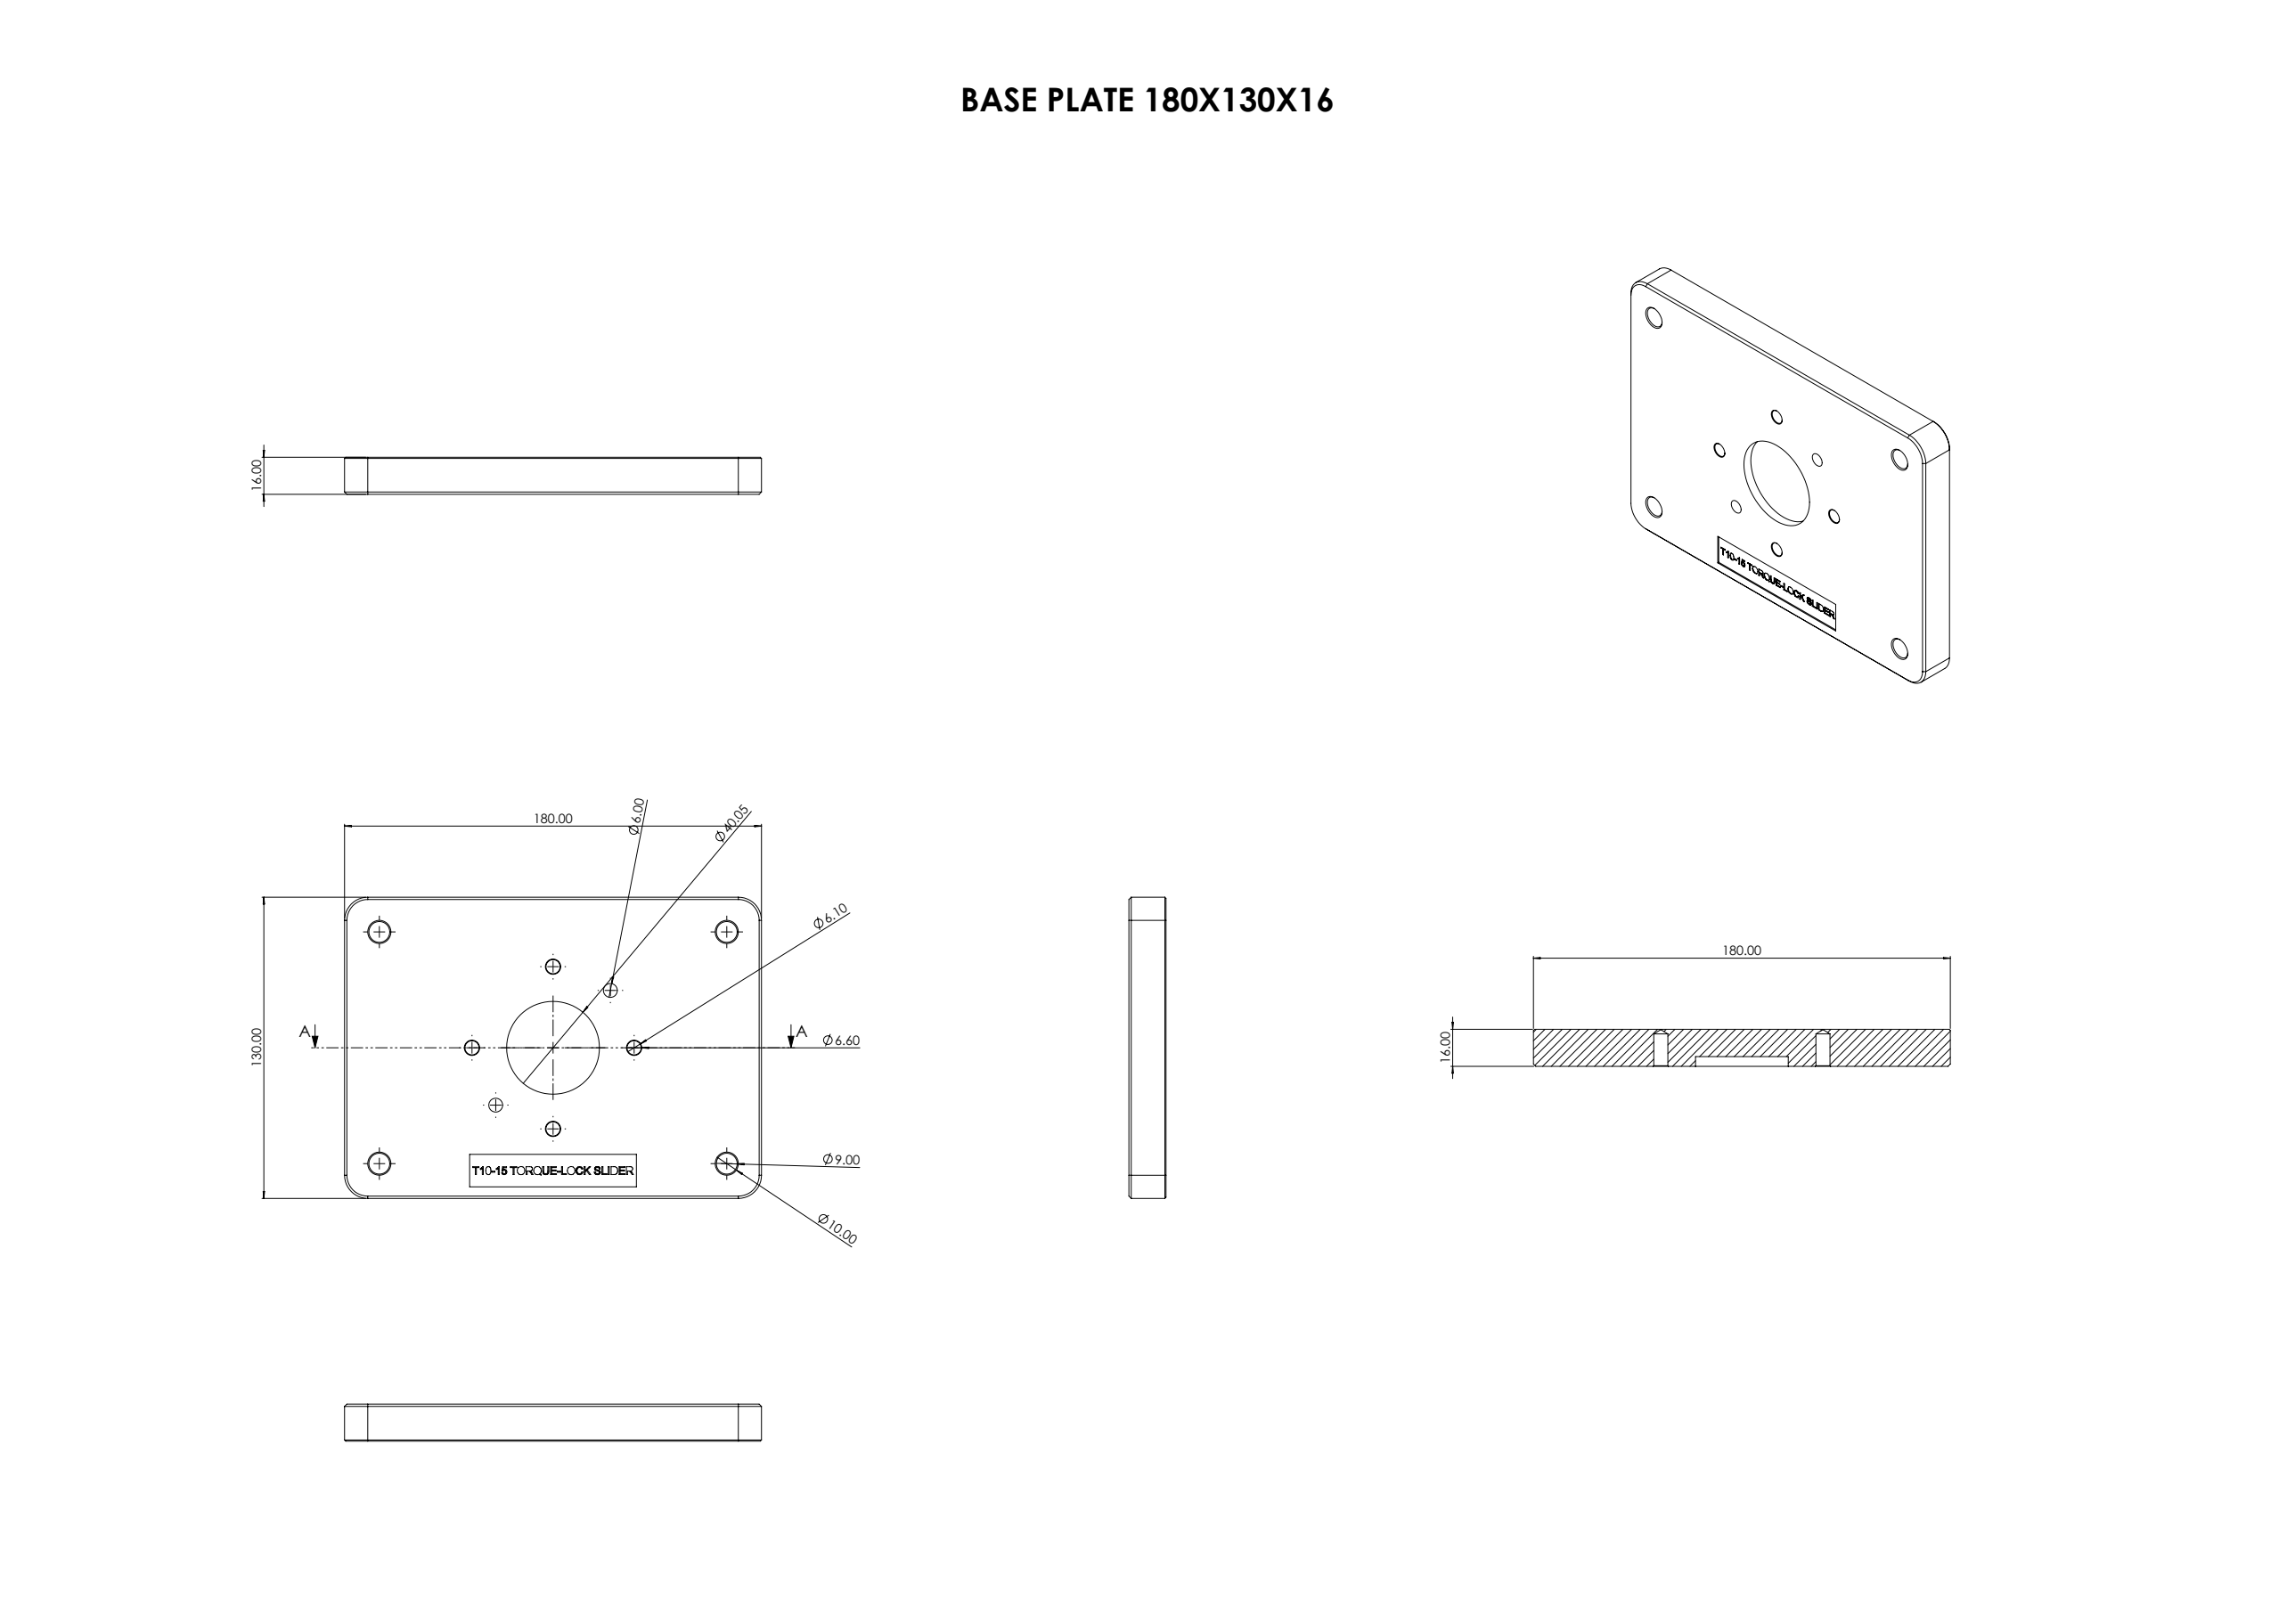
ISO-10303-21;
HEADER;
/* Generated by software containing ST-Developer
 * from STEP Tools, Inc. (www.steptools.com) 
 */

FILE_DESCRIPTION(
/* description */ (''),
/* implementation_level */ '2;1');

FILE_NAME(
/* name */ '04_Base_Plate_180x130x16.step',
/* time_stamp */ '2026-10-11T08:27:52-07:00',
/* author */ (''),
/* organization */ (''),
/* preprocessor_version */ 'ST-DEVELOPER v20.2',
/* originating_system */ 'Autodesk Translation Framework v15.15.0.0',
/* authorisation */ '');

FILE_SCHEMA (('AUTOMOTIVE_DESIGN { 1 0 10303 214 3 1 1 }'));
ENDSEC;

DATA;
#10=MECHANICAL_DESIGN_GEOMETRIC_PRESENTATION_REPRESENTATION('',(#922),#94301);
#147=B_SPLINE_CURVE_WITH_KNOTS('',2,(#80633,#80634,#80635),
 .UNSPECIFIED.,.F.,.F.,(3,3),(0.,1.),.UNSPECIFIED.);
#148=B_SPLINE_CURVE_WITH_KNOTS('',2,(#80639,#80640,#80641),
 .UNSPECIFIED.,.F.,.F.,(3,3),(0.,1.),.UNSPECIFIED.);
#149=B_SPLINE_CURVE_WITH_KNOTS('',2,(#80650,#80651,#80652),
 .UNSPECIFIED.,.F.,.F.,(3,3),(0.,1.),.UNSPECIFIED.);
#150=B_SPLINE_CURVE_WITH_KNOTS('',2,(#80655,#80656,#80657),
 .UNSPECIFIED.,.F.,.F.,(3,3),(0.,1.),.UNSPECIFIED.);
#151=B_SPLINE_CURVE_WITH_KNOTS('',2,(#80665,#80666,#80667),
 .UNSPECIFIED.,.F.,.F.,(3,3),(0.,1.),.UNSPECIFIED.);
#152=B_SPLINE_CURVE_WITH_KNOTS('',2,(#80670,#80671,#80672),
 .UNSPECIFIED.,.F.,.F.,(3,3),(0.,1.),.UNSPECIFIED.);
#153=B_SPLINE_CURVE_WITH_KNOTS('',2,(#80680,#80681,#80682),
 .UNSPECIFIED.,.F.,.F.,(3,3),(0.,1.),.UNSPECIFIED.);
#154=B_SPLINE_CURVE_WITH_KNOTS('',2,(#80685,#80686,#80687),
 .UNSPECIFIED.,.F.,.F.,(3,3),(0.,1.),.UNSPECIFIED.);
#155=B_SPLINE_CURVE_WITH_KNOTS('',2,(#80695,#80696,#80697),
 .UNSPECIFIED.,.F.,.F.,(3,3),(0.,1.),.UNSPECIFIED.);
#156=B_SPLINE_CURVE_WITH_KNOTS('',2,(#80700,#80701,#80702),
 .UNSPECIFIED.,.F.,.F.,(3,3),(0.,1.),.UNSPECIFIED.);
#157=B_SPLINE_CURVE_WITH_KNOTS('',2,(#80710,#80711,#80712),
 .UNSPECIFIED.,.F.,.F.,(3,3),(0.,1.),.UNSPECIFIED.);
#158=B_SPLINE_CURVE_WITH_KNOTS('',2,(#80715,#80716,#80717),
 .UNSPECIFIED.,.F.,.F.,(3,3),(0.,1.),.UNSPECIFIED.);
#159=B_SPLINE_CURVE_WITH_KNOTS('',2,(#80725,#80726,#80727),
 .UNSPECIFIED.,.F.,.F.,(3,3),(0.,1.),.UNSPECIFIED.);
#160=B_SPLINE_CURVE_WITH_KNOTS('',2,(#80730,#80731,#80732),
 .UNSPECIFIED.,.F.,.F.,(3,3),(0.,1.),.UNSPECIFIED.);
#161=B_SPLINE_CURVE_WITH_KNOTS('',2,(#80740,#80741,#80742),
 .UNSPECIFIED.,.F.,.F.,(3,3),(0.,1.),.UNSPECIFIED.);
#162=B_SPLINE_CURVE_WITH_KNOTS('',2,(#80745,#80746,#80747),
 .UNSPECIFIED.,.F.,.F.,(3,3),(0.,1.),.UNSPECIFIED.);
#163=B_SPLINE_CURVE_WITH_KNOTS('',2,(#80755,#80756,#80757),
 .UNSPECIFIED.,.F.,.F.,(3,3),(0.,1.),.UNSPECIFIED.);
#164=B_SPLINE_CURVE_WITH_KNOTS('',2,(#80760,#80761,#80762),
 .UNSPECIFIED.,.F.,.F.,(3,3),(0.,1.),.UNSPECIFIED.);
#165=B_SPLINE_CURVE_WITH_KNOTS('',2,(#80770,#80771,#80772),
 .UNSPECIFIED.,.F.,.F.,(3,3),(0.,1.),.UNSPECIFIED.);
#166=B_SPLINE_CURVE_WITH_KNOTS('',2,(#80775,#80776,#80777),
 .UNSPECIFIED.,.F.,.F.,(3,3),(0.,1.),.UNSPECIFIED.);
#167=B_SPLINE_CURVE_WITH_KNOTS('',2,(#80785,#80786,#80787),
 .UNSPECIFIED.,.F.,.F.,(3,3),(0.,1.),.UNSPECIFIED.);
#168=B_SPLINE_CURVE_WITH_KNOTS('',2,(#80790,#80791,#80792),
 .UNSPECIFIED.,.F.,.F.,(3,3),(0.,1.),.UNSPECIFIED.);
#169=B_SPLINE_CURVE_WITH_KNOTS('',2,(#80800,#80801,#80802),
 .UNSPECIFIED.,.F.,.F.,(3,3),(0.,1.),.UNSPECIFIED.);
#170=B_SPLINE_CURVE_WITH_KNOTS('',2,(#80805,#80806,#80807),
 .UNSPECIFIED.,.F.,.F.,(3,3),(0.,1.),.UNSPECIFIED.);
#171=B_SPLINE_CURVE_WITH_KNOTS('',2,(#80815,#80816,#80817),
 .UNSPECIFIED.,.F.,.F.,(3,3),(0.,1.),.UNSPECIFIED.);
#172=B_SPLINE_CURVE_WITH_KNOTS('',2,(#80820,#80821,#80822),
 .UNSPECIFIED.,.F.,.F.,(3,3),(0.,1.),.UNSPECIFIED.);
#173=B_SPLINE_CURVE_WITH_KNOTS('',2,(#80836,#80837,#80838),
 .UNSPECIFIED.,.F.,.F.,(3,3),(0.,1.),.UNSPECIFIED.);
#174=B_SPLINE_CURVE_WITH_KNOTS('',2,(#80841,#80842,#80843),
 .UNSPECIFIED.,.F.,.F.,(3,3),(0.,1.),.UNSPECIFIED.);
#175=B_SPLINE_CURVE_WITH_KNOTS('',2,(#80851,#80852,#80853),
 .UNSPECIFIED.,.F.,.F.,(3,3),(0.,1.),.UNSPECIFIED.);
#176=B_SPLINE_CURVE_WITH_KNOTS('',2,(#80856,#80857,#80858),
 .UNSPECIFIED.,.F.,.F.,(3,3),(0.,1.),.UNSPECIFIED.);
#177=B_SPLINE_CURVE_WITH_KNOTS('',2,(#80866,#80867,#80868),
 .UNSPECIFIED.,.F.,.F.,(3,3),(0.,1.),.UNSPECIFIED.);
#178=B_SPLINE_CURVE_WITH_KNOTS('',2,(#80871,#80872,#80873),
 .UNSPECIFIED.,.F.,.F.,(3,3),(0.,1.),.UNSPECIFIED.);
#179=B_SPLINE_CURVE_WITH_KNOTS('',2,(#80881,#80882,#80883),
 .UNSPECIFIED.,.F.,.F.,(3,3),(0.,1.),.UNSPECIFIED.);
#180=B_SPLINE_CURVE_WITH_KNOTS('',2,(#80886,#80887,#80888),
 .UNSPECIFIED.,.F.,.F.,(3,3),(0.,1.),.UNSPECIFIED.);
#181=B_SPLINE_CURVE_WITH_KNOTS('',2,(#80896,#80897,#80898),
 .UNSPECIFIED.,.F.,.F.,(3,3),(0.,1.),.UNSPECIFIED.);
#182=B_SPLINE_CURVE_WITH_KNOTS('',2,(#80901,#80902,#80903),
 .UNSPECIFIED.,.F.,.F.,(3,3),(0.,1.),.UNSPECIFIED.);
#183=B_SPLINE_CURVE_WITH_KNOTS('',2,(#80911,#80912,#80913),
 .UNSPECIFIED.,.F.,.F.,(3,3),(0.,1.),.UNSPECIFIED.);
#184=B_SPLINE_CURVE_WITH_KNOTS('',2,(#80916,#80917,#80918),
 .UNSPECIFIED.,.F.,.F.,(3,3),(0.,1.),.UNSPECIFIED.);
#185=B_SPLINE_CURVE_WITH_KNOTS('',2,(#80926,#80927,#80928),
 .UNSPECIFIED.,.F.,.F.,(3,3),(0.,1.),.UNSPECIFIED.);
#186=B_SPLINE_CURVE_WITH_KNOTS('',2,(#80931,#80932,#80933),
 .UNSPECIFIED.,.F.,.F.,(3,3),(0.,1.),.UNSPECIFIED.);
#187=B_SPLINE_CURVE_WITH_KNOTS('',2,(#80941,#80942,#80943),
 .UNSPECIFIED.,.F.,.F.,(3,3),(0.,1.),.UNSPECIFIED.);
#188=B_SPLINE_CURVE_WITH_KNOTS('',2,(#80946,#80947,#80948),
 .UNSPECIFIED.,.F.,.F.,(3,3),(0.,1.),.UNSPECIFIED.);
#189=B_SPLINE_CURVE_WITH_KNOTS('',2,(#80956,#80957,#80958),
 .UNSPECIFIED.,.F.,.F.,(3,3),(0.,1.),.UNSPECIFIED.);
#190=B_SPLINE_CURVE_WITH_KNOTS('',2,(#80961,#80962,#80963),
 .UNSPECIFIED.,.F.,.F.,(3,3),(0.,1.),.UNSPECIFIED.);
#191=B_SPLINE_CURVE_WITH_KNOTS('',2,(#80971,#80972,#80973),
 .UNSPECIFIED.,.F.,.F.,(3,3),(0.,1.),.UNSPECIFIED.);
#192=B_SPLINE_CURVE_WITH_KNOTS('',2,(#80976,#80977,#80978),
 .UNSPECIFIED.,.F.,.F.,(3,3),(0.,1.),.UNSPECIFIED.);
#193=B_SPLINE_CURVE_WITH_KNOTS('',2,(#80986,#80987,#80988),
 .UNSPECIFIED.,.F.,.F.,(3,3),(0.,1.),.UNSPECIFIED.);
#194=B_SPLINE_CURVE_WITH_KNOTS('',2,(#80991,#80992,#80993),
 .UNSPECIFIED.,.F.,.F.,(3,3),(0.,1.),.UNSPECIFIED.);
#195=B_SPLINE_CURVE_WITH_KNOTS('',2,(#81001,#81002,#81003),
 .UNSPECIFIED.,.F.,.F.,(3,3),(0.,1.),.UNSPECIFIED.);
#196=B_SPLINE_CURVE_WITH_KNOTS('',2,(#81006,#81007,#81008),
 .UNSPECIFIED.,.F.,.F.,(3,3),(0.,1.),.UNSPECIFIED.);
#197=B_SPLINE_CURVE_WITH_KNOTS('',2,(#81016,#81017,#81018),
 .UNSPECIFIED.,.F.,.F.,(3,3),(0.,1.),.UNSPECIFIED.);
#198=B_SPLINE_CURVE_WITH_KNOTS('',2,(#81021,#81022,#81023),
 .UNSPECIFIED.,.F.,.F.,(3,3),(0.,1.),.UNSPECIFIED.);
#199=B_SPLINE_CURVE_WITH_KNOTS('',2,(#81031,#81032,#81033),
 .UNSPECIFIED.,.F.,.F.,(3,3),(0.,1.),.UNSPECIFIED.);
#200=B_SPLINE_CURVE_WITH_KNOTS('',2,(#81036,#81037,#81038),
 .UNSPECIFIED.,.F.,.F.,(3,3),(0.,1.),.UNSPECIFIED.);
#201=B_SPLINE_CURVE_WITH_KNOTS('',2,(#81046,#81047,#81048),
 .UNSPECIFIED.,.F.,.F.,(3,3),(0.,1.),.UNSPECIFIED.);
#202=B_SPLINE_CURVE_WITH_KNOTS('',2,(#81051,#81052,#81053),
 .UNSPECIFIED.,.F.,.F.,(3,3),(0.,1.),.UNSPECIFIED.);
#203=B_SPLINE_CURVE_WITH_KNOTS('',2,(#81061,#81062,#81063),
 .UNSPECIFIED.,.F.,.F.,(3,3),(0.,1.),.UNSPECIFIED.);
#204=B_SPLINE_CURVE_WITH_KNOTS('',2,(#81066,#81067,#81068),
 .UNSPECIFIED.,.F.,.F.,(3,3),(0.,1.),.UNSPECIFIED.);
#205=B_SPLINE_CURVE_WITH_KNOTS('',2,(#81076,#81077,#81078),
 .UNSPECIFIED.,.F.,.F.,(3,3),(0.,1.),.UNSPECIFIED.);
#206=B_SPLINE_CURVE_WITH_KNOTS('',2,(#81081,#81082,#81083),
 .UNSPECIFIED.,.F.,.F.,(3,3),(0.,1.),.UNSPECIFIED.);
#207=B_SPLINE_CURVE_WITH_KNOTS('',2,(#81091,#81092,#81093),
 .UNSPECIFIED.,.F.,.F.,(3,3),(0.,1.),.UNSPECIFIED.);
#208=B_SPLINE_CURVE_WITH_KNOTS('',2,(#81096,#81097,#81098),
 .UNSPECIFIED.,.F.,.F.,(3,3),(0.,1.),.UNSPECIFIED.);
#209=B_SPLINE_CURVE_WITH_KNOTS('',2,(#81112,#81113,#81114),
 .UNSPECIFIED.,.F.,.F.,(3,3),(0.,1.),.UNSPECIFIED.);
#210=B_SPLINE_CURVE_WITH_KNOTS('',2,(#81117,#81118,#81119),
 .UNSPECIFIED.,.F.,.F.,(3,3),(0.,1.),.UNSPECIFIED.);
#211=B_SPLINE_CURVE_WITH_KNOTS('',2,(#81126,#81127,#81128),
 .UNSPECIFIED.,.F.,.F.,(3,3),(0.,1.),.UNSPECIFIED.);
#212=B_SPLINE_CURVE_WITH_KNOTS('',2,(#81129,#81130,#81131),
 .UNSPECIFIED.,.F.,.F.,(3,3),(0.,1.),.UNSPECIFIED.);
#213=B_SPLINE_CURVE_WITH_KNOTS('',2,(#81141,#81142,#81143),
 .UNSPECIFIED.,.F.,.F.,(3,3),(0.,1.),.UNSPECIFIED.);
#214=B_SPLINE_CURVE_WITH_KNOTS('',2,(#81147,#81148,#81149),
 .UNSPECIFIED.,.F.,.F.,(3,3),(0.,1.),.UNSPECIFIED.);
#215=B_SPLINE_CURVE_WITH_KNOTS('',2,(#81158,#81159,#81160),
 .UNSPECIFIED.,.F.,.F.,(3,3),(0.,1.),.UNSPECIFIED.);
#216=B_SPLINE_CURVE_WITH_KNOTS('',2,(#81163,#81164,#81165),
 .UNSPECIFIED.,.F.,.F.,(3,3),(0.,1.),.UNSPECIFIED.);
#217=B_SPLINE_CURVE_WITH_KNOTS('',2,(#81173,#81174,#81175),
 .UNSPECIFIED.,.F.,.F.,(3,3),(0.,1.),.UNSPECIFIED.);
#218=B_SPLINE_CURVE_WITH_KNOTS('',2,(#81178,#81179,#81180),
 .UNSPECIFIED.,.F.,.F.,(3,3),(0.,1.),.UNSPECIFIED.);
#219=B_SPLINE_CURVE_WITH_KNOTS('',2,(#81188,#81189,#81190),
 .UNSPECIFIED.,.F.,.F.,(3,3),(0.,1.),.UNSPECIFIED.);
#220=B_SPLINE_CURVE_WITH_KNOTS('',2,(#81193,#81194,#81195),
 .UNSPECIFIED.,.F.,.F.,(3,3),(0.,1.),.UNSPECIFIED.);
#221=B_SPLINE_CURVE_WITH_KNOTS('',2,(#81203,#81204,#81205),
 .UNSPECIFIED.,.F.,.F.,(3,3),(0.,1.),.UNSPECIFIED.);
#222=B_SPLINE_CURVE_WITH_KNOTS('',2,(#81208,#81209,#81210),
 .UNSPECIFIED.,.F.,.F.,(3,3),(0.,1.),.UNSPECIFIED.);
#223=B_SPLINE_CURVE_WITH_KNOTS('',2,(#81218,#81219,#81220),
 .UNSPECIFIED.,.F.,.F.,(3,3),(0.,1.),.UNSPECIFIED.);
#224=B_SPLINE_CURVE_WITH_KNOTS('',2,(#81223,#81224,#81225),
 .UNSPECIFIED.,.F.,.F.,(3,3),(0.,1.),.UNSPECIFIED.);
#225=B_SPLINE_CURVE_WITH_KNOTS('',2,(#81233,#81234,#81235),
 .UNSPECIFIED.,.F.,.F.,(3,3),(0.,1.),.UNSPECIFIED.);
#226=B_SPLINE_CURVE_WITH_KNOTS('',2,(#81238,#81239,#81240),
 .UNSPECIFIED.,.F.,.F.,(3,3),(0.,1.),.UNSPECIFIED.);
#227=B_SPLINE_CURVE_WITH_KNOTS('',2,(#81248,#81249,#81250),
 .UNSPECIFIED.,.F.,.F.,(3,3),(0.,1.),.UNSPECIFIED.);
#228=B_SPLINE_CURVE_WITH_KNOTS('',2,(#81253,#81254,#81255),
 .UNSPECIFIED.,.F.,.F.,(3,3),(0.,1.),.UNSPECIFIED.);
#229=B_SPLINE_CURVE_WITH_KNOTS('',2,(#81269,#81270,#81271),
 .UNSPECIFIED.,.F.,.F.,(3,3),(0.,1.),.UNSPECIFIED.);
#230=B_SPLINE_CURVE_WITH_KNOTS('',2,(#81274,#81275,#81276),
 .UNSPECIFIED.,.F.,.F.,(3,3),(0.,1.),.UNSPECIFIED.);
#231=B_SPLINE_CURVE_WITH_KNOTS('',2,(#81284,#81285,#81286),
 .UNSPECIFIED.,.F.,.F.,(3,3),(0.,1.),.UNSPECIFIED.);
#232=B_SPLINE_CURVE_WITH_KNOTS('',2,(#81289,#81290,#81291),
 .UNSPECIFIED.,.F.,.F.,(3,3),(0.,1.),.UNSPECIFIED.);
#233=B_SPLINE_CURVE_WITH_KNOTS('',2,(#81299,#81300,#81301),
 .UNSPECIFIED.,.F.,.F.,(3,3),(0.,1.),.UNSPECIFIED.);
#234=B_SPLINE_CURVE_WITH_KNOTS('',2,(#81304,#81305,#81306),
 .UNSPECIFIED.,.F.,.F.,(3,3),(0.,1.),.UNSPECIFIED.);
#235=B_SPLINE_CURVE_WITH_KNOTS('',2,(#81314,#81315,#81316),
 .UNSPECIFIED.,.F.,.F.,(3,3),(0.,1.),.UNSPECIFIED.);
#236=B_SPLINE_CURVE_WITH_KNOTS('',2,(#81319,#81320,#81321),
 .UNSPECIFIED.,.F.,.F.,(3,3),(0.,1.),.UNSPECIFIED.);
#237=B_SPLINE_CURVE_WITH_KNOTS('',2,(#81329,#81330,#81331),
 .UNSPECIFIED.,.F.,.F.,(3,3),(0.,1.),.UNSPECIFIED.);
#238=B_SPLINE_CURVE_WITH_KNOTS('',2,(#81334,#81335,#81336),
 .UNSPECIFIED.,.F.,.F.,(3,3),(0.,1.),.UNSPECIFIED.);
#239=B_SPLINE_CURVE_WITH_KNOTS('',2,(#81344,#81345,#81346),
 .UNSPECIFIED.,.F.,.F.,(3,3),(0.,1.),.UNSPECIFIED.);
#240=B_SPLINE_CURVE_WITH_KNOTS('',2,(#81349,#81350,#81351),
 .UNSPECIFIED.,.F.,.F.,(3,3),(0.,1.),.UNSPECIFIED.);
#241=B_SPLINE_CURVE_WITH_KNOTS('',2,(#81359,#81360,#81361),
 .UNSPECIFIED.,.F.,.F.,(3,3),(0.,1.),.UNSPECIFIED.);
#242=B_SPLINE_CURVE_WITH_KNOTS('',2,(#81364,#81365,#81366),
 .UNSPECIFIED.,.F.,.F.,(3,3),(0.,1.),.UNSPECIFIED.);
#243=B_SPLINE_CURVE_WITH_KNOTS('',2,(#81374,#81375,#81376),
 .UNSPECIFIED.,.F.,.F.,(3,3),(0.,1.),.UNSPECIFIED.);
#244=B_SPLINE_CURVE_WITH_KNOTS('',2,(#81379,#81380,#81381),
 .UNSPECIFIED.,.F.,.F.,(3,3),(0.,1.),.UNSPECIFIED.);
#245=B_SPLINE_CURVE_WITH_KNOTS('',2,(#81389,#81390,#81391),
 .UNSPECIFIED.,.F.,.F.,(3,3),(0.,1.),.UNSPECIFIED.);
#246=B_SPLINE_CURVE_WITH_KNOTS('',2,(#81394,#81395,#81396),
 .UNSPECIFIED.,.F.,.F.,(3,3),(0.,1.),.UNSPECIFIED.);
#247=B_SPLINE_CURVE_WITH_KNOTS('',2,(#81404,#81405,#81406),
 .UNSPECIFIED.,.F.,.F.,(3,3),(0.,1.),.UNSPECIFIED.);
#248=B_SPLINE_CURVE_WITH_KNOTS('',2,(#81409,#81410,#81411),
 .UNSPECIFIED.,.F.,.F.,(3,3),(0.,1.),.UNSPECIFIED.);
#249=B_SPLINE_CURVE_WITH_KNOTS('',2,(#81425,#81426,#81427),
 .UNSPECIFIED.,.F.,.F.,(3,3),(0.,1.),.UNSPECIFIED.);
#250=B_SPLINE_CURVE_WITH_KNOTS('',2,(#81430,#81431,#81432),
 .UNSPECIFIED.,.F.,.F.,(3,3),(0.,1.),.UNSPECIFIED.);
#251=B_SPLINE_CURVE_WITH_KNOTS('',2,(#81439,#81440,#81441),
 .UNSPECIFIED.,.F.,.F.,(3,3),(0.,1.),.UNSPECIFIED.);
#252=B_SPLINE_CURVE_WITH_KNOTS('',2,(#81442,#81443,#81444),
 .UNSPECIFIED.,.F.,.F.,(3,3),(0.,1.),.UNSPECIFIED.);
#253=B_SPLINE_CURVE_WITH_KNOTS('',2,(#81540,#81541,#81542),
 .UNSPECIFIED.,.F.,.F.,(3,3),(0.,1.),.UNSPECIFIED.);
#254=B_SPLINE_CURVE_WITH_KNOTS('',2,(#81546,#81547,#81548),
 .UNSPECIFIED.,.F.,.F.,(3,3),(0.,1.),.UNSPECIFIED.);
#255=B_SPLINE_CURVE_WITH_KNOTS('',2,(#81557,#81558,#81559),
 .UNSPECIFIED.,.F.,.F.,(3,3),(0.,1.),.UNSPECIFIED.);
#256=B_SPLINE_CURVE_WITH_KNOTS('',2,(#81562,#81563,#81564),
 .UNSPECIFIED.,.F.,.F.,(3,3),(0.,1.),.UNSPECIFIED.);
#257=B_SPLINE_CURVE_WITH_KNOTS('',2,(#81572,#81573,#81574),
 .UNSPECIFIED.,.F.,.F.,(3,3),(0.,1.),.UNSPECIFIED.);
#258=B_SPLINE_CURVE_WITH_KNOTS('',2,(#81577,#81578,#81579),
 .UNSPECIFIED.,.F.,.F.,(3,3),(0.,1.),.UNSPECIFIED.);
#259=B_SPLINE_CURVE_WITH_KNOTS('',2,(#81587,#81588,#81589),
 .UNSPECIFIED.,.F.,.F.,(3,3),(0.,1.),.UNSPECIFIED.);
#260=B_SPLINE_CURVE_WITH_KNOTS('',2,(#81592,#81593,#81594),
 .UNSPECIFIED.,.F.,.F.,(3,3),(0.,1.),.UNSPECIFIED.);
#261=B_SPLINE_CURVE_WITH_KNOTS('',2,(#81620,#81621,#81622),
 .UNSPECIFIED.,.F.,.F.,(3,3),(0.,1.),.UNSPECIFIED.);
#262=B_SPLINE_CURVE_WITH_KNOTS('',2,(#81625,#81626,#81627),
 .UNSPECIFIED.,.F.,.F.,(3,3),(0.,1.),.UNSPECIFIED.);
#263=B_SPLINE_CURVE_WITH_KNOTS('',2,(#81635,#81636,#81637),
 .UNSPECIFIED.,.F.,.F.,(3,3),(0.,1.),.UNSPECIFIED.);
#264=B_SPLINE_CURVE_WITH_KNOTS('',2,(#81640,#81641,#81642),
 .UNSPECIFIED.,.F.,.F.,(3,3),(0.,1.),.UNSPECIFIED.);
#265=B_SPLINE_CURVE_WITH_KNOTS('',2,(#81650,#81651,#81652),
 .UNSPECIFIED.,.F.,.F.,(3,3),(0.,1.),.UNSPECIFIED.);
#266=B_SPLINE_CURVE_WITH_KNOTS('',2,(#81655,#81656,#81657),
 .UNSPECIFIED.,.F.,.F.,(3,3),(0.,1.),.UNSPECIFIED.);
#267=B_SPLINE_CURVE_WITH_KNOTS('',2,(#81665,#81666,#81667),
 .UNSPECIFIED.,.F.,.F.,(3,3),(0.,1.),.UNSPECIFIED.);
#268=B_SPLINE_CURVE_WITH_KNOTS('',2,(#81670,#81671,#81672),
 .UNSPECIFIED.,.F.,.F.,(3,3),(0.,1.),.UNSPECIFIED.);
#269=B_SPLINE_CURVE_WITH_KNOTS('',2,(#81680,#81681,#81682),
 .UNSPECIFIED.,.F.,.F.,(3,3),(0.,1.),.UNSPECIFIED.);
#270=B_SPLINE_CURVE_WITH_KNOTS('',2,(#81685,#81686,#81687),
 .UNSPECIFIED.,.F.,.F.,(3,3),(0.,1.),.UNSPECIFIED.);
#271=B_SPLINE_CURVE_WITH_KNOTS('',2,(#81695,#81696,#81697),
 .UNSPECIFIED.,.F.,.F.,(3,3),(0.,1.),.UNSPECIFIED.);
#272=B_SPLINE_CURVE_WITH_KNOTS('',2,(#81700,#81701,#81702),
 .UNSPECIFIED.,.F.,.F.,(3,3),(0.,1.),.UNSPECIFIED.);
#273=B_SPLINE_CURVE_WITH_KNOTS('',2,(#81727,#81728,#81729),
 .UNSPECIFIED.,.F.,.F.,(3,3),(0.,1.),.UNSPECIFIED.);
#274=B_SPLINE_CURVE_WITH_KNOTS('',2,(#81730,#81731,#81732),
 .UNSPECIFIED.,.F.,.F.,(3,3),(0.,1.),.UNSPECIFIED.);
#275=B_SPLINE_CURVE_WITH_KNOTS('',2,(#81750,#81751,#81752),
 .UNSPECIFIED.,.F.,.F.,(3,3),(0.,1.),.UNSPECIFIED.);
#276=B_SPLINE_CURVE_WITH_KNOTS('',2,(#81755,#81756,#81757),
 .UNSPECIFIED.,.F.,.F.,(3,3),(0.,1.),.UNSPECIFIED.);
#277=B_SPLINE_CURVE_WITH_KNOTS('',2,(#81765,#81766,#81767),
 .UNSPECIFIED.,.F.,.F.,(3,3),(0.,1.),.UNSPECIFIED.);
#278=B_SPLINE_CURVE_WITH_KNOTS('',2,(#81770,#81771,#81772),
 .UNSPECIFIED.,.F.,.F.,(3,3),(0.,1.),.UNSPECIFIED.);
#279=B_SPLINE_CURVE_WITH_KNOTS('',2,(#81780,#81781,#81782),
 .UNSPECIFIED.,.F.,.F.,(3,3),(0.,1.),.UNSPECIFIED.);
#280=B_SPLINE_CURVE_WITH_KNOTS('',2,(#81785,#81786,#81787),
 .UNSPECIFIED.,.F.,.F.,(3,3),(0.,1.),.UNSPECIFIED.);
#281=B_SPLINE_CURVE_WITH_KNOTS('',2,(#81795,#81796,#81797),
 .UNSPECIFIED.,.F.,.F.,(3,3),(0.,1.),.UNSPECIFIED.);
#282=B_SPLINE_CURVE_WITH_KNOTS('',2,(#81800,#81801,#81802),
 .UNSPECIFIED.,.F.,.F.,(3,3),(0.,1.),.UNSPECIFIED.);
#283=B_SPLINE_CURVE_WITH_KNOTS('',2,(#81828,#81829,#81830),
 .UNSPECIFIED.,.F.,.F.,(3,3),(0.,1.),.UNSPECIFIED.);
#284=B_SPLINE_CURVE_WITH_KNOTS('',2,(#81833,#81834,#81835),
 .UNSPECIFIED.,.F.,.F.,(3,3),(0.,1.),.UNSPECIFIED.);
#285=B_SPLINE_CURVE_WITH_KNOTS('',2,(#81843,#81844,#81845),
 .UNSPECIFIED.,.F.,.F.,(3,3),(0.,1.),.UNSPECIFIED.);
#286=B_SPLINE_CURVE_WITH_KNOTS('',2,(#81848,#81849,#81850),
 .UNSPECIFIED.,.F.,.F.,(3,3),(0.,1.),.UNSPECIFIED.);
#287=B_SPLINE_CURVE_WITH_KNOTS('',2,(#81858,#81859,#81860),
 .UNSPECIFIED.,.F.,.F.,(3,3),(0.,1.),.UNSPECIFIED.);
#288=B_SPLINE_CURVE_WITH_KNOTS('',2,(#81863,#81864,#81865),
 .UNSPECIFIED.,.F.,.F.,(3,3),(0.,1.),.UNSPECIFIED.);
#289=B_SPLINE_CURVE_WITH_KNOTS('',2,(#81873,#81874,#81875),
 .UNSPECIFIED.,.F.,.F.,(3,3),(0.,1.),.UNSPECIFIED.);
#290=B_SPLINE_CURVE_WITH_KNOTS('',2,(#81878,#81879,#81880),
 .UNSPECIFIED.,.F.,.F.,(3,3),(0.,1.),.UNSPECIFIED.);
#291=B_SPLINE_CURVE_WITH_KNOTS('',2,(#81888,#81889,#81890),
 .UNSPECIFIED.,.F.,.F.,(3,3),(0.,1.),.UNSPECIFIED.);
#292=B_SPLINE_CURVE_WITH_KNOTS('',2,(#81893,#81894,#81895),
 .UNSPECIFIED.,.F.,.F.,(3,3),(0.,1.),.UNSPECIFIED.);
#293=B_SPLINE_CURVE_WITH_KNOTS('',2,(#81903,#81904,#81905),
 .UNSPECIFIED.,.F.,.F.,(3,3),(0.,1.),.UNSPECIFIED.);
#294=B_SPLINE_CURVE_WITH_KNOTS('',2,(#81908,#81909,#81910),
 .UNSPECIFIED.,.F.,.F.,(3,3),(0.,1.),.UNSPECIFIED.);
#295=B_SPLINE_CURVE_WITH_KNOTS('',2,(#81918,#81919,#81920),
 .UNSPECIFIED.,.F.,.F.,(3,3),(0.,1.),.UNSPECIFIED.);
#296=B_SPLINE_CURVE_WITH_KNOTS('',2,(#81923,#81924,#81925),
 .UNSPECIFIED.,.F.,.F.,(3,3),(0.,1.),.UNSPECIFIED.);
#297=B_SPLINE_CURVE_WITH_KNOTS('',2,(#82005,#82006,#82007),
 .UNSPECIFIED.,.F.,.F.,(3,3),(0.,1.),.UNSPECIFIED.);
#298=B_SPLINE_CURVE_WITH_KNOTS('',2,(#82011,#82012,#82013),
 .UNSPECIFIED.,.F.,.F.,(3,3),(0.,1.),.UNSPECIFIED.);
#299=B_SPLINE_CURVE_WITH_KNOTS('',2,(#82022,#82023,#82024),
 .UNSPECIFIED.,.F.,.F.,(3,3),(0.,1.),.UNSPECIFIED.);
#300=B_SPLINE_CURVE_WITH_KNOTS('',2,(#82027,#82028,#82029),
 .UNSPECIFIED.,.F.,.F.,(3,3),(0.,1.),.UNSPECIFIED.);
#301=B_SPLINE_CURVE_WITH_KNOTS('',2,(#82043,#82044,#82045),
 .UNSPECIFIED.,.F.,.F.,(3,3),(0.,1.),.UNSPECIFIED.);
#302=B_SPLINE_CURVE_WITH_KNOTS('',2,(#82048,#82049,#82050),
 .UNSPECIFIED.,.F.,.F.,(3,3),(0.,1.),.UNSPECIFIED.);
#303=B_SPLINE_CURVE_WITH_KNOTS('',2,(#82058,#82059,#82060),
 .UNSPECIFIED.,.F.,.F.,(3,3),(0.,1.),.UNSPECIFIED.);
#304=B_SPLINE_CURVE_WITH_KNOTS('',2,(#82063,#82064,#82065),
 .UNSPECIFIED.,.F.,.F.,(3,3),(0.,1.),.UNSPECIFIED.);
#305=B_SPLINE_CURVE_WITH_KNOTS('',2,(#82096,#82097,#82098),
 .UNSPECIFIED.,.F.,.F.,(3,3),(0.,1.),.UNSPECIFIED.);
#306=B_SPLINE_CURVE_WITH_KNOTS('',2,(#82102,#82103,#82104),
 .UNSPECIFIED.,.F.,.F.,(3,3),(0.,1.),.UNSPECIFIED.);
#307=B_SPLINE_CURVE_WITH_KNOTS('',2,(#82113,#82114,#82115),
 .UNSPECIFIED.,.F.,.F.,(3,3),(0.,1.),.UNSPECIFIED.);
#308=B_SPLINE_CURVE_WITH_KNOTS('',2,(#82118,#82119,#82120),
 .UNSPECIFIED.,.F.,.F.,(3,3),(0.,1.),.UNSPECIFIED.);
#309=B_SPLINE_CURVE_WITH_KNOTS('',2,(#82128,#82129,#82130),
 .UNSPECIFIED.,.F.,.F.,(3,3),(0.,1.),.UNSPECIFIED.);
#310=B_SPLINE_CURVE_WITH_KNOTS('',2,(#82133,#82134,#82135),
 .UNSPECIFIED.,.F.,.F.,(3,3),(0.,1.),.UNSPECIFIED.);
#311=B_SPLINE_CURVE_WITH_KNOTS('',2,(#82143,#82144,#82145),
 .UNSPECIFIED.,.F.,.F.,(3,3),(0.,1.),.UNSPECIFIED.);
#312=B_SPLINE_CURVE_WITH_KNOTS('',2,(#82148,#82149,#82150),
 .UNSPECIFIED.,.F.,.F.,(3,3),(0.,1.),.UNSPECIFIED.);
#313=B_SPLINE_CURVE_WITH_KNOTS('',2,(#82158,#82159,#82160),
 .UNSPECIFIED.,.F.,.F.,(3,3),(0.,1.),.UNSPECIFIED.);
#314=B_SPLINE_CURVE_WITH_KNOTS('',2,(#82163,#82164,#82165),
 .UNSPECIFIED.,.F.,.F.,(3,3),(0.,1.),.UNSPECIFIED.);
#315=B_SPLINE_CURVE_WITH_KNOTS('',2,(#82173,#82174,#82175),
 .UNSPECIFIED.,.F.,.F.,(3,3),(0.,1.),.UNSPECIFIED.);
#316=B_SPLINE_CURVE_WITH_KNOTS('',2,(#82178,#82179,#82180),
 .UNSPECIFIED.,.F.,.F.,(3,3),(0.,1.),.UNSPECIFIED.);
#317=B_SPLINE_CURVE_WITH_KNOTS('',2,(#82188,#82189,#82190),
 .UNSPECIFIED.,.F.,.F.,(3,3),(0.,1.),.UNSPECIFIED.);
#318=B_SPLINE_CURVE_WITH_KNOTS('',2,(#82193,#82194,#82195),
 .UNSPECIFIED.,.F.,.F.,(3,3),(0.,1.),.UNSPECIFIED.);
#319=B_SPLINE_CURVE_WITH_KNOTS('',2,(#82203,#82204,#82205),
 .UNSPECIFIED.,.F.,.F.,(3,3),(0.,1.),.UNSPECIFIED.);
#320=B_SPLINE_CURVE_WITH_KNOTS('',2,(#82208,#82209,#82210),
 .UNSPECIFIED.,.F.,.F.,(3,3),(0.,1.),.UNSPECIFIED.);
#321=B_SPLINE_CURVE_WITH_KNOTS('',2,(#82218,#82219,#82220),
 .UNSPECIFIED.,.F.,.F.,(3,3),(0.,1.),.UNSPECIFIED.);
#322=B_SPLINE_CURVE_WITH_KNOTS('',2,(#82223,#82224,#82225),
 .UNSPECIFIED.,.F.,.F.,(3,3),(0.,1.),.UNSPECIFIED.);
#323=B_SPLINE_CURVE_WITH_KNOTS('',2,(#82233,#82234,#82235),
 .UNSPECIFIED.,.F.,.F.,(3,3),(0.,1.),.UNSPECIFIED.);
#324=B_SPLINE_CURVE_WITH_KNOTS('',2,(#82238,#82239,#82240),
 .UNSPECIFIED.,.F.,.F.,(3,3),(0.,1.),.UNSPECIFIED.);
#325=B_SPLINE_CURVE_WITH_KNOTS('',2,(#82248,#82249,#82250),
 .UNSPECIFIED.,.F.,.F.,(3,3),(0.,1.),.UNSPECIFIED.);
#326=B_SPLINE_CURVE_WITH_KNOTS('',2,(#82253,#82254,#82255),
 .UNSPECIFIED.,.F.,.F.,(3,3),(0.,1.),.UNSPECIFIED.);
#327=B_SPLINE_CURVE_WITH_KNOTS('',2,(#82262,#82263,#82264),
 .UNSPECIFIED.,.F.,.F.,(3,3),(0.,1.),.UNSPECIFIED.);
#328=B_SPLINE_CURVE_WITH_KNOTS('',2,(#82265,#82266,#82267),
 .UNSPECIFIED.,.F.,.F.,(3,3),(0.,1.),.UNSPECIFIED.);
#329=B_SPLINE_CURVE_WITH_KNOTS('',2,(#82277,#82278,#82279),
 .UNSPECIFIED.,.F.,.F.,(3,3),(0.,1.),.UNSPECIFIED.);
#330=B_SPLINE_CURVE_WITH_KNOTS('',2,(#82283,#82284,#82285),
 .UNSPECIFIED.,.F.,.F.,(3,3),(0.,1.),.UNSPECIFIED.);
#331=B_SPLINE_CURVE_WITH_KNOTS('',2,(#82294,#82295,#82296),
 .UNSPECIFIED.,.F.,.F.,(3,3),(0.,1.),.UNSPECIFIED.);
#332=B_SPLINE_CURVE_WITH_KNOTS('',2,(#82299,#82300,#82301),
 .UNSPECIFIED.,.F.,.F.,(3,3),(0.,1.),.UNSPECIFIED.);
#333=B_SPLINE_CURVE_WITH_KNOTS('',2,(#82315,#82316,#82317),
 .UNSPECIFIED.,.F.,.F.,(3,3),(0.,1.),.UNSPECIFIED.);
#334=B_SPLINE_CURVE_WITH_KNOTS('',2,(#82320,#82321,#82322),
 .UNSPECIFIED.,.F.,.F.,(3,3),(0.,1.),.UNSPECIFIED.);
#335=B_SPLINE_CURVE_WITH_KNOTS('',2,(#82330,#82331,#82332),
 .UNSPECIFIED.,.F.,.F.,(3,3),(0.,1.),.UNSPECIFIED.);
#336=B_SPLINE_CURVE_WITH_KNOTS('',2,(#82335,#82336,#82337),
 .UNSPECIFIED.,.F.,.F.,(3,3),(0.,1.),.UNSPECIFIED.);
#337=B_SPLINE_CURVE_WITH_KNOTS('',2,(#82393,#82394,#82395),
 .UNSPECIFIED.,.F.,.F.,(3,3),(0.,1.),.UNSPECIFIED.);
#338=B_SPLINE_CURVE_WITH_KNOTS('',2,(#82399,#82400,#82401),
 .UNSPECIFIED.,.F.,.F.,(3,3),(0.,1.),.UNSPECIFIED.);
#339=B_SPLINE_CURVE_WITH_KNOTS('',2,(#82410,#82411,#82412),
 .UNSPECIFIED.,.F.,.F.,(3,3),(0.,1.),.UNSPECIFIED.);
#340=B_SPLINE_CURVE_WITH_KNOTS('',2,(#82415,#82416,#82417),
 .UNSPECIFIED.,.F.,.F.,(3,3),(0.,1.),.UNSPECIFIED.);
#341=B_SPLINE_CURVE_WITH_KNOTS('',2,(#82425,#82426,#82427),
 .UNSPECIFIED.,.F.,.F.,(3,3),(0.,1.),.UNSPECIFIED.);
#342=B_SPLINE_CURVE_WITH_KNOTS('',2,(#82430,#82431,#82432),
 .UNSPECIFIED.,.F.,.F.,(3,3),(0.,1.),.UNSPECIFIED.);
#343=B_SPLINE_CURVE_WITH_KNOTS('',2,(#82440,#82441,#82442),
 .UNSPECIFIED.,.F.,.F.,(3,3),(0.,1.),.UNSPECIFIED.);
#344=B_SPLINE_CURVE_WITH_KNOTS('',2,(#82445,#82446,#82447),
 .UNSPECIFIED.,.F.,.F.,(3,3),(0.,1.),.UNSPECIFIED.);
#345=B_SPLINE_CURVE_WITH_KNOTS('',2,(#82455,#82456,#82457),
 .UNSPECIFIED.,.F.,.F.,(3,3),(0.,1.),.UNSPECIFIED.);
#346=B_SPLINE_CURVE_WITH_KNOTS('',2,(#82460,#82461,#82462),
 .UNSPECIFIED.,.F.,.F.,(3,3),(0.,1.),.UNSPECIFIED.);
#347=B_SPLINE_CURVE_WITH_KNOTS('',2,(#82506,#82507,#82508),
 .UNSPECIFIED.,.F.,.F.,(3,3),(0.,1.),.UNSPECIFIED.);
#348=B_SPLINE_CURVE_WITH_KNOTS('',2,(#82511,#82512,#82513),
 .UNSPECIFIED.,.F.,.F.,(3,3),(0.,1.),.UNSPECIFIED.);
#349=B_SPLINE_CURVE_WITH_KNOTS('',2,(#82521,#82522,#82523),
 .UNSPECIFIED.,.F.,.F.,(3,3),(0.,1.),.UNSPECIFIED.);
#350=B_SPLINE_CURVE_WITH_KNOTS('',2,(#82526,#82527,#82528),
 .UNSPECIFIED.,.F.,.F.,(3,3),(0.,1.),.UNSPECIFIED.);
#351=B_SPLINE_CURVE_WITH_KNOTS('',2,(#82536,#82537,#82538),
 .UNSPECIFIED.,.F.,.F.,(3,3),(0.,1.),.UNSPECIFIED.);
#352=B_SPLINE_CURVE_WITH_KNOTS('',2,(#82541,#82542,#82543),
 .UNSPECIFIED.,.F.,.F.,(3,3),(0.,1.),.UNSPECIFIED.);
#353=B_SPLINE_CURVE_WITH_KNOTS('',2,(#82551,#82552,#82553),
 .UNSPECIFIED.,.F.,.F.,(3,3),(0.,1.),.UNSPECIFIED.);
#354=B_SPLINE_CURVE_WITH_KNOTS('',2,(#82556,#82557,#82558),
 .UNSPECIFIED.,.F.,.F.,(3,3),(0.,1.),.UNSPECIFIED.);
#355=B_SPLINE_CURVE_WITH_KNOTS('',2,(#82566,#82567,#82568),
 .UNSPECIFIED.,.F.,.F.,(3,3),(0.,1.),.UNSPECIFIED.);
#356=B_SPLINE_CURVE_WITH_KNOTS('',2,(#82571,#82572,#82573),
 .UNSPECIFIED.,.F.,.F.,(3,3),(0.,1.),.UNSPECIFIED.);
#357=B_SPLINE_CURVE_WITH_KNOTS('',2,(#82581,#82582,#82583),
 .UNSPECIFIED.,.F.,.F.,(3,3),(0.,1.),.UNSPECIFIED.);
#358=B_SPLINE_CURVE_WITH_KNOTS('',2,(#82586,#82587,#82588),
 .UNSPECIFIED.,.F.,.F.,(3,3),(0.,1.),.UNSPECIFIED.);
#359=B_SPLINE_CURVE_WITH_KNOTS('',2,(#82596,#82597,#82598),
 .UNSPECIFIED.,.F.,.F.,(3,3),(0.,1.),.UNSPECIFIED.);
#360=B_SPLINE_CURVE_WITH_KNOTS('',2,(#82601,#82602,#82603),
 .UNSPECIFIED.,.F.,.F.,(3,3),(0.,1.),.UNSPECIFIED.);
#361=B_SPLINE_CURVE_WITH_KNOTS('',2,(#82611,#82612,#82613),
 .UNSPECIFIED.,.F.,.F.,(3,3),(0.,1.),.UNSPECIFIED.);
#362=B_SPLINE_CURVE_WITH_KNOTS('',2,(#82616,#82617,#82618),
 .UNSPECIFIED.,.F.,.F.,(3,3),(0.,1.),.UNSPECIFIED.);
#363=B_SPLINE_CURVE_WITH_KNOTS('',2,(#82632,#82633,#82634),
 .UNSPECIFIED.,.F.,.F.,(3,3),(0.,1.),.UNSPECIFIED.);
#364=B_SPLINE_CURVE_WITH_KNOTS('',2,(#82637,#82638,#82639),
 .UNSPECIFIED.,.F.,.F.,(3,3),(0.,1.),.UNSPECIFIED.);
#365=B_SPLINE_CURVE_WITH_KNOTS('',2,(#82646,#82647,#82648),
 .UNSPECIFIED.,.F.,.F.,(3,3),(0.,1.),.UNSPECIFIED.);
#366=B_SPLINE_CURVE_WITH_KNOTS('',2,(#82649,#82650,#82651),
 .UNSPECIFIED.,.F.,.F.,(3,3),(0.,1.),.UNSPECIFIED.);
#367=B_SPLINE_CURVE_WITH_KNOTS('',2,(#82661,#82662,#82663),
 .UNSPECIFIED.,.F.,.F.,(3,3),(0.,1.),.UNSPECIFIED.);
#368=B_SPLINE_CURVE_WITH_KNOTS('',2,(#82667,#82668,#82669),
 .UNSPECIFIED.,.F.,.F.,(3,3),(0.,1.),.UNSPECIFIED.);
#369=B_SPLINE_CURVE_WITH_KNOTS('',2,(#82678,#82679,#82680),
 .UNSPECIFIED.,.F.,.F.,(3,3),(0.,1.),.UNSPECIFIED.);
#370=B_SPLINE_CURVE_WITH_KNOTS('',2,(#82683,#82684,#82685),
 .UNSPECIFIED.,.F.,.F.,(3,3),(0.,1.),.UNSPECIFIED.);
#371=B_SPLINE_CURVE_WITH_KNOTS('',2,(#82693,#82694,#82695),
 .UNSPECIFIED.,.F.,.F.,(3,3),(0.,1.),.UNSPECIFIED.);
#372=B_SPLINE_CURVE_WITH_KNOTS('',2,(#82698,#82699,#82700),
 .UNSPECIFIED.,.F.,.F.,(3,3),(0.,1.),.UNSPECIFIED.);
#373=B_SPLINE_CURVE_WITH_KNOTS('',2,(#82708,#82709,#82710),
 .UNSPECIFIED.,.F.,.F.,(3,3),(0.,1.),.UNSPECIFIED.);
#374=B_SPLINE_CURVE_WITH_KNOTS('',2,(#82713,#82714,#82715),
 .UNSPECIFIED.,.F.,.F.,(3,3),(0.,1.),.UNSPECIFIED.);
#375=B_SPLINE_CURVE_WITH_KNOTS('',2,(#82723,#82724,#82725),
 .UNSPECIFIED.,.F.,.F.,(3,3),(0.,1.),.UNSPECIFIED.);
#376=B_SPLINE_CURVE_WITH_KNOTS('',2,(#82728,#82729,#82730),
 .UNSPECIFIED.,.F.,.F.,(3,3),(0.,1.),.UNSPECIFIED.);
#377=B_SPLINE_CURVE_WITH_KNOTS('',2,(#82738,#82739,#82740),
 .UNSPECIFIED.,.F.,.F.,(3,3),(0.,1.),.UNSPECIFIED.);
#378=B_SPLINE_CURVE_WITH_KNOTS('',2,(#82743,#82744,#82745),
 .UNSPECIFIED.,.F.,.F.,(3,3),(0.,1.),.UNSPECIFIED.);
#379=B_SPLINE_CURVE_WITH_KNOTS('',2,(#82753,#82754,#82755),
 .UNSPECIFIED.,.F.,.F.,(3,3),(0.,1.),.UNSPECIFIED.);
#380=B_SPLINE_CURVE_WITH_KNOTS('',2,(#82758,#82759,#82760),
 .UNSPECIFIED.,.F.,.F.,(3,3),(0.,1.),.UNSPECIFIED.);
#381=B_SPLINE_CURVE_WITH_KNOTS('',2,(#82768,#82769,#82770),
 .UNSPECIFIED.,.F.,.F.,(3,3),(0.,1.),.UNSPECIFIED.);
#382=B_SPLINE_CURVE_WITH_KNOTS('',2,(#82773,#82774,#82775),
 .UNSPECIFIED.,.F.,.F.,(3,3),(0.,1.),.UNSPECIFIED.);
#383=B_SPLINE_CURVE_WITH_KNOTS('',2,(#82783,#82784,#82785),
 .UNSPECIFIED.,.F.,.F.,(3,3),(0.,1.),.UNSPECIFIED.);
#384=B_SPLINE_CURVE_WITH_KNOTS('',2,(#82788,#82789,#82790),
 .UNSPECIFIED.,.F.,.F.,(3,3),(0.,1.),.UNSPECIFIED.);
#385=B_SPLINE_CURVE_WITH_KNOTS('',2,(#82798,#82799,#82800),
 .UNSPECIFIED.,.F.,.F.,(3,3),(0.,1.),.UNSPECIFIED.);
#386=B_SPLINE_CURVE_WITH_KNOTS('',2,(#82803,#82804,#82805),
 .UNSPECIFIED.,.F.,.F.,(3,3),(0.,1.),.UNSPECIFIED.);
#387=B_SPLINE_CURVE_WITH_KNOTS('',2,(#82812,#82813,#82814),
 .UNSPECIFIED.,.F.,.F.,(3,3),(0.,1.),.UNSPECIFIED.);
#388=B_SPLINE_CURVE_WITH_KNOTS('',2,(#82815,#82816,#82817),
 .UNSPECIFIED.,.F.,.F.,(3,3),(0.,1.),.UNSPECIFIED.);
#389=B_SPLINE_CURVE_WITH_KNOTS('',2,(#82827,#82828,#82829),
 .UNSPECIFIED.,.F.,.F.,(3,3),(0.,1.),.UNSPECIFIED.);
#390=B_SPLINE_CURVE_WITH_KNOTS('',2,(#82833,#82834,#82835),
 .UNSPECIFIED.,.F.,.F.,(3,3),(0.,1.),.UNSPECIFIED.);
#391=B_SPLINE_CURVE_WITH_KNOTS('',2,(#82844,#82845,#82846),
 .UNSPECIFIED.,.F.,.F.,(3,3),(0.,1.),.UNSPECIFIED.);
#392=B_SPLINE_CURVE_WITH_KNOTS('',2,(#82849,#82850,#82851),
 .UNSPECIFIED.,.F.,.F.,(3,3),(0.,1.),.UNSPECIFIED.);
#393=B_SPLINE_CURVE_WITH_KNOTS('',2,(#82859,#82860,#82861),
 .UNSPECIFIED.,.F.,.F.,(3,3),(0.,1.),.UNSPECIFIED.);
#394=B_SPLINE_CURVE_WITH_KNOTS('',2,(#82864,#82865,#82866),
 .UNSPECIFIED.,.F.,.F.,(3,3),(0.,1.),.UNSPECIFIED.);
#395=B_SPLINE_CURVE_WITH_KNOTS('',2,(#82874,#82875,#82876),
 .UNSPECIFIED.,.F.,.F.,(3,3),(0.,1.),.UNSPECIFIED.);
#396=B_SPLINE_CURVE_WITH_KNOTS('',2,(#82879,#82880,#82881),
 .UNSPECIFIED.,.F.,.F.,(3,3),(0.,1.),.UNSPECIFIED.);
#397=B_SPLINE_CURVE_WITH_KNOTS('',2,(#82889,#82890,#82891),
 .UNSPECIFIED.,.F.,.F.,(3,3),(0.,1.),.UNSPECIFIED.);
#398=B_SPLINE_CURVE_WITH_KNOTS('',2,(#82894,#82895,#82896),
 .UNSPECIFIED.,.F.,.F.,(3,3),(0.,1.),.UNSPECIFIED.);
#399=B_SPLINE_CURVE_WITH_KNOTS('',2,(#82904,#82905,#82906),
 .UNSPECIFIED.,.F.,.F.,(3,3),(0.,1.),.UNSPECIFIED.);
#400=B_SPLINE_CURVE_WITH_KNOTS('',2,(#82909,#82910,#82911),
 .UNSPECIFIED.,.F.,.F.,(3,3),(0.,1.),.UNSPECIFIED.);
#401=B_SPLINE_CURVE_WITH_KNOTS('',2,(#82919,#82920,#82921),
 .UNSPECIFIED.,.F.,.F.,(3,3),(0.,1.),.UNSPECIFIED.);
#402=B_SPLINE_CURVE_WITH_KNOTS('',2,(#82924,#82925,#82926),
 .UNSPECIFIED.,.F.,.F.,(3,3),(0.,1.),.UNSPECIFIED.);
#403=B_SPLINE_CURVE_WITH_KNOTS('',2,(#82934,#82935,#82936),
 .UNSPECIFIED.,.F.,.F.,(3,3),(0.,1.),.UNSPECIFIED.);
#404=B_SPLINE_CURVE_WITH_KNOTS('',2,(#82939,#82940,#82941),
 .UNSPECIFIED.,.F.,.F.,(3,3),(0.,1.),.UNSPECIFIED.);
#405=B_SPLINE_CURVE_WITH_KNOTS('',2,(#82949,#82950,#82951),
 .UNSPECIFIED.,.F.,.F.,(3,3),(0.,1.),.UNSPECIFIED.);
#406=B_SPLINE_CURVE_WITH_KNOTS('',2,(#82954,#82955,#82956),
 .UNSPECIFIED.,.F.,.F.,(3,3),(0.,1.),.UNSPECIFIED.);
#407=B_SPLINE_CURVE_WITH_KNOTS('',2,(#82964,#82965,#82966),
 .UNSPECIFIED.,.F.,.F.,(3,3),(0.,1.),.UNSPECIFIED.);
#408=B_SPLINE_CURVE_WITH_KNOTS('',2,(#82969,#82970,#82971),
 .UNSPECIFIED.,.F.,.F.,(3,3),(0.,1.),.UNSPECIFIED.);
#409=B_SPLINE_CURVE_WITH_KNOTS('',2,(#82979,#82980,#82981),
 .UNSPECIFIED.,.F.,.F.,(3,3),(0.,1.),.UNSPECIFIED.);
#410=B_SPLINE_CURVE_WITH_KNOTS('',2,(#82984,#82985,#82986),
 .UNSPECIFIED.,.F.,.F.,(3,3),(0.,1.),.UNSPECIFIED.);
#411=B_SPLINE_CURVE_WITH_KNOTS('',2,(#83000,#83001,#83002),
 .UNSPECIFIED.,.F.,.F.,(3,3),(0.,1.),.UNSPECIFIED.);
#412=B_SPLINE_CURVE_WITH_KNOTS('',2,(#83005,#83006,#83007),
 .UNSPECIFIED.,.F.,.F.,(3,3),(0.,1.),.UNSPECIFIED.);
#413=B_SPLINE_CURVE_WITH_KNOTS('',2,(#83015,#83016,#83017),
 .UNSPECIFIED.,.F.,.F.,(3,3),(0.,1.),.UNSPECIFIED.);
#414=B_SPLINE_CURVE_WITH_KNOTS('',2,(#83020,#83021,#83022),
 .UNSPECIFIED.,.F.,.F.,(3,3),(0.,1.),.UNSPECIFIED.);
#415=B_SPLINE_CURVE_WITH_KNOTS('',2,(#83029,#83030,#83031),
 .UNSPECIFIED.,.F.,.F.,(3,3),(0.,1.),.UNSPECIFIED.);
#416=B_SPLINE_CURVE_WITH_KNOTS('',2,(#83032,#83033,#83034),
 .UNSPECIFIED.,.F.,.F.,(3,3),(0.,1.),.UNSPECIFIED.);
#417=B_SPLINE_CURVE_WITH_KNOTS('',2,(#83142,#83143,#83144),
 .UNSPECIFIED.,.F.,.F.,(3,3),(0.,1.),.UNSPECIFIED.);
#418=B_SPLINE_CURVE_WITH_KNOTS('',2,(#83148,#83149,#83150),
 .UNSPECIFIED.,.F.,.F.,(3,3),(0.,1.),.UNSPECIFIED.);
#419=B_SPLINE_CURVE_WITH_KNOTS('',2,(#83159,#83160,#83161),
 .UNSPECIFIED.,.F.,.F.,(3,3),(0.,1.),.UNSPECIFIED.);
#420=B_SPLINE_CURVE_WITH_KNOTS('',2,(#83164,#83165,#83166),
 .UNSPECIFIED.,.F.,.F.,(3,3),(0.,1.),.UNSPECIFIED.);
#421=B_SPLINE_CURVE_WITH_KNOTS('',2,(#83174,#83175,#83176),
 .UNSPECIFIED.,.F.,.F.,(3,3),(0.,1.),.UNSPECIFIED.);
#422=B_SPLINE_CURVE_WITH_KNOTS('',2,(#83179,#83180,#83181),
 .UNSPECIFIED.,.F.,.F.,(3,3),(0.,1.),.UNSPECIFIED.);
#423=B_SPLINE_CURVE_WITH_KNOTS('',2,(#83189,#83190,#83191),
 .UNSPECIFIED.,.F.,.F.,(3,3),(0.,1.),.UNSPECIFIED.);
#424=B_SPLINE_CURVE_WITH_KNOTS('',2,(#83194,#83195,#83196),
 .UNSPECIFIED.,.F.,.F.,(3,3),(0.,1.),.UNSPECIFIED.);
#425=B_SPLINE_CURVE_WITH_KNOTS('',2,(#83204,#83205,#83206),
 .UNSPECIFIED.,.F.,.F.,(3,3),(0.,1.),.UNSPECIFIED.);
#426=B_SPLINE_CURVE_WITH_KNOTS('',2,(#83209,#83210,#83211),
 .UNSPECIFIED.,.F.,.F.,(3,3),(0.,1.),.UNSPECIFIED.);
#427=B_SPLINE_CURVE_WITH_KNOTS('',2,(#83219,#83220,#83221),
 .UNSPECIFIED.,.F.,.F.,(3,3),(0.,1.),.UNSPECIFIED.);
#428=B_SPLINE_CURVE_WITH_KNOTS('',2,(#83224,#83225,#83226),
 .UNSPECIFIED.,.F.,.F.,(3,3),(0.,1.),.UNSPECIFIED.);
#429=B_SPLINE_CURVE_WITH_KNOTS('',2,(#83234,#83235,#83236),
 .UNSPECIFIED.,.F.,.F.,(3,3),(0.,1.),.UNSPECIFIED.);
#430=B_SPLINE_CURVE_WITH_KNOTS('',2,(#83239,#83240,#83241),
 .UNSPECIFIED.,.F.,.F.,(3,3),(0.,1.),.UNSPECIFIED.);
#431=B_SPLINE_CURVE_WITH_KNOTS('',2,(#83249,#83250,#83251),
 .UNSPECIFIED.,.F.,.F.,(3,3),(0.,1.),.UNSPECIFIED.);
#432=B_SPLINE_CURVE_WITH_KNOTS('',2,(#83254,#83255,#83256),
 .UNSPECIFIED.,.F.,.F.,(3,3),(0.,1.),.UNSPECIFIED.);
#433=B_SPLINE_CURVE_WITH_KNOTS('',2,(#83264,#83265,#83266),
 .UNSPECIFIED.,.F.,.F.,(3,3),(0.,1.),.UNSPECIFIED.);
#434=B_SPLINE_CURVE_WITH_KNOTS('',2,(#83269,#83270,#83271),
 .UNSPECIFIED.,.F.,.F.,(3,3),(0.,1.),.UNSPECIFIED.);
#435=B_SPLINE_CURVE_WITH_KNOTS('',2,(#83279,#83280,#83281),
 .UNSPECIFIED.,.F.,.F.,(3,3),(0.,1.),.UNSPECIFIED.);
#436=B_SPLINE_CURVE_WITH_KNOTS('',2,(#83284,#83285,#83286),
 .UNSPECIFIED.,.F.,.F.,(3,3),(0.,1.),.UNSPECIFIED.);
#437=B_SPLINE_CURVE_WITH_KNOTS('',2,(#83293,#83294,#83295),
 .UNSPECIFIED.,.F.,.F.,(3,3),(0.,1.),.UNSPECIFIED.);
#438=B_SPLINE_CURVE_WITH_KNOTS('',2,(#83296,#83297,#83298),
 .UNSPECIFIED.,.F.,.F.,(3,3),(0.,1.),.UNSPECIFIED.);
#439=B_SPLINE_CURVE_WITH_KNOTS('',2,(#83418,#83419,#83420),
 .UNSPECIFIED.,.F.,.F.,(3,3),(0.,1.),.UNSPECIFIED.);
#440=B_SPLINE_CURVE_WITH_KNOTS('',2,(#83424,#83425,#83426),
 .UNSPECIFIED.,.F.,.F.,(3,3),(0.,1.),.UNSPECIFIED.);
#441=B_SPLINE_CURVE_WITH_KNOTS('',2,(#83435,#83436,#83437),
 .UNSPECIFIED.,.F.,.F.,(3,3),(0.,1.),.UNSPECIFIED.);
#442=B_SPLINE_CURVE_WITH_KNOTS('',2,(#83440,#83441,#83442),
 .UNSPECIFIED.,.F.,.F.,(3,3),(0.,1.),.UNSPECIFIED.);
#443=B_SPLINE_CURVE_WITH_KNOTS('',2,(#83450,#83451,#83452),
 .UNSPECIFIED.,.F.,.F.,(3,3),(0.,1.),.UNSPECIFIED.);
#444=B_SPLINE_CURVE_WITH_KNOTS('',2,(#83455,#83456,#83457),
 .UNSPECIFIED.,.F.,.F.,(3,3),(0.,1.),.UNSPECIFIED.);
#445=B_SPLINE_CURVE_WITH_KNOTS('',2,(#83465,#83466,#83467),
 .UNSPECIFIED.,.F.,.F.,(3,3),(0.,1.),.UNSPECIFIED.);
#446=B_SPLINE_CURVE_WITH_KNOTS('',2,(#83470,#83471,#83472),
 .UNSPECIFIED.,.F.,.F.,(3,3),(0.,1.),.UNSPECIFIED.);
#447=B_SPLINE_CURVE_WITH_KNOTS('',2,(#83480,#83481,#83482),
 .UNSPECIFIED.,.F.,.F.,(3,3),(0.,1.),.UNSPECIFIED.);
#448=B_SPLINE_CURVE_WITH_KNOTS('',2,(#83485,#83486,#83487),
 .UNSPECIFIED.,.F.,.F.,(3,3),(0.,1.),.UNSPECIFIED.);
#449=B_SPLINE_CURVE_WITH_KNOTS('',2,(#83495,#83496,#83497),
 .UNSPECIFIED.,.F.,.F.,(3,3),(0.,1.),.UNSPECIFIED.);
#450=B_SPLINE_CURVE_WITH_KNOTS('',2,(#83500,#83501,#83502),
 .UNSPECIFIED.,.F.,.F.,(3,3),(0.,1.),.UNSPECIFIED.);
#451=B_SPLINE_CURVE_WITH_KNOTS('',2,(#83510,#83511,#83512),
 .UNSPECIFIED.,.F.,.F.,(3,3),(0.,1.),.UNSPECIFIED.);
#452=B_SPLINE_CURVE_WITH_KNOTS('',2,(#83515,#83516,#83517),
 .UNSPECIFIED.,.F.,.F.,(3,3),(0.,1.),.UNSPECIFIED.);
#453=B_SPLINE_CURVE_WITH_KNOTS('',2,(#83525,#83526,#83527),
 .UNSPECIFIED.,.F.,.F.,(3,3),(0.,1.),.UNSPECIFIED.);
#454=B_SPLINE_CURVE_WITH_KNOTS('',2,(#83530,#83531,#83532),
 .UNSPECIFIED.,.F.,.F.,(3,3),(0.,1.),.UNSPECIFIED.);
#455=B_SPLINE_CURVE_WITH_KNOTS('',2,(#83557,#83558,#83559),
 .UNSPECIFIED.,.F.,.F.,(3,3),(0.,1.),.UNSPECIFIED.);
#456=B_SPLINE_CURVE_WITH_KNOTS('',2,(#83560,#83561,#83562),
 .UNSPECIFIED.,.F.,.F.,(3,3),(0.,1.),.UNSPECIFIED.);
#457=B_SPLINE_CURVE_WITH_KNOTS('',2,(#83580,#83581,#83582),
 .UNSPECIFIED.,.F.,.F.,(3,3),(0.,1.),.UNSPECIFIED.);
#458=B_SPLINE_CURVE_WITH_KNOTS('',2,(#83585,#83586,#83587),
 .UNSPECIFIED.,.F.,.F.,(3,3),(0.,1.),.UNSPECIFIED.);
#459=B_SPLINE_CURVE_WITH_KNOTS('',2,(#83595,#83596,#83597),
 .UNSPECIFIED.,.F.,.F.,(3,3),(0.,1.),.UNSPECIFIED.);
#460=B_SPLINE_CURVE_WITH_KNOTS('',2,(#83600,#83601,#83602),
 .UNSPECIFIED.,.F.,.F.,(3,3),(0.,1.),.UNSPECIFIED.);
#461=B_SPLINE_CURVE_WITH_KNOTS('',2,(#83610,#83611,#83612),
 .UNSPECIFIED.,.F.,.F.,(3,3),(0.,1.),.UNSPECIFIED.);
#462=B_SPLINE_CURVE_WITH_KNOTS('',2,(#83615,#83616,#83617),
 .UNSPECIFIED.,.F.,.F.,(3,3),(0.,1.),.UNSPECIFIED.);
#463=B_SPLINE_CURVE_WITH_KNOTS('',2,(#83625,#83626,#83627),
 .UNSPECIFIED.,.F.,.F.,(3,3),(0.,1.),.UNSPECIFIED.);
#464=B_SPLINE_CURVE_WITH_KNOTS('',2,(#83630,#83631,#83632),
 .UNSPECIFIED.,.F.,.F.,(3,3),(0.,1.),.UNSPECIFIED.);
#465=B_SPLINE_CURVE_WITH_KNOTS('',2,(#83658,#83659,#83660),
 .UNSPECIFIED.,.F.,.F.,(3,3),(0.,1.),.UNSPECIFIED.);
#466=B_SPLINE_CURVE_WITH_KNOTS('',2,(#83663,#83664,#83665),
 .UNSPECIFIED.,.F.,.F.,(3,3),(0.,1.),.UNSPECIFIED.);
#467=B_SPLINE_CURVE_WITH_KNOTS('',2,(#83673,#83674,#83675),
 .UNSPECIFIED.,.F.,.F.,(3,3),(0.,1.),.UNSPECIFIED.);
#468=B_SPLINE_CURVE_WITH_KNOTS('',2,(#83678,#83679,#83680),
 .UNSPECIFIED.,.F.,.F.,(3,3),(0.,1.),.UNSPECIFIED.);
#469=B_SPLINE_CURVE_WITH_KNOTS('',2,(#83688,#83689,#83690),
 .UNSPECIFIED.,.F.,.F.,(3,3),(0.,1.),.UNSPECIFIED.);
#470=B_SPLINE_CURVE_WITH_KNOTS('',2,(#83693,#83694,#83695),
 .UNSPECIFIED.,.F.,.F.,(3,3),(0.,1.),.UNSPECIFIED.);
#471=B_SPLINE_CURVE_WITH_KNOTS('',2,(#83703,#83704,#83705),
 .UNSPECIFIED.,.F.,.F.,(3,3),(0.,1.),.UNSPECIFIED.);
#472=B_SPLINE_CURVE_WITH_KNOTS('',2,(#83708,#83709,#83710),
 .UNSPECIFIED.,.F.,.F.,(3,3),(0.,1.),.UNSPECIFIED.);
#473=B_SPLINE_CURVE_WITH_KNOTS('',2,(#83718,#83719,#83720),
 .UNSPECIFIED.,.F.,.F.,(3,3),(0.,1.),.UNSPECIFIED.);
#474=B_SPLINE_CURVE_WITH_KNOTS('',2,(#83723,#83724,#83725),
 .UNSPECIFIED.,.F.,.F.,(3,3),(0.,1.),.UNSPECIFIED.);
#475=B_SPLINE_CURVE_WITH_KNOTS('',2,(#83733,#83734,#83735),
 .UNSPECIFIED.,.F.,.F.,(3,3),(0.,1.),.UNSPECIFIED.);
#476=B_SPLINE_CURVE_WITH_KNOTS('',2,(#83738,#83739,#83740),
 .UNSPECIFIED.,.F.,.F.,(3,3),(0.,1.),.UNSPECIFIED.);
#477=B_SPLINE_CURVE_WITH_KNOTS('',2,(#83748,#83749,#83750),
 .UNSPECIFIED.,.F.,.F.,(3,3),(0.,1.),.UNSPECIFIED.);
#478=B_SPLINE_CURVE_WITH_KNOTS('',2,(#83753,#83754,#83755),
 .UNSPECIFIED.,.F.,.F.,(3,3),(0.,1.),.UNSPECIFIED.);
#719=B_SPLINE_SURFACE_WITH_KNOTS('',2,1,((#80625,#80626),(#80627,#80628),
(#80629,#80630)),.UNSPECIFIED.,.F.,.F.,.F.,(3,3),(2,2),(0.,1.),(0.,0.03),
 .UNSPECIFIED.);
#720=B_SPLINE_SURFACE_WITH_KNOTS('',2,1,((#80643,#80644),(#80645,#80646),
(#80647,#80648)),.UNSPECIFIED.,.F.,.F.,.F.,(3,3),(2,2),(0.,1.),(0.,0.03),
 .UNSPECIFIED.);
#721=B_SPLINE_SURFACE_WITH_KNOTS('',2,1,((#80658,#80659),(#80660,#80661),
(#80662,#80663)),.UNSPECIFIED.,.F.,.F.,.F.,(3,3),(2,2),(0.,1.),(0.,0.03),
 .UNSPECIFIED.);
#722=B_SPLINE_SURFACE_WITH_KNOTS('',2,1,((#80673,#80674),(#80675,#80676),
(#80677,#80678)),.UNSPECIFIED.,.F.,.F.,.F.,(3,3),(2,2),(0.,1.),(0.,0.03),
 .UNSPECIFIED.);
#723=B_SPLINE_SURFACE_WITH_KNOTS('',2,1,((#80688,#80689),(#80690,#80691),
(#80692,#80693)),.UNSPECIFIED.,.F.,.F.,.F.,(3,3),(2,2),(0.,1.),(0.,0.03),
 .UNSPECIFIED.);
#724=B_SPLINE_SURFACE_WITH_KNOTS('',2,1,((#80703,#80704),(#80705,#80706),
(#80707,#80708)),.UNSPECIFIED.,.F.,.F.,.F.,(3,3),(2,2),(0.,1.),(0.,0.03),
 .UNSPECIFIED.);
#725=B_SPLINE_SURFACE_WITH_KNOTS('',2,1,((#80718,#80719),(#80720,#80721),
(#80722,#80723)),.UNSPECIFIED.,.F.,.F.,.F.,(3,3),(2,2),(0.,1.),(0.,0.03),
 .UNSPECIFIED.);
#726=B_SPLINE_SURFACE_WITH_KNOTS('',2,1,((#80733,#80734),(#80735,#80736),
(#80737,#80738)),.UNSPECIFIED.,.F.,.F.,.F.,(3,3),(2,2),(0.,1.),(0.,0.03),
 .UNSPECIFIED.);
#727=B_SPLINE_SURFACE_WITH_KNOTS('',2,1,((#80748,#80749),(#80750,#80751),
(#80752,#80753)),.UNSPECIFIED.,.F.,.F.,.F.,(3,3),(2,2),(0.,1.),(0.,0.03),
 .UNSPECIFIED.);
#728=B_SPLINE_SURFACE_WITH_KNOTS('',2,1,((#80763,#80764),(#80765,#80766),
(#80767,#80768)),.UNSPECIFIED.,.F.,.F.,.F.,(3,3),(2,2),(0.,1.),(0.,0.03),
 .UNSPECIFIED.);
#729=B_SPLINE_SURFACE_WITH_KNOTS('',2,1,((#80778,#80779),(#80780,#80781),
(#80782,#80783)),.UNSPECIFIED.,.F.,.F.,.F.,(3,3),(2,2),(0.,1.),(0.,0.03),
 .UNSPECIFIED.);
#730=B_SPLINE_SURFACE_WITH_KNOTS('',2,1,((#80793,#80794),(#80795,#80796),
(#80797,#80798)),.UNSPECIFIED.,.F.,.F.,.F.,(3,3),(2,2),(0.,1.),(0.,0.03),
 .UNSPECIFIED.);
#731=B_SPLINE_SURFACE_WITH_KNOTS('',2,1,((#80808,#80809),(#80810,#80811),
(#80812,#80813)),.UNSPECIFIED.,.F.,.F.,.F.,(3,3),(2,2),(0.,1.),(0.,0.03),
 .UNSPECIFIED.);
#732=B_SPLINE_SURFACE_WITH_KNOTS('',2,1,((#80829,#80830),(#80831,#80832),
(#80833,#80834)),.UNSPECIFIED.,.F.,.F.,.F.,(3,3),(2,2),(0.,1.),(0.,0.03),
 .UNSPECIFIED.);
#733=B_SPLINE_SURFACE_WITH_KNOTS('',2,1,((#80844,#80845),(#80846,#80847),
(#80848,#80849)),.UNSPECIFIED.,.F.,.F.,.F.,(3,3),(2,2),(0.,1.),(0.,0.03),
 .UNSPECIFIED.);
#734=B_SPLINE_SURFACE_WITH_KNOTS('',2,1,((#80859,#80860),(#80861,#80862),
(#80863,#80864)),.UNSPECIFIED.,.F.,.F.,.F.,(3,3),(2,2),(0.,1.),(0.,0.03),
 .UNSPECIFIED.);
#735=B_SPLINE_SURFACE_WITH_KNOTS('',2,1,((#80874,#80875),(#80876,#80877),
(#80878,#80879)),.UNSPECIFIED.,.F.,.F.,.F.,(3,3),(2,2),(0.,1.),(0.,0.03),
 .UNSPECIFIED.);
#736=B_SPLINE_SURFACE_WITH_KNOTS('',2,1,((#80889,#80890),(#80891,#80892),
(#80893,#80894)),.UNSPECIFIED.,.F.,.F.,.F.,(3,3),(2,2),(0.,1.),(0.,0.03),
 .UNSPECIFIED.);
#737=B_SPLINE_SURFACE_WITH_KNOTS('',2,1,((#80904,#80905),(#80906,#80907),
(#80908,#80909)),.UNSPECIFIED.,.F.,.F.,.F.,(3,3),(2,2),(0.,1.),(0.,0.03),
 .UNSPECIFIED.);
#738=B_SPLINE_SURFACE_WITH_KNOTS('',2,1,((#80919,#80920),(#80921,#80922),
(#80923,#80924)),.UNSPECIFIED.,.F.,.F.,.F.,(3,3),(2,2),(0.,1.),(0.,0.03),
 .UNSPECIFIED.);
#739=B_SPLINE_SURFACE_WITH_KNOTS('',2,1,((#80934,#80935),(#80936,#80937),
(#80938,#80939)),.UNSPECIFIED.,.F.,.F.,.F.,(3,3),(2,2),(0.,1.),(0.,0.03),
 .UNSPECIFIED.);
#740=B_SPLINE_SURFACE_WITH_KNOTS('',2,1,((#80949,#80950),(#80951,#80952),
(#80953,#80954)),.UNSPECIFIED.,.F.,.F.,.F.,(3,3),(2,2),(0.,1.),(0.,0.03),
 .UNSPECIFIED.);
#741=B_SPLINE_SURFACE_WITH_KNOTS('',2,1,((#80964,#80965),(#80966,#80967),
(#80968,#80969)),.UNSPECIFIED.,.F.,.F.,.F.,(3,3),(2,2),(0.,1.),(0.,0.03),
 .UNSPECIFIED.);
#742=B_SPLINE_SURFACE_WITH_KNOTS('',2,1,((#80979,#80980),(#80981,#80982),
(#80983,#80984)),.UNSPECIFIED.,.F.,.F.,.F.,(3,3),(2,2),(0.,1.),(0.,0.03),
 .UNSPECIFIED.);
#743=B_SPLINE_SURFACE_WITH_KNOTS('',2,1,((#80994,#80995),(#80996,#80997),
(#80998,#80999)),.UNSPECIFIED.,.F.,.F.,.F.,(3,3),(2,2),(0.,1.),(0.,0.03),
 .UNSPECIFIED.);
#744=B_SPLINE_SURFACE_WITH_KNOTS('',2,1,((#81009,#81010),(#81011,#81012),
(#81013,#81014)),.UNSPECIFIED.,.F.,.F.,.F.,(3,3),(2,2),(0.,1.),(0.,0.03),
 .UNSPECIFIED.);
#745=B_SPLINE_SURFACE_WITH_KNOTS('',2,1,((#81024,#81025),(#81026,#81027),
(#81028,#81029)),.UNSPECIFIED.,.F.,.F.,.F.,(3,3),(2,2),(0.,1.),(0.,0.03),
 .UNSPECIFIED.);
#746=B_SPLINE_SURFACE_WITH_KNOTS('',2,1,((#81039,#81040),(#81041,#81042),
(#81043,#81044)),.UNSPECIFIED.,.F.,.F.,.F.,(3,3),(2,2),(0.,1.),(0.,0.03),
 .UNSPECIFIED.);
#747=B_SPLINE_SURFACE_WITH_KNOTS('',2,1,((#81054,#81055),(#81056,#81057),
(#81058,#81059)),.UNSPECIFIED.,.F.,.F.,.F.,(3,3),(2,2),(0.,1.),(0.,0.03),
 .UNSPECIFIED.);
#748=B_SPLINE_SURFACE_WITH_KNOTS('',2,1,((#81069,#81070),(#81071,#81072),
(#81073,#81074)),.UNSPECIFIED.,.F.,.F.,.F.,(3,3),(2,2),(0.,1.),(0.,0.03),
 .UNSPECIFIED.);
#749=B_SPLINE_SURFACE_WITH_KNOTS('',2,1,((#81084,#81085),(#81086,#81087),
(#81088,#81089)),.UNSPECIFIED.,.F.,.F.,.F.,(3,3),(2,2),(0.,1.),(0.,0.03),
 .UNSPECIFIED.);
#750=B_SPLINE_SURFACE_WITH_KNOTS('',2,1,((#81105,#81106),(#81107,#81108),
(#81109,#81110)),.UNSPECIFIED.,.F.,.F.,.F.,(3,3),(2,2),(0.,1.),(0.,0.03),
 .UNSPECIFIED.);
#751=B_SPLINE_SURFACE_WITH_KNOTS('',2,1,((#81120,#81121),(#81122,#81123),
(#81124,#81125)),.UNSPECIFIED.,.F.,.F.,.F.,(3,3),(2,2),(0.,1.),(0.,0.03),
 .UNSPECIFIED.);
#752=B_SPLINE_SURFACE_WITH_KNOTS('',2,1,((#81133,#81134),(#81135,#81136),
(#81137,#81138)),.UNSPECIFIED.,.F.,.F.,.F.,(3,3),(2,2),(0.,1.),(0.,0.03),
 .UNSPECIFIED.);
#753=B_SPLINE_SURFACE_WITH_KNOTS('',2,1,((#81151,#81152),(#81153,#81154),
(#81155,#81156)),.UNSPECIFIED.,.F.,.F.,.F.,(3,3),(2,2),(0.,1.),(0.,0.03),
 .UNSPECIFIED.);
#754=B_SPLINE_SURFACE_WITH_KNOTS('',2,1,((#81166,#81167),(#81168,#81169),
(#81170,#81171)),.UNSPECIFIED.,.F.,.F.,.F.,(3,3),(2,2),(0.,1.),(0.,0.03),
 .UNSPECIFIED.);
#755=B_SPLINE_SURFACE_WITH_KNOTS('',2,1,((#81181,#81182),(#81183,#81184),
(#81185,#81186)),.UNSPECIFIED.,.F.,.F.,.F.,(3,3),(2,2),(0.,1.),(0.,0.03),
 .UNSPECIFIED.);
#756=B_SPLINE_SURFACE_WITH_KNOTS('',2,1,((#81196,#81197),(#81198,#81199),
(#81200,#81201)),.UNSPECIFIED.,.F.,.F.,.F.,(3,3),(2,2),(0.,1.),(0.,0.03),
 .UNSPECIFIED.);
#757=B_SPLINE_SURFACE_WITH_KNOTS('',2,1,((#81211,#81212),(#81213,#81214),
(#81215,#81216)),.UNSPECIFIED.,.F.,.F.,.F.,(3,3),(2,2),(0.,1.),(0.,0.03),
 .UNSPECIFIED.);
#758=B_SPLINE_SURFACE_WITH_KNOTS('',2,1,((#81226,#81227),(#81228,#81229),
(#81230,#81231)),.UNSPECIFIED.,.F.,.F.,.F.,(3,3),(2,2),(0.,1.),(0.,0.03),
 .UNSPECIFIED.);
#759=B_SPLINE_SURFACE_WITH_KNOTS('',2,1,((#81241,#81242),(#81243,#81244),
(#81245,#81246)),.UNSPECIFIED.,.F.,.F.,.F.,(3,3),(2,2),(0.,1.),(0.,0.03),
 .UNSPECIFIED.);
#760=B_SPLINE_SURFACE_WITH_KNOTS('',2,1,((#81262,#81263),(#81264,#81265),
(#81266,#81267)),.UNSPECIFIED.,.F.,.F.,.F.,(3,3),(2,2),(0.,1.),(0.,0.03),
 .UNSPECIFIED.);
#761=B_SPLINE_SURFACE_WITH_KNOTS('',2,1,((#81277,#81278),(#81279,#81280),
(#81281,#81282)),.UNSPECIFIED.,.F.,.F.,.F.,(3,3),(2,2),(0.,1.),(0.,0.03),
 .UNSPECIFIED.);
#762=B_SPLINE_SURFACE_WITH_KNOTS('',2,1,((#81292,#81293),(#81294,#81295),
(#81296,#81297)),.UNSPECIFIED.,.F.,.F.,.F.,(3,3),(2,2),(0.,1.),(0.,0.03),
 .UNSPECIFIED.);
#763=B_SPLINE_SURFACE_WITH_KNOTS('',2,1,((#81307,#81308),(#81309,#81310),
(#81311,#81312)),.UNSPECIFIED.,.F.,.F.,.F.,(3,3),(2,2),(0.,1.),(0.,0.03),
 .UNSPECIFIED.);
#764=B_SPLINE_SURFACE_WITH_KNOTS('',2,1,((#81322,#81323),(#81324,#81325),
(#81326,#81327)),.UNSPECIFIED.,.F.,.F.,.F.,(3,3),(2,2),(0.,1.),(0.,0.03),
 .UNSPECIFIED.);
#765=B_SPLINE_SURFACE_WITH_KNOTS('',2,1,((#81337,#81338),(#81339,#81340),
(#81341,#81342)),.UNSPECIFIED.,.F.,.F.,.F.,(3,3),(2,2),(0.,1.),(0.,0.03),
 .UNSPECIFIED.);
#766=B_SPLINE_SURFACE_WITH_KNOTS('',2,1,((#81352,#81353),(#81354,#81355),
(#81356,#81357)),.UNSPECIFIED.,.F.,.F.,.F.,(3,3),(2,2),(0.,1.),(0.,0.03),
 .UNSPECIFIED.);
#767=B_SPLINE_SURFACE_WITH_KNOTS('',2,1,((#81367,#81368),(#81369,#81370),
(#81371,#81372)),.UNSPECIFIED.,.F.,.F.,.F.,(3,3),(2,2),(0.,1.),(0.,0.03),
 .UNSPECIFIED.);
#768=B_SPLINE_SURFACE_WITH_KNOTS('',2,1,((#81382,#81383),(#81384,#81385),
(#81386,#81387)),.UNSPECIFIED.,.F.,.F.,.F.,(3,3),(2,2),(0.,1.),(0.,0.03),
 .UNSPECIFIED.);
#769=B_SPLINE_SURFACE_WITH_KNOTS('',2,1,((#81397,#81398),(#81399,#81400),
(#81401,#81402)),.UNSPECIFIED.,.F.,.F.,.F.,(3,3),(2,2),(0.,1.),(0.,0.03),
 .UNSPECIFIED.);
#770=B_SPLINE_SURFACE_WITH_KNOTS('',2,1,((#81418,#81419),(#81420,#81421),
(#81422,#81423)),.UNSPECIFIED.,.F.,.F.,.F.,(3,3),(2,2),(0.,1.),(0.,0.03),
 .UNSPECIFIED.);
#771=B_SPLINE_SURFACE_WITH_KNOTS('',2,1,((#81433,#81434),(#81435,#81436),
(#81437,#81438)),.UNSPECIFIED.,.F.,.F.,.F.,(3,3),(2,2),(0.,1.),(0.,0.03),
 .UNSPECIFIED.);
#772=B_SPLINE_SURFACE_WITH_KNOTS('',2,1,((#81532,#81533),(#81534,#81535),
(#81536,#81537)),.UNSPECIFIED.,.F.,.F.,.F.,(3,3),(2,2),(0.,1.),(0.,0.03),
 .UNSPECIFIED.);
#773=B_SPLINE_SURFACE_WITH_KNOTS('',2,1,((#81550,#81551),(#81552,#81553),
(#81554,#81555)),.UNSPECIFIED.,.F.,.F.,.F.,(3,3),(2,2),(0.,1.),(0.,0.03),
 .UNSPECIFIED.);
#774=B_SPLINE_SURFACE_WITH_KNOTS('',2,1,((#81565,#81566),(#81567,#81568),
(#81569,#81570)),.UNSPECIFIED.,.F.,.F.,.F.,(3,3),(2,2),(0.,1.),(0.,0.03),
 .UNSPECIFIED.);
#775=B_SPLINE_SURFACE_WITH_KNOTS('',2,1,((#81580,#81581),(#81582,#81583),
(#81584,#81585)),.UNSPECIFIED.,.F.,.F.,.F.,(3,3),(2,2),(0.,1.),(0.,0.03),
 .UNSPECIFIED.);
#776=B_SPLINE_SURFACE_WITH_KNOTS('',2,1,((#81613,#81614),(#81615,#81616),
(#81617,#81618)),.UNSPECIFIED.,.F.,.F.,.F.,(3,3),(2,2),(0.,1.),(0.,0.03),
 .UNSPECIFIED.);
#777=B_SPLINE_SURFACE_WITH_KNOTS('',2,1,((#81628,#81629),(#81630,#81631),
(#81632,#81633)),.UNSPECIFIED.,.F.,.F.,.F.,(3,3),(2,2),(0.,1.),(0.,0.03),
 .UNSPECIFIED.);
#778=B_SPLINE_SURFACE_WITH_KNOTS('',2,1,((#81643,#81644),(#81645,#81646),
(#81647,#81648)),.UNSPECIFIED.,.F.,.F.,.F.,(3,3),(2,2),(0.,1.),(0.,0.03),
 .UNSPECIFIED.);
#779=B_SPLINE_SURFACE_WITH_KNOTS('',2,1,((#81658,#81659),(#81660,#81661),
(#81662,#81663)),.UNSPECIFIED.,.F.,.F.,.F.,(3,3),(2,2),(0.,1.),(0.,0.03),
 .UNSPECIFIED.);
#780=B_SPLINE_SURFACE_WITH_KNOTS('',2,1,((#81673,#81674),(#81675,#81676),
(#81677,#81678)),.UNSPECIFIED.,.F.,.F.,.F.,(3,3),(2,2),(0.,1.),(0.,0.03),
 .UNSPECIFIED.);
#781=B_SPLINE_SURFACE_WITH_KNOTS('',2,1,((#81688,#81689),(#81690,#81691),
(#81692,#81693)),.UNSPECIFIED.,.F.,.F.,.F.,(3,3),(2,2),(0.,1.),(0.,0.03),
 .UNSPECIFIED.);
#782=B_SPLINE_SURFACE_WITH_KNOTS('',2,1,((#81721,#81722),(#81723,#81724),
(#81725,#81726)),.UNSPECIFIED.,.F.,.F.,.F.,(3,3),(2,2),(0.,1.),(0.,0.03),
 .UNSPECIFIED.);
#783=B_SPLINE_SURFACE_WITH_KNOTS('',2,1,((#81743,#81744),(#81745,#81746),
(#81747,#81748)),.UNSPECIFIED.,.F.,.F.,.F.,(3,3),(2,2),(0.,1.),(0.,0.03),
 .UNSPECIFIED.);
#784=B_SPLINE_SURFACE_WITH_KNOTS('',2,1,((#81758,#81759),(#81760,#81761),
(#81762,#81763)),.UNSPECIFIED.,.F.,.F.,.F.,(3,3),(2,2),(0.,1.),(0.,0.03),
 .UNSPECIFIED.);
#785=B_SPLINE_SURFACE_WITH_KNOTS('',2,1,((#81773,#81774),(#81775,#81776),
(#81777,#81778)),.UNSPECIFIED.,.F.,.F.,.F.,(3,3),(2,2),(0.,1.),(0.,0.03),
 .UNSPECIFIED.);
#786=B_SPLINE_SURFACE_WITH_KNOTS('',2,1,((#81788,#81789),(#81790,#81791),
(#81792,#81793)),.UNSPECIFIED.,.F.,.F.,.F.,(3,3),(2,2),(0.,1.),(0.,0.03),
 .UNSPECIFIED.);
#787=B_SPLINE_SURFACE_WITH_KNOTS('',2,1,((#81821,#81822),(#81823,#81824),
(#81825,#81826)),.UNSPECIFIED.,.F.,.F.,.F.,(3,3),(2,2),(0.,1.),(0.,0.03),
 .UNSPECIFIED.);
#788=B_SPLINE_SURFACE_WITH_KNOTS('',2,1,((#81836,#81837),(#81838,#81839),
(#81840,#81841)),.UNSPECIFIED.,.F.,.F.,.F.,(3,3),(2,2),(0.,1.),(0.,0.03),
 .UNSPECIFIED.);
#789=B_SPLINE_SURFACE_WITH_KNOTS('',2,1,((#81851,#81852),(#81853,#81854),
(#81855,#81856)),.UNSPECIFIED.,.F.,.F.,.F.,(3,3),(2,2),(0.,1.),(0.,0.03),
 .UNSPECIFIED.);
#790=B_SPLINE_SURFACE_WITH_KNOTS('',2,1,((#81866,#81867),(#81868,#81869),
(#81870,#81871)),.UNSPECIFIED.,.F.,.F.,.F.,(3,3),(2,2),(0.,1.),(0.,0.03),
 .UNSPECIFIED.);
#791=B_SPLINE_SURFACE_WITH_KNOTS('',2,1,((#81881,#81882),(#81883,#81884),
(#81885,#81886)),.UNSPECIFIED.,.F.,.F.,.F.,(3,3),(2,2),(0.,1.),(0.,0.03),
 .UNSPECIFIED.);
#792=B_SPLINE_SURFACE_WITH_KNOTS('',2,1,((#81896,#81897),(#81898,#81899),
(#81900,#81901)),.UNSPECIFIED.,.F.,.F.,.F.,(3,3),(2,2),(0.,1.),(0.,0.03),
 .UNSPECIFIED.);
#793=B_SPLINE_SURFACE_WITH_KNOTS('',2,1,((#81911,#81912),(#81913,#81914),
(#81915,#81916)),.UNSPECIFIED.,.F.,.F.,.F.,(3,3),(2,2),(0.,1.),(0.,0.03),
 .UNSPECIFIED.);
#794=B_SPLINE_SURFACE_WITH_KNOTS('',2,1,((#81997,#81998),(#81999,#82000),
(#82001,#82002)),.UNSPECIFIED.,.F.,.F.,.F.,(3,3),(2,2),(0.,1.),(0.,0.03),
 .UNSPECIFIED.);
#795=B_SPLINE_SURFACE_WITH_KNOTS('',2,1,((#82015,#82016),(#82017,#82018),
(#82019,#82020)),.UNSPECIFIED.,.F.,.F.,.F.,(3,3),(2,2),(0.,1.),(0.,0.03),
 .UNSPECIFIED.);
#796=B_SPLINE_SURFACE_WITH_KNOTS('',2,1,((#82036,#82037),(#82038,#82039),
(#82040,#82041)),.UNSPECIFIED.,.F.,.F.,.F.,(3,3),(2,2),(0.,1.),(0.,0.03),
 .UNSPECIFIED.);
#797=B_SPLINE_SURFACE_WITH_KNOTS('',2,1,((#82051,#82052),(#82053,#82054),
(#82055,#82056)),.UNSPECIFIED.,.F.,.F.,.F.,(3,3),(2,2),(0.,1.),(0.,0.03),
 .UNSPECIFIED.);
#798=B_SPLINE_SURFACE_WITH_KNOTS('',2,1,((#82088,#82089),(#82090,#82091),
(#82092,#82093)),.UNSPECIFIED.,.F.,.F.,.F.,(3,3),(2,2),(0.,1.),(0.,0.03),
 .UNSPECIFIED.);
#799=B_SPLINE_SURFACE_WITH_KNOTS('',2,1,((#82106,#82107),(#82108,#82109),
(#82110,#82111)),.UNSPECIFIED.,.F.,.F.,.F.,(3,3),(2,2),(0.,1.),(0.,0.03),
 .UNSPECIFIED.);
#800=B_SPLINE_SURFACE_WITH_KNOTS('',2,1,((#82121,#82122),(#82123,#82124),
(#82125,#82126)),.UNSPECIFIED.,.F.,.F.,.F.,(3,3),(2,2),(0.,1.),(0.,0.03),
 .UNSPECIFIED.);
#801=B_SPLINE_SURFACE_WITH_KNOTS('',2,1,((#82136,#82137),(#82138,#82139),
(#82140,#82141)),.UNSPECIFIED.,.F.,.F.,.F.,(3,3),(2,2),(0.,1.),(0.,0.03),
 .UNSPECIFIED.);
#802=B_SPLINE_SURFACE_WITH_KNOTS('',2,1,((#82151,#82152),(#82153,#82154),
(#82155,#82156)),.UNSPECIFIED.,.F.,.F.,.F.,(3,3),(2,2),(0.,1.),(0.,0.03),
 .UNSPECIFIED.);
#803=B_SPLINE_SURFACE_WITH_KNOTS('',2,1,((#82166,#82167),(#82168,#82169),
(#82170,#82171)),.UNSPECIFIED.,.F.,.F.,.F.,(3,3),(2,2),(0.,1.),(0.,0.03),
 .UNSPECIFIED.);
#804=B_SPLINE_SURFACE_WITH_KNOTS('',2,1,((#82181,#82182),(#82183,#82184),
(#82185,#82186)),.UNSPECIFIED.,.F.,.F.,.F.,(3,3),(2,2),(0.,1.),(0.,0.03),
 .UNSPECIFIED.);
#805=B_SPLINE_SURFACE_WITH_KNOTS('',2,1,((#82196,#82197),(#82198,#82199),
(#82200,#82201)),.UNSPECIFIED.,.F.,.F.,.F.,(3,3),(2,2),(0.,1.),(0.,0.03),
 .UNSPECIFIED.);
#806=B_SPLINE_SURFACE_WITH_KNOTS('',2,1,((#82211,#82212),(#82213,#82214),
(#82215,#82216)),.UNSPECIFIED.,.F.,.F.,.F.,(3,3),(2,2),(0.,1.),(0.,0.03),
 .UNSPECIFIED.);
#807=B_SPLINE_SURFACE_WITH_KNOTS('',2,1,((#82226,#82227),(#82228,#82229),
(#82230,#82231)),.UNSPECIFIED.,.F.,.F.,.F.,(3,3),(2,2),(0.,1.),(0.,0.03),
 .UNSPECIFIED.);
#808=B_SPLINE_SURFACE_WITH_KNOTS('',2,1,((#82241,#82242),(#82243,#82244),
(#82245,#82246)),.UNSPECIFIED.,.F.,.F.,.F.,(3,3),(2,2),(0.,1.),(0.,0.03),
 .UNSPECIFIED.);
#809=B_SPLINE_SURFACE_WITH_KNOTS('',2,1,((#82256,#82257),(#82258,#82259),
(#82260,#82261)),.UNSPECIFIED.,.F.,.F.,.F.,(3,3),(2,2),(0.,1.),(0.,0.03),
 .UNSPECIFIED.);
#810=B_SPLINE_SURFACE_WITH_KNOTS('',2,1,((#82269,#82270),(#82271,#82272),
(#82273,#82274)),.UNSPECIFIED.,.F.,.F.,.F.,(3,3),(2,2),(0.,1.),(0.,0.03),
 .UNSPECIFIED.);
#811=B_SPLINE_SURFACE_WITH_KNOTS('',2,1,((#82287,#82288),(#82289,#82290),
(#82291,#82292)),.UNSPECIFIED.,.F.,.F.,.F.,(3,3),(2,2),(0.,1.),(0.,0.03),
 .UNSPECIFIED.);
#812=B_SPLINE_SURFACE_WITH_KNOTS('',2,1,((#82308,#82309),(#82310,#82311),
(#82312,#82313)),.UNSPECIFIED.,.F.,.F.,.F.,(3,3),(2,2),(0.,1.),(0.,0.03),
 .UNSPECIFIED.);
#813=B_SPLINE_SURFACE_WITH_KNOTS('',2,1,((#82323,#82324),(#82325,#82326),
(#82327,#82328)),.UNSPECIFIED.,.F.,.F.,.F.,(3,3),(2,2),(0.,1.),(0.,0.03),
 .UNSPECIFIED.);
#814=B_SPLINE_SURFACE_WITH_KNOTS('',2,1,((#82385,#82386),(#82387,#82388),
(#82389,#82390)),.UNSPECIFIED.,.F.,.F.,.F.,(3,3),(2,2),(0.,1.),(0.,0.03),
 .UNSPECIFIED.);
#815=B_SPLINE_SURFACE_WITH_KNOTS('',2,1,((#82403,#82404),(#82405,#82406),
(#82407,#82408)),.UNSPECIFIED.,.F.,.F.,.F.,(3,3),(2,2),(0.,1.),(0.,0.03),
 .UNSPECIFIED.);
#816=B_SPLINE_SURFACE_WITH_KNOTS('',2,1,((#82418,#82419),(#82420,#82421),
(#82422,#82423)),.UNSPECIFIED.,.F.,.F.,.F.,(3,3),(2,2),(0.,1.),(0.,0.03),
 .UNSPECIFIED.);
#817=B_SPLINE_SURFACE_WITH_KNOTS('',2,1,((#82433,#82434),(#82435,#82436),
(#82437,#82438)),.UNSPECIFIED.,.F.,.F.,.F.,(3,3),(2,2),(0.,1.),(0.,0.03),
 .UNSPECIFIED.);
#818=B_SPLINE_SURFACE_WITH_KNOTS('',2,1,((#82448,#82449),(#82450,#82451),
(#82452,#82453)),.UNSPECIFIED.,.F.,.F.,.F.,(3,3),(2,2),(0.,1.),(0.,0.03),
 .UNSPECIFIED.);
#819=B_SPLINE_SURFACE_WITH_KNOTS('',2,1,((#82499,#82500),(#82501,#82502),
(#82503,#82504)),.UNSPECIFIED.,.F.,.F.,.F.,(3,3),(2,2),(0.,1.),(0.,0.03),
 .UNSPECIFIED.);
#820=B_SPLINE_SURFACE_WITH_KNOTS('',2,1,((#82514,#82515),(#82516,#82517),
(#82518,#82519)),.UNSPECIFIED.,.F.,.F.,.F.,(3,3),(2,2),(0.,1.),(0.,0.03),
 .UNSPECIFIED.);
#821=B_SPLINE_SURFACE_WITH_KNOTS('',2,1,((#82529,#82530),(#82531,#82532),
(#82533,#82534)),.UNSPECIFIED.,.F.,.F.,.F.,(3,3),(2,2),(0.,1.),(0.,0.03),
 .UNSPECIFIED.);
#822=B_SPLINE_SURFACE_WITH_KNOTS('',2,1,((#82544,#82545),(#82546,#82547),
(#82548,#82549)),.UNSPECIFIED.,.F.,.F.,.F.,(3,3),(2,2),(0.,1.),(0.,0.03),
 .UNSPECIFIED.);
#823=B_SPLINE_SURFACE_WITH_KNOTS('',2,1,((#82559,#82560),(#82561,#82562),
(#82563,#82564)),.UNSPECIFIED.,.F.,.F.,.F.,(3,3),(2,2),(0.,1.),(0.,0.03),
 .UNSPECIFIED.);
#824=B_SPLINE_SURFACE_WITH_KNOTS('',2,1,((#82574,#82575),(#82576,#82577),
(#82578,#82579)),.UNSPECIFIED.,.F.,.F.,.F.,(3,3),(2,2),(0.,1.),(0.,0.03),
 .UNSPECIFIED.);
#825=B_SPLINE_SURFACE_WITH_KNOTS('',2,1,((#82589,#82590),(#82591,#82592),
(#82593,#82594)),.UNSPECIFIED.,.F.,.F.,.F.,(3,3),(2,2),(0.,1.),(0.,0.03),
 .UNSPECIFIED.);
#826=B_SPLINE_SURFACE_WITH_KNOTS('',2,1,((#82604,#82605),(#82606,#82607),
(#82608,#82609)),.UNSPECIFIED.,.F.,.F.,.F.,(3,3),(2,2),(0.,1.),(0.,0.03),
 .UNSPECIFIED.);
#827=B_SPLINE_SURFACE_WITH_KNOTS('',2,1,((#82625,#82626),(#82627,#82628),
(#82629,#82630)),.UNSPECIFIED.,.F.,.F.,.F.,(3,3),(2,2),(0.,1.),(0.,0.03),
 .UNSPECIFIED.);
#828=B_SPLINE_SURFACE_WITH_KNOTS('',2,1,((#82640,#82641),(#82642,#82643),
(#82644,#82645)),.UNSPECIFIED.,.F.,.F.,.F.,(3,3),(2,2),(0.,1.),(0.,0.03),
 .UNSPECIFIED.);
#829=B_SPLINE_SURFACE_WITH_KNOTS('',2,1,((#82653,#82654),(#82655,#82656),
(#82657,#82658)),.UNSPECIFIED.,.F.,.F.,.F.,(3,3),(2,2),(0.,1.),(0.,0.03),
 .UNSPECIFIED.);
#830=B_SPLINE_SURFACE_WITH_KNOTS('',2,1,((#82671,#82672),(#82673,#82674),
(#82675,#82676)),.UNSPECIFIED.,.F.,.F.,.F.,(3,3),(2,2),(0.,1.),(0.,0.03),
 .UNSPECIFIED.);
#831=B_SPLINE_SURFACE_WITH_KNOTS('',2,1,((#82686,#82687),(#82688,#82689),
(#82690,#82691)),.UNSPECIFIED.,.F.,.F.,.F.,(3,3),(2,2),(0.,1.),(0.,0.03),
 .UNSPECIFIED.);
#832=B_SPLINE_SURFACE_WITH_KNOTS('',2,1,((#82701,#82702),(#82703,#82704),
(#82705,#82706)),.UNSPECIFIED.,.F.,.F.,.F.,(3,3),(2,2),(0.,1.),(0.,0.03),
 .UNSPECIFIED.);
#833=B_SPLINE_SURFACE_WITH_KNOTS('',2,1,((#82716,#82717),(#82718,#82719),
(#82720,#82721)),.UNSPECIFIED.,.F.,.F.,.F.,(3,3),(2,2),(0.,1.),(0.,0.03),
 .UNSPECIFIED.);
#834=B_SPLINE_SURFACE_WITH_KNOTS('',2,1,((#82731,#82732),(#82733,#82734),
(#82735,#82736)),.UNSPECIFIED.,.F.,.F.,.F.,(3,3),(2,2),(0.,1.),(0.,0.03),
 .UNSPECIFIED.);
#835=B_SPLINE_SURFACE_WITH_KNOTS('',2,1,((#82746,#82747),(#82748,#82749),
(#82750,#82751)),.UNSPECIFIED.,.F.,.F.,.F.,(3,3),(2,2),(0.,1.),(0.,0.03),
 .UNSPECIFIED.);
#836=B_SPLINE_SURFACE_WITH_KNOTS('',2,1,((#82761,#82762),(#82763,#82764),
(#82765,#82766)),.UNSPECIFIED.,.F.,.F.,.F.,(3,3),(2,2),(0.,1.),(0.,0.03),
 .UNSPECIFIED.);
#837=B_SPLINE_SURFACE_WITH_KNOTS('',2,1,((#82776,#82777),(#82778,#82779),
(#82780,#82781)),.UNSPECIFIED.,.F.,.F.,.F.,(3,3),(2,2),(0.,1.),(0.,0.03),
 .UNSPECIFIED.);
#838=B_SPLINE_SURFACE_WITH_KNOTS('',2,1,((#82791,#82792),(#82793,#82794),
(#82795,#82796)),.UNSPECIFIED.,.F.,.F.,.F.,(3,3),(2,2),(0.,1.),(0.,0.03),
 .UNSPECIFIED.);
#839=B_SPLINE_SURFACE_WITH_KNOTS('',2,1,((#82806,#82807),(#82808,#82809),
(#82810,#82811)),.UNSPECIFIED.,.F.,.F.,.F.,(3,3),(2,2),(0.,1.),(0.,0.03),
 .UNSPECIFIED.);
#840=B_SPLINE_SURFACE_WITH_KNOTS('',2,1,((#82819,#82820),(#82821,#82822),
(#82823,#82824)),.UNSPECIFIED.,.F.,.F.,.F.,(3,3),(2,2),(0.,1.),(0.,0.03),
 .UNSPECIFIED.);
#841=B_SPLINE_SURFACE_WITH_KNOTS('',2,1,((#82837,#82838),(#82839,#82840),
(#82841,#82842)),.UNSPECIFIED.,.F.,.F.,.F.,(3,3),(2,2),(0.,1.),(0.,0.03),
 .UNSPECIFIED.);
#842=B_SPLINE_SURFACE_WITH_KNOTS('',2,1,((#82852,#82853),(#82854,#82855),
(#82856,#82857)),.UNSPECIFIED.,.F.,.F.,.F.,(3,3),(2,2),(0.,1.),(0.,0.03),
 .UNSPECIFIED.);
#843=B_SPLINE_SURFACE_WITH_KNOTS('',2,1,((#82867,#82868),(#82869,#82870),
(#82871,#82872)),.UNSPECIFIED.,.F.,.F.,.F.,(3,3),(2,2),(0.,1.),(0.,0.03),
 .UNSPECIFIED.);
#844=B_SPLINE_SURFACE_WITH_KNOTS('',2,1,((#82882,#82883),(#82884,#82885),
(#82886,#82887)),.UNSPECIFIED.,.F.,.F.,.F.,(3,3),(2,2),(0.,1.),(0.,0.03),
 .UNSPECIFIED.);
#845=B_SPLINE_SURFACE_WITH_KNOTS('',2,1,((#82897,#82898),(#82899,#82900),
(#82901,#82902)),.UNSPECIFIED.,.F.,.F.,.F.,(3,3),(2,2),(0.,1.),(0.,0.03),
 .UNSPECIFIED.);
#846=B_SPLINE_SURFACE_WITH_KNOTS('',2,1,((#82912,#82913),(#82914,#82915),
(#82916,#82917)),.UNSPECIFIED.,.F.,.F.,.F.,(3,3),(2,2),(0.,1.),(0.,0.03),
 .UNSPECIFIED.);
#847=B_SPLINE_SURFACE_WITH_KNOTS('',2,1,((#82927,#82928),(#82929,#82930),
(#82931,#82932)),.UNSPECIFIED.,.F.,.F.,.F.,(3,3),(2,2),(0.,1.),(0.,0.03),
 .UNSPECIFIED.);
#848=B_SPLINE_SURFACE_WITH_KNOTS('',2,1,((#82942,#82943),(#82944,#82945),
(#82946,#82947)),.UNSPECIFIED.,.F.,.F.,.F.,(3,3),(2,2),(0.,1.),(0.,0.03),
 .UNSPECIFIED.);
#849=B_SPLINE_SURFACE_WITH_KNOTS('',2,1,((#82957,#82958),(#82959,#82960),
(#82961,#82962)),.UNSPECIFIED.,.F.,.F.,.F.,(3,3),(2,2),(0.,1.),(0.,0.03),
 .UNSPECIFIED.);
#850=B_SPLINE_SURFACE_WITH_KNOTS('',2,1,((#82972,#82973),(#82974,#82975),
(#82976,#82977)),.UNSPECIFIED.,.F.,.F.,.F.,(3,3),(2,2),(0.,1.),(0.,0.03),
 .UNSPECIFIED.);
#851=B_SPLINE_SURFACE_WITH_KNOTS('',2,1,((#82993,#82994),(#82995,#82996),
(#82997,#82998)),.UNSPECIFIED.,.F.,.F.,.F.,(3,3),(2,2),(0.,1.),(0.,0.03),
 .UNSPECIFIED.);
#852=B_SPLINE_SURFACE_WITH_KNOTS('',2,1,((#83008,#83009),(#83010,#83011),
(#83012,#83013)),.UNSPECIFIED.,.F.,.F.,.F.,(3,3),(2,2),(0.,1.),(0.,0.03),
 .UNSPECIFIED.);
#853=B_SPLINE_SURFACE_WITH_KNOTS('',2,1,((#83023,#83024),(#83025,#83026),
(#83027,#83028)),.UNSPECIFIED.,.F.,.F.,.F.,(3,3),(2,2),(0.,1.),(0.,0.03),
 .UNSPECIFIED.);
#854=B_SPLINE_SURFACE_WITH_KNOTS('',2,1,((#83134,#83135),(#83136,#83137),
(#83138,#83139)),.UNSPECIFIED.,.F.,.F.,.F.,(3,3),(2,2),(0.,1.),(0.,0.03),
 .UNSPECIFIED.);
#855=B_SPLINE_SURFACE_WITH_KNOTS('',2,1,((#83152,#83153),(#83154,#83155),
(#83156,#83157)),.UNSPECIFIED.,.F.,.F.,.F.,(3,3),(2,2),(0.,1.),(0.,0.03),
 .UNSPECIFIED.);
#856=B_SPLINE_SURFACE_WITH_KNOTS('',2,1,((#83167,#83168),(#83169,#83170),
(#83171,#83172)),.UNSPECIFIED.,.F.,.F.,.F.,(3,3),(2,2),(0.,1.),(0.,0.03),
 .UNSPECIFIED.);
#857=B_SPLINE_SURFACE_WITH_KNOTS('',2,1,((#83182,#83183),(#83184,#83185),
(#83186,#83187)),.UNSPECIFIED.,.F.,.F.,.F.,(3,3),(2,2),(0.,1.),(0.,0.03),
 .UNSPECIFIED.);
#858=B_SPLINE_SURFACE_WITH_KNOTS('',2,1,((#83197,#83198),(#83199,#83200),
(#83201,#83202)),.UNSPECIFIED.,.F.,.F.,.F.,(3,3),(2,2),(0.,1.),(0.,0.03),
 .UNSPECIFIED.);
#859=B_SPLINE_SURFACE_WITH_KNOTS('',2,1,((#83212,#83213),(#83214,#83215),
(#83216,#83217)),.UNSPECIFIED.,.F.,.F.,.F.,(3,3),(2,2),(0.,1.),(0.,0.03),
 .UNSPECIFIED.);
#860=B_SPLINE_SURFACE_WITH_KNOTS('',2,1,((#83227,#83228),(#83229,#83230),
(#83231,#83232)),.UNSPECIFIED.,.F.,.F.,.F.,(3,3),(2,2),(0.,1.),(0.,0.03),
 .UNSPECIFIED.);
#861=B_SPLINE_SURFACE_WITH_KNOTS('',2,1,((#83242,#83243),(#83244,#83245),
(#83246,#83247)),.UNSPECIFIED.,.F.,.F.,.F.,(3,3),(2,2),(0.,1.),(0.,0.03),
 .UNSPECIFIED.);
#862=B_SPLINE_SURFACE_WITH_KNOTS('',2,1,((#83257,#83258),(#83259,#83260),
(#83261,#83262)),.UNSPECIFIED.,.F.,.F.,.F.,(3,3),(2,2),(0.,1.),(0.,0.03),
 .UNSPECIFIED.);
#863=B_SPLINE_SURFACE_WITH_KNOTS('',2,1,((#83272,#83273),(#83274,#83275),
(#83276,#83277)),.UNSPECIFIED.,.F.,.F.,.F.,(3,3),(2,2),(0.,1.),(0.,0.03),
 .UNSPECIFIED.);
#864=B_SPLINE_SURFACE_WITH_KNOTS('',2,1,((#83287,#83288),(#83289,#83290),
(#83291,#83292)),.UNSPECIFIED.,.F.,.F.,.F.,(3,3),(2,2),(0.,1.),(0.,0.03),
 .UNSPECIFIED.);
#865=B_SPLINE_SURFACE_WITH_KNOTS('',2,1,((#83410,#83411),(#83412,#83413),
(#83414,#83415)),.UNSPECIFIED.,.F.,.F.,.F.,(3,3),(2,2),(0.,1.),(0.,0.03),
 .UNSPECIFIED.);
#866=B_SPLINE_SURFACE_WITH_KNOTS('',2,1,((#83428,#83429),(#83430,#83431),
(#83432,#83433)),.UNSPECIFIED.,.F.,.F.,.F.,(3,3),(2,2),(0.,1.),(0.,0.03),
 .UNSPECIFIED.);
#867=B_SPLINE_SURFACE_WITH_KNOTS('',2,1,((#83443,#83444),(#83445,#83446),
(#83447,#83448)),.UNSPECIFIED.,.F.,.F.,.F.,(3,3),(2,2),(0.,1.),(0.,0.03),
 .UNSPECIFIED.);
#868=B_SPLINE_SURFACE_WITH_KNOTS('',2,1,((#83458,#83459),(#83460,#83461),
(#83462,#83463)),.UNSPECIFIED.,.F.,.F.,.F.,(3,3),(2,2),(0.,1.),(0.,0.03),
 .UNSPECIFIED.);
#869=B_SPLINE_SURFACE_WITH_KNOTS('',2,1,((#83473,#83474),(#83475,#83476),
(#83477,#83478)),.UNSPECIFIED.,.F.,.F.,.F.,(3,3),(2,2),(0.,1.),(0.,0.03),
 .UNSPECIFIED.);
#870=B_SPLINE_SURFACE_WITH_KNOTS('',2,1,((#83488,#83489),(#83490,#83491),
(#83492,#83493)),.UNSPECIFIED.,.F.,.F.,.F.,(3,3),(2,2),(0.,1.),(0.,0.03),
 .UNSPECIFIED.);
#871=B_SPLINE_SURFACE_WITH_KNOTS('',2,1,((#83503,#83504),(#83505,#83506),
(#83507,#83508)),.UNSPECIFIED.,.F.,.F.,.F.,(3,3),(2,2),(0.,1.),(0.,0.03),
 .UNSPECIFIED.);
#872=B_SPLINE_SURFACE_WITH_KNOTS('',2,1,((#83518,#83519),(#83520,#83521),
(#83522,#83523)),.UNSPECIFIED.,.F.,.F.,.F.,(3,3),(2,2),(0.,1.),(0.,0.03),
 .UNSPECIFIED.);
#873=B_SPLINE_SURFACE_WITH_KNOTS('',2,1,((#83551,#83552),(#83553,#83554),
(#83555,#83556)),.UNSPECIFIED.,.F.,.F.,.F.,(3,3),(2,2),(0.,1.),(0.,0.03),
 .UNSPECIFIED.);
#874=B_SPLINE_SURFACE_WITH_KNOTS('',2,1,((#83573,#83574),(#83575,#83576),
(#83577,#83578)),.UNSPECIFIED.,.F.,.F.,.F.,(3,3),(2,2),(0.,1.),(0.,0.03),
 .UNSPECIFIED.);
#875=B_SPLINE_SURFACE_WITH_KNOTS('',2,1,((#83588,#83589),(#83590,#83591),
(#83592,#83593)),.UNSPECIFIED.,.F.,.F.,.F.,(3,3),(2,2),(0.,1.),(0.,0.03),
 .UNSPECIFIED.);
#876=B_SPLINE_SURFACE_WITH_KNOTS('',2,1,((#83603,#83604),(#83605,#83606),
(#83607,#83608)),.UNSPECIFIED.,.F.,.F.,.F.,(3,3),(2,2),(0.,1.),(0.,0.03),
 .UNSPECIFIED.);
#877=B_SPLINE_SURFACE_WITH_KNOTS('',2,1,((#83618,#83619),(#83620,#83621),
(#83622,#83623)),.UNSPECIFIED.,.F.,.F.,.F.,(3,3),(2,2),(0.,1.),(0.,0.03),
 .UNSPECIFIED.);
#878=B_SPLINE_SURFACE_WITH_KNOTS('',2,1,((#83651,#83652),(#83653,#83654),
(#83655,#83656)),.UNSPECIFIED.,.F.,.F.,.F.,(3,3),(2,2),(0.,1.),(0.,0.03),
 .UNSPECIFIED.);
#879=B_SPLINE_SURFACE_WITH_KNOTS('',2,1,((#83666,#83667),(#83668,#83669),
(#83670,#83671)),.UNSPECIFIED.,.F.,.F.,.F.,(3,3),(2,2),(0.,1.),(0.,0.03),
 .UNSPECIFIED.);
#880=B_SPLINE_SURFACE_WITH_KNOTS('',2,1,((#83681,#83682),(#83683,#83684),
(#83685,#83686)),.UNSPECIFIED.,.F.,.F.,.F.,(3,3),(2,2),(0.,1.),(0.,0.03),
 .UNSPECIFIED.);
#881=B_SPLINE_SURFACE_WITH_KNOTS('',2,1,((#83696,#83697),(#83698,#83699),
(#83700,#83701)),.UNSPECIFIED.,.F.,.F.,.F.,(3,3),(2,2),(0.,1.),(0.,0.03),
 .UNSPECIFIED.);
#882=B_SPLINE_SURFACE_WITH_KNOTS('',2,1,((#83711,#83712),(#83713,#83714),
(#83715,#83716)),.UNSPECIFIED.,.F.,.F.,.F.,(3,3),(2,2),(0.,1.),(0.,0.03),
 .UNSPECIFIED.);
#883=B_SPLINE_SURFACE_WITH_KNOTS('',2,1,((#83726,#83727),(#83728,#83729),
(#83730,#83731)),.UNSPECIFIED.,.F.,.F.,.F.,(3,3),(2,2),(0.,1.),(0.,0.03),
 .UNSPECIFIED.);
#884=B_SPLINE_SURFACE_WITH_KNOTS('',2,1,((#83741,#83742),(#83743,#83744),
(#83745,#83746)),.UNSPECIFIED.,.F.,.F.,.F.,(3,3),(2,2),(0.,1.),(0.,0.03),
 .UNSPECIFIED.);
#894=SHAPE_REPRESENTATION_RELATIONSHIP('SRR','None',#94374,#908);
#908=ADVANCED_BREP_SHAPE_REPRESENTATION('',(#936),#94290);
#922=STYLED_ITEM('',(#94560),#936);
#936=MANIFOLD_SOLID_BREP('Body1',#51021);
#989=FACE_BOUND('',#18062,.T.);
#990=FACE_BOUND('',#18063,.T.);
#991=FACE_BOUND('',#18064,.T.);
#992=FACE_BOUND('',#18065,.T.);
#993=FACE_BOUND('',#18066,.T.);
#994=FACE_BOUND('',#18067,.T.);
#995=FACE_BOUND('',#18068,.T.);
#996=FACE_BOUND('',#18069,.T.);
#997=FACE_BOUND('',#18070,.T.);
#998=FACE_BOUND('',#18071,.T.);
#999=FACE_BOUND('',#18072,.T.);
#1000=FACE_BOUND('',#18073,.T.);
#1001=FACE_BOUND('',#18074,.T.);
#1002=FACE_BOUND('',#18075,.T.);
#1003=FACE_BOUND('',#18076,.T.);
#1004=FACE_BOUND('',#18077,.T.);
#1005=FACE_BOUND('',#18078,.T.);
#1006=FACE_BOUND('',#18079,.T.);
#1007=FACE_BOUND('',#18080,.T.);
#1008=FACE_BOUND('',#18081,.T.);
#1009=FACE_BOUND('',#18082,.T.);
#1010=FACE_BOUND('',#18083,.T.);
#1011=FACE_BOUND('',#18084,.T.);
#1012=FACE_BOUND('',#18088,.T.);
#1013=FACE_BOUND('',#18089,.T.);
#1014=FACE_BOUND('',#18090,.T.);
#1015=FACE_BOUND('',#18091,.T.);
#1016=FACE_BOUND('',#18092,.T.);
#1017=FACE_BOUND('',#18093,.T.);
#1018=FACE_BOUND('',#18094,.T.);
#1019=FACE_BOUND('',#18095,.T.);
#1020=FACE_BOUND('',#18096,.T.);
#1021=FACE_BOUND('',#18097,.T.);
#1022=FACE_BOUND('',#18098,.T.);
#1023=FACE_BOUND('',#18099,.T.);
#1024=FACE_BOUND('',#18102,.T.);
#1025=FACE_BOUND('',#18103,.T.);
#1026=FACE_BOUND('',#18104,.T.);
#1027=FACE_BOUND('',#18105,.T.);
#1140=CYLINDRICAL_SURFACE('',#54371,4.5);
#1141=CYLINDRICAL_SURFACE('',#54400,4.5);
#1142=CYLINDRICAL_SURFACE('',#54405,4.5);
#1143=CYLINDRICAL_SURFACE('',#54410,4.5);
#1144=CYLINDRICAL_SURFACE('',#54415,3.);
#1145=CYLINDRICAL_SURFACE('',#54418,3.);
#1146=CYLINDRICAL_SURFACE('',#54423,3.05);
#1147=CYLINDRICAL_SURFACE('',#54428,3.05);
#1148=CYLINDRICAL_SURFACE('',#54433,3.05);
#1149=CYLINDRICAL_SURFACE('',#54438,3.05);
#1150=CYLINDRICAL_SURFACE('',#54439,20.025);
#1151=CYLINDRICAL_SURFACE('',#54455,10.);
#1152=CYLINDRICAL_SURFACE('',#54458,10.);
#1153=CYLINDRICAL_SURFACE('',#54470,10.);
#1154=CYLINDRICAL_SURFACE('',#54472,10.);
#5357=LINE('',#80530,#9885);
#5358=LINE('',#80532,#9886);
#5359=LINE('',#80534,#9887);
#5360=LINE('',#80535,#9888);
#5361=LINE('',#80538,#9889);
#5362=LINE('',#80540,#9890);
#5363=LINE('',#80541,#9891);
#5364=LINE('',#80544,#9892);
#5365=LINE('',#80546,#9893);
#5366=LINE('',#80547,#9894);
#5367=LINE('',#80550,#9895);
#5368=LINE('',#80552,#9896);
#5369=LINE('',#80553,#9897);
#5370=LINE('',#80556,#9898);
#5371=LINE('',#80558,#9899);
#5372=LINE('',#80559,#9900);
#5373=LINE('',#80562,#9901);
#5374=LINE('',#80564,#9902);
#5375=LINE('',#80565,#9903);
#5376=LINE('',#80568,#9904);
#5377=LINE('',#80570,#9905);
#5378=LINE('',#80571,#9906);
#5379=LINE('',#80574,#9907);
#5380=LINE('',#80576,#9908);
#5381=LINE('',#80577,#9909);
#5382=LINE('',#80580,#9910);
#5383=LINE('',#80582,#9911);
#5384=LINE('',#80583,#9912);
#5385=LINE('',#80586,#9913);
#5386=LINE('',#80588,#9914);
#5387=LINE('',#80589,#9915);
#5388=LINE('',#80592,#9916);
#5389=LINE('',#80594,#9917);
#5390=LINE('',#80595,#9918);
#5391=LINE('',#80597,#9919);
#5392=LINE('',#80598,#9920);
#5393=LINE('',#80603,#9921);
#5394=LINE('',#80605,#9922);
#5395=LINE('',#80607,#9923);
#5396=LINE('',#80608,#9924);
#5397=LINE('',#80611,#9925);
#5398=LINE('',#80613,#9926);
#5399=LINE('',#80614,#9927);
#5400=LINE('',#80617,#9928);
#5401=LINE('',#80619,#9929);
#5402=LINE('',#80620,#9930);
#5403=LINE('',#80622,#9931);
#5404=LINE('',#80623,#9932);
#5405=LINE('',#80637,#9933);
#5406=LINE('',#80642,#9934);
#5407=LINE('',#80654,#9935);
#5408=LINE('',#80669,#9936);
#5409=LINE('',#80684,#9937);
#5410=LINE('',#80699,#9938);
#5411=LINE('',#80714,#9939);
#5412=LINE('',#80729,#9940);
#5413=LINE('',#80744,#9941);
#5414=LINE('',#80759,#9942);
#5415=LINE('',#80774,#9943);
#5416=LINE('',#80789,#9944);
#5417=LINE('',#80804,#9945);
#5418=LINE('',#80819,#9946);
#5419=LINE('',#80825,#9947);
#5420=LINE('',#80827,#9948);
#5421=LINE('',#80828,#9949);
#5422=LINE('',#80840,#9950);
#5423=LINE('',#80855,#9951);
#5424=LINE('',#80870,#9952);
#5425=LINE('',#80885,#9953);
#5426=LINE('',#80900,#9954);
#5427=LINE('',#80915,#9955);
#5428=LINE('',#80930,#9956);
#5429=LINE('',#80945,#9957);
#5430=LINE('',#80960,#9958);
#5431=LINE('',#80975,#9959);
#5432=LINE('',#80990,#9960);
#5433=LINE('',#81005,#9961);
#5434=LINE('',#81020,#9962);
#5435=LINE('',#81035,#9963);
#5436=LINE('',#81050,#9964);
#5437=LINE('',#81065,#9965);
#5438=LINE('',#81080,#9966);
#5439=LINE('',#81095,#9967);
#5440=LINE('',#81101,#9968);
#5441=LINE('',#81103,#9969);
#5442=LINE('',#81104,#9970);
#5443=LINE('',#81116,#9971);
#5444=LINE('',#81145,#9972);
#5445=LINE('',#81150,#9973);
#5446=LINE('',#81162,#9974);
#5447=LINE('',#81177,#9975);
#5448=LINE('',#81192,#9976);
#5449=LINE('',#81207,#9977);
#5450=LINE('',#81222,#9978);
#5451=LINE('',#81237,#9979);
#5452=LINE('',#81252,#9980);
#5453=LINE('',#81258,#9981);
#5454=LINE('',#81260,#9982);
#5455=LINE('',#81261,#9983);
#5456=LINE('',#81273,#9984);
#5457=LINE('',#81288,#9985);
#5458=LINE('',#81303,#9986);
#5459=LINE('',#81318,#9987);
#5460=LINE('',#81333,#9988);
#5461=LINE('',#81348,#9989);
#5462=LINE('',#81363,#9990);
#5463=LINE('',#81378,#9991);
#5464=LINE('',#81393,#9992);
#5465=LINE('',#81408,#9993);
#5466=LINE('',#81414,#9994);
#5467=LINE('',#81416,#9995);
#5468=LINE('',#81417,#9996);
#5469=LINE('',#81429,#9997);
#5470=LINE('',#81449,#9998);
#5471=LINE('',#81451,#9999);
#5472=LINE('',#81453,#10000);
#5473=LINE('',#81454,#10001);
#5474=LINE('',#81457,#10002);
#5475=LINE('',#81459,#10003);
#5476=LINE('',#81460,#10004);
#5477=LINE('',#81463,#10005);
#5478=LINE('',#81465,#10006);
#5479=LINE('',#81466,#10007);
#5480=LINE('',#81469,#10008);
#5481=LINE('',#81471,#10009);
#5482=LINE('',#81472,#10010);
#5483=LINE('',#81475,#10011);
#5484=LINE('',#81477,#10012);
#5485=LINE('',#81478,#10013);
#5486=LINE('',#81480,#10014);
#5487=LINE('',#81481,#10015);
#5488=LINE('',#81486,#10016);
#5489=LINE('',#81488,#10017);
#5490=LINE('',#81490,#10018);
#5491=LINE('',#81491,#10019);
#5492=LINE('',#81494,#10020);
#5493=LINE('',#81496,#10021);
#5494=LINE('',#81497,#10022);
#5495=LINE('',#81500,#10023);
#5496=LINE('',#81502,#10024);
#5497=LINE('',#81503,#10025);
#5498=LINE('',#81506,#10026);
#5499=LINE('',#81508,#10027);
#5500=LINE('',#81509,#10028);
#5501=LINE('',#81512,#10029);
#5502=LINE('',#81514,#10030);
#5503=LINE('',#81515,#10031);
#5504=LINE('',#81518,#10032);
#5505=LINE('',#81520,#10033);
#5506=LINE('',#81521,#10034);
#5507=LINE('',#81524,#10035);
#5508=LINE('',#81526,#10036);
#5509=LINE('',#81527,#10037);
#5510=LINE('',#81529,#10038);
#5511=LINE('',#81530,#10039);
#5512=LINE('',#81544,#10040);
#5513=LINE('',#81549,#10041);
#5514=LINE('',#81561,#10042);
#5515=LINE('',#81576,#10043);
#5516=LINE('',#81591,#10044);
#5517=LINE('',#81597,#10045);
#5518=LINE('',#81599,#10046);
#5519=LINE('',#81600,#10047);
#5520=LINE('',#81603,#10048);
#5521=LINE('',#81605,#10049);
#5522=LINE('',#81606,#10050);
#5523=LINE('',#81609,#10051);
#5524=LINE('',#81611,#10052);
#5525=LINE('',#81612,#10053);
#5526=LINE('',#81624,#10054);
#5527=LINE('',#81639,#10055);
#5528=LINE('',#81654,#10056);
#5529=LINE('',#81669,#10057);
#5530=LINE('',#81684,#10058);
#5531=LINE('',#81699,#10059);
#5532=LINE('',#81705,#10060);
#5533=LINE('',#81707,#10061);
#5534=LINE('',#81708,#10062);
#5535=LINE('',#81711,#10063);
#5536=LINE('',#81713,#10064);
#5537=LINE('',#81714,#10065);
#5538=LINE('',#81717,#10066);
#5539=LINE('',#81719,#10067);
#5540=LINE('',#81720,#10068);
#5541=LINE('',#81737,#10069);
#5542=LINE('',#81739,#10070);
#5543=LINE('',#81741,#10071);
#5544=LINE('',#81742,#10072);
#5545=LINE('',#81754,#10073);
#5546=LINE('',#81769,#10074);
#5547=LINE('',#81784,#10075);
#5548=LINE('',#81799,#10076);
#5549=LINE('',#81805,#10077);
#5550=LINE('',#81807,#10078);
#5551=LINE('',#81808,#10079);
#5552=LINE('',#81811,#10080);
#5553=LINE('',#81813,#10081);
#5554=LINE('',#81814,#10082);
#5555=LINE('',#81817,#10083);
#5556=LINE('',#81819,#10084);
#5557=LINE('',#81820,#10085);
#5558=LINE('',#81832,#10086);
#5559=LINE('',#81847,#10087);
#5560=LINE('',#81862,#10088);
#5561=LINE('',#81877,#10089);
#5562=LINE('',#81892,#10090);
#5563=LINE('',#81907,#10091);
#5564=LINE('',#81922,#10092);
#5565=LINE('',#81928,#10093);
#5566=LINE('',#81930,#10094);
#5567=LINE('',#81931,#10095);
#5568=LINE('',#81934,#10096);
#5569=LINE('',#81936,#10097);
#5570=LINE('',#81937,#10098);
#5571=LINE('',#81940,#10099);
#5572=LINE('',#81942,#10100);
#5573=LINE('',#81943,#10101);
#5574=LINE('',#81945,#10102);
#5575=LINE('',#81946,#10103);
#5576=LINE('',#81951,#10104);
#5577=LINE('',#81953,#10105);
#5578=LINE('',#81955,#10106);
#5579=LINE('',#81956,#10107);
#5580=LINE('',#81959,#10108);
#5581=LINE('',#81961,#10109);
#5582=LINE('',#81962,#10110);
#5583=LINE('',#81965,#10111);
#5584=LINE('',#81967,#10112);
#5585=LINE('',#81968,#10113);
#5586=LINE('',#81971,#10114);
#5587=LINE('',#81973,#10115);
#5588=LINE('',#81974,#10116);
#5589=LINE('',#81977,#10117);
#5590=LINE('',#81979,#10118);
#5591=LINE('',#81980,#10119);
#5592=LINE('',#81983,#10120);
#5593=LINE('',#81985,#10121);
#5594=LINE('',#81986,#10122);
#5595=LINE('',#81989,#10123);
#5596=LINE('',#81991,#10124);
#5597=LINE('',#81992,#10125);
#5598=LINE('',#81994,#10126);
#5599=LINE('',#81995,#10127);
#5600=LINE('',#82009,#10128);
#5601=LINE('',#82014,#10129);
#5602=LINE('',#82026,#10130);
#5603=LINE('',#82032,#10131);
#5604=LINE('',#82034,#10132);
#5605=LINE('',#82035,#10133);
#5606=LINE('',#82047,#10134);
#5607=LINE('',#82062,#10135);
#5608=LINE('',#82068,#10136);
#5609=LINE('',#82070,#10137);
#5610=LINE('',#82071,#10138);
#5611=LINE('',#82074,#10139);
#5612=LINE('',#82076,#10140);
#5613=LINE('',#82077,#10141);
#5614=LINE('',#82080,#10142);
#5615=LINE('',#82082,#10143);
#5616=LINE('',#82083,#10144);
#5617=LINE('',#82085,#10145);
#5618=LINE('',#82086,#10146);
#5619=LINE('',#82100,#10147);
#5620=LINE('',#82105,#10148);
#5621=LINE('',#82117,#10149);
#5622=LINE('',#82132,#10150);
#5623=LINE('',#82147,#10151);
#5624=LINE('',#82162,#10152);
#5625=LINE('',#82177,#10153);
#5626=LINE('',#82192,#10154);
#5627=LINE('',#82207,#10155);
#5628=LINE('',#82222,#10156);
#5629=LINE('',#82237,#10157);
#5630=LINE('',#82252,#10158);
#5631=LINE('',#82281,#10159);
#5632=LINE('',#82286,#10160);
#5633=LINE('',#82298,#10161);
#5634=LINE('',#82304,#10162);
#5635=LINE('',#82306,#10163);
#5636=LINE('',#82307,#10164);
#5637=LINE('',#82319,#10165);
#5638=LINE('',#82334,#10166);
#5639=LINE('',#82340,#10167);
#5640=LINE('',#82342,#10168);
#5641=LINE('',#82343,#10169);
#5642=LINE('',#82346,#10170);
#5643=LINE('',#82348,#10171);
#5644=LINE('',#82349,#10172);
#5645=LINE('',#82352,#10173);
#5646=LINE('',#82354,#10174);
#5647=LINE('',#82355,#10175);
#5648=LINE('',#82357,#10176);
#5649=LINE('',#82358,#10177);
#5650=LINE('',#82363,#10178);
#5651=LINE('',#82365,#10179);
#5652=LINE('',#82367,#10180);
#5653=LINE('',#82368,#10181);
#5654=LINE('',#82371,#10182);
#5655=LINE('',#82373,#10183);
#5656=LINE('',#82374,#10184);
#5657=LINE('',#82377,#10185);
#5658=LINE('',#82379,#10186);
#5659=LINE('',#82380,#10187);
#5660=LINE('',#82382,#10188);
#5661=LINE('',#82383,#10189);
#5662=LINE('',#82397,#10190);
#5663=LINE('',#82402,#10191);
#5664=LINE('',#82414,#10192);
#5665=LINE('',#82429,#10193);
#5666=LINE('',#82444,#10194);
#5667=LINE('',#82459,#10195);
#5668=LINE('',#82465,#10196);
#5669=LINE('',#82467,#10197);
#5670=LINE('',#82468,#10198);
#5671=LINE('',#82471,#10199);
#5672=LINE('',#82473,#10200);
#5673=LINE('',#82474,#10201);
#5674=LINE('',#82477,#10202);
#5675=LINE('',#82479,#10203);
#5676=LINE('',#82480,#10204);
#5677=LINE('',#82483,#10205);
#5678=LINE('',#82485,#10206);
#5679=LINE('',#82486,#10207);
#5680=LINE('',#82489,#10208);
#5681=LINE('',#82491,#10209);
#5682=LINE('',#82492,#10210);
#5683=LINE('',#82495,#10211);
#5684=LINE('',#82497,#10212);
#5685=LINE('',#82498,#10213);
#5686=LINE('',#82510,#10214);
#5687=LINE('',#82525,#10215);
#5688=LINE('',#82540,#10216);
#5689=LINE('',#82555,#10217);
#5690=LINE('',#82570,#10218);
#5691=LINE('',#82585,#10219);
#5692=LINE('',#82600,#10220);
#5693=LINE('',#82615,#10221);
#5694=LINE('',#82621,#10222);
#5695=LINE('',#82623,#10223);
#5696=LINE('',#82624,#10224);
#5697=LINE('',#82636,#10225);
#5698=LINE('',#82665,#10226);
#5699=LINE('',#82670,#10227);
#5700=LINE('',#82682,#10228);
#5701=LINE('',#82697,#10229);
#5702=LINE('',#82712,#10230);
#5703=LINE('',#82727,#10231);
#5704=LINE('',#82742,#10232);
#5705=LINE('',#82757,#10233);
#5706=LINE('',#82772,#10234);
#5707=LINE('',#82787,#10235);
#5708=LINE('',#82802,#10236);
#5709=LINE('',#82831,#10237);
#5710=LINE('',#82836,#10238);
#5711=LINE('',#82848,#10239);
#5712=LINE('',#82863,#10240);
#5713=LINE('',#82878,#10241);
#5714=LINE('',#82893,#10242);
#5715=LINE('',#82908,#10243);
#5716=LINE('',#82923,#10244);
#5717=LINE('',#82938,#10245);
#5718=LINE('',#82953,#10246);
#5719=LINE('',#82968,#10247);
#5720=LINE('',#82983,#10248);
#5721=LINE('',#82989,#10249);
#5722=LINE('',#82991,#10250);
#5723=LINE('',#82992,#10251);
#5724=LINE('',#83004,#10252);
#5725=LINE('',#83019,#10253);
#5726=LINE('',#83039,#10254);
#5727=LINE('',#83041,#10255);
#5728=LINE('',#83043,#10256);
#5729=LINE('',#83044,#10257);
#5730=LINE('',#83047,#10258);
#5731=LINE('',#83049,#10259);
#5732=LINE('',#83050,#10260);
#5733=LINE('',#83053,#10261);
#5734=LINE('',#83055,#10262);
#5735=LINE('',#83056,#10263);
#5736=LINE('',#83059,#10264);
#5737=LINE('',#83061,#10265);
#5738=LINE('',#83062,#10266);
#5739=LINE('',#83065,#10267);
#5740=LINE('',#83067,#10268);
#5741=LINE('',#83068,#10269);
#5742=LINE('',#83071,#10270);
#5743=LINE('',#83073,#10271);
#5744=LINE('',#83074,#10272);
#5745=LINE('',#83077,#10273);
#5746=LINE('',#83079,#10274);
#5747=LINE('',#83080,#10275);
#5748=LINE('',#83083,#10276);
#5749=LINE('',#83085,#10277);
#5750=LINE('',#83086,#10278);
#5751=LINE('',#83089,#10279);
#5752=LINE('',#83091,#10280);
#5753=LINE('',#83092,#10281);
#5754=LINE('',#83095,#10282);
#5755=LINE('',#83097,#10283);
#5756=LINE('',#83098,#10284);
#5757=LINE('',#83101,#10285);
#5758=LINE('',#83103,#10286);
#5759=LINE('',#83104,#10287);
#5760=LINE('',#83106,#10288);
#5761=LINE('',#83107,#10289);
#5762=LINE('',#83112,#10290);
#5763=LINE('',#83114,#10291);
#5764=LINE('',#83116,#10292);
#5765=LINE('',#83117,#10293);
#5766=LINE('',#83120,#10294);
#5767=LINE('',#83122,#10295);
#5768=LINE('',#83123,#10296);
#5769=LINE('',#83126,#10297);
#5770=LINE('',#83128,#10298);
#5771=LINE('',#83129,#10299);
#5772=LINE('',#83131,#10300);
#5773=LINE('',#83132,#10301);
#5774=LINE('',#83146,#10302);
#5775=LINE('',#83151,#10303);
#5776=LINE('',#83163,#10304);
#5777=LINE('',#83178,#10305);
#5778=LINE('',#83193,#10306);
#5779=LINE('',#83208,#10307);
#5780=LINE('',#83223,#10308);
#5781=LINE('',#83238,#10309);
#5782=LINE('',#83253,#10310);
#5783=LINE('',#83268,#10311);
#5784=LINE('',#83283,#10312);
#5785=LINE('',#83303,#10313);
#5786=LINE('',#83305,#10314);
#5787=LINE('',#83307,#10315);
#5788=LINE('',#83308,#10316);
#5789=LINE('',#83311,#10317);
#5790=LINE('',#83313,#10318);
#5791=LINE('',#83314,#10319);
#5792=LINE('',#83317,#10320);
#5793=LINE('',#83319,#10321);
#5794=LINE('',#83320,#10322);
#5795=LINE('',#83323,#10323);
#5796=LINE('',#83325,#10324);
#5797=LINE('',#83326,#10325);
#5798=LINE('',#83329,#10326);
#5799=LINE('',#83331,#10327);
#5800=LINE('',#83332,#10328);
#5801=LINE('',#83335,#10329);
#5802=LINE('',#83337,#10330);
#5803=LINE('',#83338,#10331);
#5804=LINE('',#83341,#10332);
#5805=LINE('',#83343,#10333);
#5806=LINE('',#83344,#10334);
#5807=LINE('',#83347,#10335);
#5808=LINE('',#83349,#10336);
#5809=LINE('',#83350,#10337);
#5810=LINE('',#83353,#10338);
#5811=LINE('',#83355,#10339);
#5812=LINE('',#83356,#10340);
#5813=LINE('',#83359,#10341);
#5814=LINE('',#83361,#10342);
#5815=LINE('',#83362,#10343);
#5816=LINE('',#83365,#10344);
#5817=LINE('',#83367,#10345);
#5818=LINE('',#83368,#10346);
#5819=LINE('',#83370,#10347);
#5820=LINE('',#83371,#10348);
#5821=LINE('',#83376,#10349);
#5822=LINE('',#83378,#10350);
#5823=LINE('',#83380,#10351);
#5824=LINE('',#83381,#10352);
#5825=LINE('',#83384,#10353);
#5826=LINE('',#83386,#10354);
#5827=LINE('',#83387,#10355);
#5828=LINE('',#83390,#10356);
#5829=LINE('',#83392,#10357);
#5830=LINE('',#83393,#10358);
#5831=LINE('',#83396,#10359);
#5832=LINE('',#83398,#10360);
#5833=LINE('',#83399,#10361);
#5834=LINE('',#83402,#10362);
#5835=LINE('',#83404,#10363);
#5836=LINE('',#83405,#10364);
#5837=LINE('',#83407,#10365);
#5838=LINE('',#83408,#10366);
#5839=LINE('',#83422,#10367);
#5840=LINE('',#83427,#10368);
#5841=LINE('',#83439,#10369);
#5842=LINE('',#83454,#10370);
#5843=LINE('',#83469,#10371);
#5844=LINE('',#83484,#10372);
#5845=LINE('',#83499,#10373);
#5846=LINE('',#83514,#10374);
#5847=LINE('',#83529,#10375);
#5848=LINE('',#83535,#10376);
#5849=LINE('',#83537,#10377);
#5850=LINE('',#83538,#10378);
#5851=LINE('',#83541,#10379);
#5852=LINE('',#83543,#10380);
#5853=LINE('',#83544,#10381);
#5854=LINE('',#83547,#10382);
#5855=LINE('',#83549,#10383);
#5856=LINE('',#83550,#10384);
#5857=LINE('',#83567,#10385);
#5858=LINE('',#83569,#10386);
#5859=LINE('',#83571,#10387);
#5860=LINE('',#83572,#10388);
#5861=LINE('',#83584,#10389);
#5862=LINE('',#83599,#10390);
#5863=LINE('',#83614,#10391);
#5864=LINE('',#83629,#10392);
#5865=LINE('',#83635,#10393);
#5866=LINE('',#83637,#10394);
#5867=LINE('',#83638,#10395);
#5868=LINE('',#83641,#10396);
#5869=LINE('',#83643,#10397);
#5870=LINE('',#83644,#10398);
#5871=LINE('',#83647,#10399);
#5872=LINE('',#83649,#10400);
#5873=LINE('',#83650,#10401);
#5874=LINE('',#83662,#10402);
#5875=LINE('',#83677,#10403);
#5876=LINE('',#83692,#10404);
#5877=LINE('',#83707,#10405);
#5878=LINE('',#83722,#10406);
#5879=LINE('',#83737,#10407);
#5880=LINE('',#83752,#10408);
#5881=LINE('',#83758,#10409);
#5882=LINE('',#83760,#10410);
#5883=LINE('',#83761,#10411);
#5884=LINE('',#83764,#10412);
#5885=LINE('',#83766,#10413);
#5886=LINE('',#83767,#10414);
#5887=LINE('',#83770,#10415);
#5888=LINE('',#83772,#10416);
#5889=LINE('',#83773,#10417);
#5890=LINE('',#83775,#10418);
#5891=LINE('',#83776,#10419);
#5892=LINE('',#83781,#10420);
#5893=LINE('',#83783,#10421);
#5894=LINE('',#83785,#10422);
#5895=LINE('',#83786,#10423);
#5896=LINE('',#83789,#10424);
#5897=LINE('',#83791,#10425);
#5898=LINE('',#83792,#10426);
#5899=LINE('',#83795,#10427);
#5900=LINE('',#83797,#10428);
#5901=LINE('',#83798,#10429);
#5902=LINE('',#83800,#10430);
#5903=LINE('',#83801,#10431);
#5904=LINE('',#83807,#10432);
#5905=LINE('',#83812,#10433);
#5906=LINE('',#83816,#10434);
#5907=LINE('',#83820,#10435);
#5908=LINE('',#83824,#10436);
#5909=LINE('',#83828,#10437);
#5910=LINE('',#83853,#10438);
#5911=LINE('',#83859,#10439);
#5912=LINE('',#83863,#10440);
#5913=LINE('',#83867,#10441);
#5914=LINE('',#83870,#10442);
#5915=LINE('',#83879,#10443);
#5916=LINE('',#83884,#10444);
#5917=LINE('',#83886,#10445);
#5918=LINE('',#83889,#10446);
#5919=LINE('',#83894,#10447);
#5920=LINE('',#83896,#10448);
#5921=LINE('',#83899,#10449);
#5922=LINE('',#83904,#10450);
#5923=LINE('',#83906,#10451);
#5924=LINE('',#83911,#10452);
#5925=LINE('',#83913,#10453);
#5926=LINE('',#83918,#10454);
#5927=LINE('',#83920,#10455);
#5928=LINE('',#83925,#10456);
#5929=LINE('',#83928,#10457);
#5930=LINE('',#83931,#10458);
#5931=LINE('',#83936,#10459);
#5932=LINE('',#83939,#10460);
#5933=LINE('',#83942,#10461);
#5934=LINE('',#83947,#10462);
#5935=LINE('',#83950,#10463);
#5936=LINE('',#83953,#10464);
#5937=LINE('',#83958,#10465);
#5938=LINE('',#83961,#10466);
#5939=LINE('',#83964,#10467);
#5940=LINE('',#83968,#10468);
#5941=LINE('',#83972,#10469);
#5942=LINE('',#83975,#10470);
#5943=LINE('',#83978,#10471);
#5944=LINE('',#83979,#10472);
#5945=LINE('',#83982,#10473);
#5946=LINE('',#83986,#10474);
#5947=LINE('',#83987,#10475);
#5948=LINE('',#83990,#10476);
#5949=LINE('',#83994,#10477);
#5950=LINE('',#83995,#10478);
#5951=LINE('',#83998,#10479);
#5952=LINE('',#84001,#10480);
#5953=LINE('',#84004,#10481);
#5954=LINE('',#84006,#10482);
#5955=LINE('',#84007,#10483);
#5956=LINE('',#84010,#10484);
#5957=LINE('',#84014,#10485);
#5958=LINE('',#84015,#10486);
#5959=LINE('',#84018,#10487);
#5960=LINE('',#84021,#10488);
#5961=LINE('',#84022,#10489);
#5962=LINE('',#84024,#10490);
#5963=LINE('',#84026,#10491);
#5964=LINE('',#84028,#10492);
#5965=LINE('',#84031,#10493);
#5966=LINE('',#84032,#10494);
#5967=LINE('',#84035,#10495);
#5968=LINE('',#84039,#10496);
#5969=LINE('',#84040,#10497);
#5970=LINE('',#84044,#10498);
#5971=LINE('',#84046,#10499);
#5972=LINE('',#84048,#10500);
#9885=VECTOR('',#64627,10.);
#9886=VECTOR('',#64628,10.);
#9887=VECTOR('',#64629,10.);
#9888=VECTOR('',#64630,10.);
#9889=VECTOR('',#64633,10.);
#9890=VECTOR('',#64634,10.);
#9891=VECTOR('',#64635,10.);
#9892=VECTOR('',#64638,10.);
#9893=VECTOR('',#64639,10.);
#9894=VECTOR('',#64640,10.);
#9895=VECTOR('',#64643,10.);
#9896=VECTOR('',#64644,10.);
#9897=VECTOR('',#64645,10.);
#9898=VECTOR('',#64648,10.);
#9899=VECTOR('',#64649,10.);
#9900=VECTOR('',#64650,10.);
#9901=VECTOR('',#64653,10.);
#9902=VECTOR('',#64654,10.);
#9903=VECTOR('',#64655,10.);
#9904=VECTOR('',#64658,10.);
#9905=VECTOR('',#64659,10.);
#9906=VECTOR('',#64660,10.);
#9907=VECTOR('',#64663,10.);
#9908=VECTOR('',#64664,10.);
#9909=VECTOR('',#64665,10.);
#9910=VECTOR('',#64668,10.);
#9911=VECTOR('',#64669,10.);
#9912=VECTOR('',#64670,10.);
#9913=VECTOR('',#64673,10.);
#9914=VECTOR('',#64674,10.);
#9915=VECTOR('',#64675,10.);
#9916=VECTOR('',#64678,10.);
#9917=VECTOR('',#64679,10.);
#9918=VECTOR('',#64680,10.);
#9919=VECTOR('',#64683,10.);
#9920=VECTOR('',#64684,10.);
#9921=VECTOR('',#64689,10.);
#9922=VECTOR('',#64690,10.);
#9923=VECTOR('',#64691,10.);
#9924=VECTOR('',#64692,10.);
#9925=VECTOR('',#64695,10.);
#9926=VECTOR('',#64696,10.);
#9927=VECTOR('',#64697,10.);
#9928=VECTOR('',#64700,10.);
#9929=VECTOR('',#64701,10.);
#9930=VECTOR('',#64702,10.);
#9931=VECTOR('',#64705,10.);
#9932=VECTOR('',#64706,10.);
#9933=VECTOR('',#64709,10.);
#9934=VECTOR('',#64710,10.);
#9935=VECTOR('',#64711,10.);
#9936=VECTOR('',#64712,10.);
#9937=VECTOR('',#64713,10.);
#9938=VECTOR('',#64714,10.);
#9939=VECTOR('',#64715,10.);
#9940=VECTOR('',#64716,10.);
#9941=VECTOR('',#64717,10.);
#9942=VECTOR('',#64718,10.);
#9943=VECTOR('',#64719,10.);
#9944=VECTOR('',#64720,10.);
#9945=VECTOR('',#64721,10.);
#9946=VECTOR('',#64722,10.);
#9947=VECTOR('',#64725,10.);
#9948=VECTOR('',#64726,10.);
#9949=VECTOR('',#64727,10.);
#9950=VECTOR('',#64728,10.);
#9951=VECTOR('',#64729,10.);
#9952=VECTOR('',#64730,10.);
#9953=VECTOR('',#64731,10.);
#9954=VECTOR('',#64732,10.);
#9955=VECTOR('',#64733,10.);
#9956=VECTOR('',#64734,10.);
#9957=VECTOR('',#64735,10.);
#9958=VECTOR('',#64736,10.);
#9959=VECTOR('',#64737,10.);
#9960=VECTOR('',#64738,10.);
#9961=VECTOR('',#64739,10.);
#9962=VECTOR('',#64740,10.);
#9963=VECTOR('',#64741,10.);
#9964=VECTOR('',#64742,10.);
#9965=VECTOR('',#64743,10.);
#9966=VECTOR('',#64744,10.);
#9967=VECTOR('',#64745,10.);
#9968=VECTOR('',#64748,10.);
#9969=VECTOR('',#64749,10.);
#9970=VECTOR('',#64750,10.);
#9971=VECTOR('',#64751,10.);
#9972=VECTOR('',#64754,10.);
#9973=VECTOR('',#64755,10.);
#9974=VECTOR('',#64756,10.);
#9975=VECTOR('',#64757,10.);
#9976=VECTOR('',#64758,10.);
#9977=VECTOR('',#64759,10.);
#9978=VECTOR('',#64760,10.);
#9979=VECTOR('',#64761,10.);
#9980=VECTOR('',#64762,10.);
#9981=VECTOR('',#64765,10.);
#9982=VECTOR('',#64766,10.);
#9983=VECTOR('',#64767,10.);
#9984=VECTOR('',#64768,10.);
#9985=VECTOR('',#64769,10.);
#9986=VECTOR('',#64770,10.);
#9987=VECTOR('',#64771,10.);
#9988=VECTOR('',#64772,10.);
#9989=VECTOR('',#64773,10.);
#9990=VECTOR('',#64774,10.);
#9991=VECTOR('',#64775,10.);
#9992=VECTOR('',#64776,10.);
#9993=VECTOR('',#64777,10.);
#9994=VECTOR('',#64780,10.);
#9995=VECTOR('',#64781,10.);
#9996=VECTOR('',#64782,10.);
#9997=VECTOR('',#64783,10.);
#9998=VECTOR('',#64788,10.);
#9999=VECTOR('',#64789,10.);
#10000=VECTOR('',#64790,10.);
#10001=VECTOR('',#64791,10.);
#10002=VECTOR('',#64794,10.);
#10003=VECTOR('',#64795,10.);
#10004=VECTOR('',#64796,10.);
#10005=VECTOR('',#64799,10.);
#10006=VECTOR('',#64800,10.);
#10007=VECTOR('',#64801,10.);
#10008=VECTOR('',#64804,10.);
#10009=VECTOR('',#64805,10.);
#10010=VECTOR('',#64806,10.);
#10011=VECTOR('',#64809,10.);
#10012=VECTOR('',#64810,10.);
#10013=VECTOR('',#64811,10.);
#10014=VECTOR('',#64814,10.);
#10015=VECTOR('',#64815,10.);
#10016=VECTOR('',#64820,10.);
#10017=VECTOR('',#64821,10.);
#10018=VECTOR('',#64822,10.);
#10019=VECTOR('',#64823,10.);
#10020=VECTOR('',#64826,10.);
#10021=VECTOR('',#64827,10.);
#10022=VECTOR('',#64828,10.);
#10023=VECTOR('',#64831,10.);
#10024=VECTOR('',#64832,10.);
#10025=VECTOR('',#64833,10.);
#10026=VECTOR('',#64836,10.);
#10027=VECTOR('',#64837,10.);
#10028=VECTOR('',#64838,10.);
#10029=VECTOR('',#64841,10.);
#10030=VECTOR('',#64842,10.);
#10031=VECTOR('',#64843,10.);
#10032=VECTOR('',#64846,10.);
#10033=VECTOR('',#64847,10.);
#10034=VECTOR('',#64848,10.);
#10035=VECTOR('',#64851,10.);
#10036=VECTOR('',#64852,10.);
#10037=VECTOR('',#64853,10.);
#10038=VECTOR('',#64856,10.);
#10039=VECTOR('',#64857,10.);
#10040=VECTOR('',#64860,10.);
#10041=VECTOR('',#64861,10.);
#10042=VECTOR('',#64862,10.);
#10043=VECTOR('',#64863,10.);
#10044=VECTOR('',#64864,10.);
#10045=VECTOR('',#64867,10.);
#10046=VECTOR('',#64868,10.);
#10047=VECTOR('',#64869,10.);
#10048=VECTOR('',#64872,10.);
#10049=VECTOR('',#64873,10.);
#10050=VECTOR('',#64874,10.);
#10051=VECTOR('',#64877,10.);
#10052=VECTOR('',#64878,10.);
#10053=VECTOR('',#64879,10.);
#10054=VECTOR('',#64880,10.);
#10055=VECTOR('',#64881,10.);
#10056=VECTOR('',#64882,10.);
#10057=VECTOR('',#64883,10.);
#10058=VECTOR('',#64884,10.);
#10059=VECTOR('',#64885,10.);
#10060=VECTOR('',#64888,10.);
#10061=VECTOR('',#64889,10.);
#10062=VECTOR('',#64890,10.);
#10063=VECTOR('',#64893,10.);
#10064=VECTOR('',#64894,10.);
#10065=VECTOR('',#64895,10.);
#10066=VECTOR('',#64898,10.);
#10067=VECTOR('',#64899,10.);
#10068=VECTOR('',#64900,10.);
#10069=VECTOR('',#64905,10.);
#10070=VECTOR('',#64906,10.);
#10071=VECTOR('',#64907,10.);
#10072=VECTOR('',#64908,10.);
#10073=VECTOR('',#64909,10.);
#10074=VECTOR('',#64910,10.);
#10075=VECTOR('',#64911,10.);
#10076=VECTOR('',#64912,10.);
#10077=VECTOR('',#64915,10.);
#10078=VECTOR('',#64916,10.);
#10079=VECTOR('',#64917,10.);
#10080=VECTOR('',#64920,10.);
#10081=VECTOR('',#64921,10.);
#10082=VECTOR('',#64922,10.);
#10083=VECTOR('',#64925,10.);
#10084=VECTOR('',#64926,10.);
#10085=VECTOR('',#64927,10.);
#10086=VECTOR('',#64928,10.);
#10087=VECTOR('',#64929,10.);
#10088=VECTOR('',#64930,10.);
#10089=VECTOR('',#64931,10.);
#10090=VECTOR('',#64932,10.);
#10091=VECTOR('',#64933,10.);
#10092=VECTOR('',#64934,10.);
#10093=VECTOR('',#64937,10.);
#10094=VECTOR('',#64938,10.);
#10095=VECTOR('',#64939,10.);
#10096=VECTOR('',#64942,10.);
#10097=VECTOR('',#64943,10.);
#10098=VECTOR('',#64944,10.);
#10099=VECTOR('',#64947,10.);
#10100=VECTOR('',#64948,10.);
#10101=VECTOR('',#64949,10.);
#10102=VECTOR('',#64952,10.);
#10103=VECTOR('',#64953,10.);
#10104=VECTOR('',#64958,10.);
#10105=VECTOR('',#64959,10.);
#10106=VECTOR('',#64960,10.);
#10107=VECTOR('',#64961,10.);
#10108=VECTOR('',#64964,10.);
#10109=VECTOR('',#64965,10.);
#10110=VECTOR('',#64966,10.);
#10111=VECTOR('',#64969,10.);
#10112=VECTOR('',#64970,10.);
#10113=VECTOR('',#64971,10.);
#10114=VECTOR('',#64974,10.);
#10115=VECTOR('',#64975,10.);
#10116=VECTOR('',#64976,10.);
#10117=VECTOR('',#64979,10.);
#10118=VECTOR('',#64980,10.);
#10119=VECTOR('',#64981,10.);
#10120=VECTOR('',#64984,10.);
#10121=VECTOR('',#64985,10.);
#10122=VECTOR('',#64986,10.);
#10123=VECTOR('',#64989,10.);
#10124=VECTOR('',#64990,10.);
#10125=VECTOR('',#64991,10.);
#10126=VECTOR('',#64994,10.);
#10127=VECTOR('',#64995,10.);
#10128=VECTOR('',#64998,10.);
#10129=VECTOR('',#64999,10.);
#10130=VECTOR('',#65000,10.);
#10131=VECTOR('',#65003,10.);
#10132=VECTOR('',#65004,10.);
#10133=VECTOR('',#65005,10.);
#10134=VECTOR('',#65006,10.);
#10135=VECTOR('',#65007,10.);
#10136=VECTOR('',#65010,10.);
#10137=VECTOR('',#65011,10.);
#10138=VECTOR('',#65012,10.);
#10139=VECTOR('',#65015,10.);
#10140=VECTOR('',#65016,10.);
#10141=VECTOR('',#65017,10.);
#10142=VECTOR('',#65020,10.);
#10143=VECTOR('',#65021,10.);
#10144=VECTOR('',#65022,10.);
#10145=VECTOR('',#65025,10.);
#10146=VECTOR('',#65026,10.);
#10147=VECTOR('',#65029,10.);
#10148=VECTOR('',#65030,10.);
#10149=VECTOR('',#65031,10.);
#10150=VECTOR('',#65032,10.);
#10151=VECTOR('',#65033,10.);
#10152=VECTOR('',#65034,10.);
#10153=VECTOR('',#65035,10.);
#10154=VECTOR('',#65036,10.);
#10155=VECTOR('',#65037,10.);
#10156=VECTOR('',#65038,10.);
#10157=VECTOR('',#65039,10.);
#10158=VECTOR('',#65040,10.);
#10159=VECTOR('',#65043,10.);
#10160=VECTOR('',#65044,10.);
#10161=VECTOR('',#65045,10.);
#10162=VECTOR('',#65048,10.);
#10163=VECTOR('',#65049,10.);
#10164=VECTOR('',#65050,10.);
#10165=VECTOR('',#65051,10.);
#10166=VECTOR('',#65052,10.);
#10167=VECTOR('',#65055,10.);
#10168=VECTOR('',#65056,10.);
#10169=VECTOR('',#65057,10.);
#10170=VECTOR('',#65060,10.);
#10171=VECTOR('',#65061,10.);
#10172=VECTOR('',#65062,10.);
#10173=VECTOR('',#65065,10.);
#10174=VECTOR('',#65066,10.);
#10175=VECTOR('',#65067,10.);
#10176=VECTOR('',#65070,10.);
#10177=VECTOR('',#65071,10.);
#10178=VECTOR('',#65076,10.);
#10179=VECTOR('',#65077,10.);
#10180=VECTOR('',#65078,10.);
#10181=VECTOR('',#65079,10.);
#10182=VECTOR('',#65082,10.);
#10183=VECTOR('',#65083,10.);
#10184=VECTOR('',#65084,10.);
#10185=VECTOR('',#65087,10.);
#10186=VECTOR('',#65088,10.);
#10187=VECTOR('',#65089,10.);
#10188=VECTOR('',#65092,10.);
#10189=VECTOR('',#65093,10.);
#10190=VECTOR('',#65096,10.);
#10191=VECTOR('',#65097,10.);
#10192=VECTOR('',#65098,10.);
#10193=VECTOR('',#65099,10.);
#10194=VECTOR('',#65100,10.);
#10195=VECTOR('',#65101,10.);
#10196=VECTOR('',#65104,10.);
#10197=VECTOR('',#65105,10.);
#10198=VECTOR('',#65106,10.);
#10199=VECTOR('',#65109,10.);
#10200=VECTOR('',#65110,10.);
#10201=VECTOR('',#65111,10.);
#10202=VECTOR('',#65114,10.);
#10203=VECTOR('',#65115,10.);
#10204=VECTOR('',#65116,10.);
#10205=VECTOR('',#65119,10.);
#10206=VECTOR('',#65120,10.);
#10207=VECTOR('',#65121,10.);
#10208=VECTOR('',#65124,10.);
#10209=VECTOR('',#65125,10.);
#10210=VECTOR('',#65126,10.);
#10211=VECTOR('',#65129,10.);
#10212=VECTOR('',#65130,10.);
#10213=VECTOR('',#65131,10.);
#10214=VECTOR('',#65132,10.);
#10215=VECTOR('',#65133,10.);
#10216=VECTOR('',#65134,10.);
#10217=VECTOR('',#65135,10.);
#10218=VECTOR('',#65136,10.);
#10219=VECTOR('',#65137,10.);
#10220=VECTOR('',#65138,10.);
#10221=VECTOR('',#65139,10.);
#10222=VECTOR('',#65142,10.);
#10223=VECTOR('',#65143,10.);
#10224=VECTOR('',#65144,10.);
#10225=VECTOR('',#65145,10.);
#10226=VECTOR('',#65148,10.);
#10227=VECTOR('',#65149,10.);
#10228=VECTOR('',#65150,10.);
#10229=VECTOR('',#65151,10.);
#10230=VECTOR('',#65152,10.);
#10231=VECTOR('',#65153,10.);
#10232=VECTOR('',#65154,10.);
#10233=VECTOR('',#65155,10.);
#10234=VECTOR('',#65156,10.);
#10235=VECTOR('',#65157,10.);
#10236=VECTOR('',#65158,10.);
#10237=VECTOR('',#65161,10.);
#10238=VECTOR('',#65162,10.);
#10239=VECTOR('',#65163,10.);
#10240=VECTOR('',#65164,10.);
#10241=VECTOR('',#65165,10.);
#10242=VECTOR('',#65166,10.);
#10243=VECTOR('',#65167,10.);
#10244=VECTOR('',#65168,10.);
#10245=VECTOR('',#65169,10.);
#10246=VECTOR('',#65170,10.);
#10247=VECTOR('',#65171,10.);
#10248=VECTOR('',#65172,10.);
#10249=VECTOR('',#65175,10.);
#10250=VECTOR('',#65176,10.);
#10251=VECTOR('',#65177,10.);
#10252=VECTOR('',#65178,10.);
#10253=VECTOR('',#65179,10.);
#10254=VECTOR('',#65184,10.);
#10255=VECTOR('',#65185,10.);
#10256=VECTOR('',#65186,10.);
#10257=VECTOR('',#65187,10.);
#10258=VECTOR('',#65190,10.);
#10259=VECTOR('',#65191,10.);
#10260=VECTOR('',#65192,10.);
#10261=VECTOR('',#65195,10.);
#10262=VECTOR('',#65196,10.);
#10263=VECTOR('',#65197,10.);
#10264=VECTOR('',#65200,10.);
#10265=VECTOR('',#65201,10.);
#10266=VECTOR('',#65202,10.);
#10267=VECTOR('',#65205,10.);
#10268=VECTOR('',#65206,10.);
#10269=VECTOR('',#65207,10.);
#10270=VECTOR('',#65210,10.);
#10271=VECTOR('',#65211,10.);
#10272=VECTOR('',#65212,10.);
#10273=VECTOR('',#65215,10.);
#10274=VECTOR('',#65216,10.);
#10275=VECTOR('',#65217,10.);
#10276=VECTOR('',#65220,10.);
#10277=VECTOR('',#65221,10.);
#10278=VECTOR('',#65222,10.);
#10279=VECTOR('',#65225,10.);
#10280=VECTOR('',#65226,10.);
#10281=VECTOR('',#65227,10.);
#10282=VECTOR('',#65230,10.);
#10283=VECTOR('',#65231,10.);
#10284=VECTOR('',#65232,10.);
#10285=VECTOR('',#65235,10.);
#10286=VECTOR('',#65236,10.);
#10287=VECTOR('',#65237,10.);
#10288=VECTOR('',#65240,10.);
#10289=VECTOR('',#65241,10.);
#10290=VECTOR('',#65246,10.);
#10291=VECTOR('',#65247,10.);
#10292=VECTOR('',#65248,10.);
#10293=VECTOR('',#65249,10.);
#10294=VECTOR('',#65252,10.);
#10295=VECTOR('',#65253,10.);
#10296=VECTOR('',#65254,10.);
#10297=VECTOR('',#65257,10.);
#10298=VECTOR('',#65258,10.);
#10299=VECTOR('',#65259,10.);
#10300=VECTOR('',#65262,10.);
#10301=VECTOR('',#65263,10.);
#10302=VECTOR('',#65266,10.);
#10303=VECTOR('',#65267,10.);
#10304=VECTOR('',#65268,10.);
#10305=VECTOR('',#65269,10.);
#10306=VECTOR('',#65270,10.);
#10307=VECTOR('',#65271,10.);
#10308=VECTOR('',#65272,10.);
#10309=VECTOR('',#65273,10.);
#10310=VECTOR('',#65274,10.);
#10311=VECTOR('',#65275,10.);
#10312=VECTOR('',#65276,10.);
#10313=VECTOR('',#65281,10.);
#10314=VECTOR('',#65282,10.);
#10315=VECTOR('',#65283,10.);
#10316=VECTOR('',#65284,10.);
#10317=VECTOR('',#65287,10.);
#10318=VECTOR('',#65288,10.);
#10319=VECTOR('',#65289,10.);
#10320=VECTOR('',#65292,10.);
#10321=VECTOR('',#65293,10.);
#10322=VECTOR('',#65294,10.);
#10323=VECTOR('',#65297,10.);
#10324=VECTOR('',#65298,10.);
#10325=VECTOR('',#65299,10.);
#10326=VECTOR('',#65302,10.);
#10327=VECTOR('',#65303,10.);
#10328=VECTOR('',#65304,10.);
#10329=VECTOR('',#65307,10.);
#10330=VECTOR('',#65308,10.);
#10331=VECTOR('',#65309,10.);
#10332=VECTOR('',#65312,10.);
#10333=VECTOR('',#65313,10.);
#10334=VECTOR('',#65314,10.);
#10335=VECTOR('',#65317,10.);
#10336=VECTOR('',#65318,10.);
#10337=VECTOR('',#65319,10.);
#10338=VECTOR('',#65322,10.);
#10339=VECTOR('',#65323,10.);
#10340=VECTOR('',#65324,10.);
#10341=VECTOR('',#65327,10.);
#10342=VECTOR('',#65328,10.);
#10343=VECTOR('',#65329,10.);
#10344=VECTOR('',#65332,10.);
#10345=VECTOR('',#65333,10.);
#10346=VECTOR('',#65334,10.);
#10347=VECTOR('',#65337,10.);
#10348=VECTOR('',#65338,10.);
#10349=VECTOR('',#65343,10.);
#10350=VECTOR('',#65344,10.);
#10351=VECTOR('',#65345,10.);
#10352=VECTOR('',#65346,10.);
#10353=VECTOR('',#65349,10.);
#10354=VECTOR('',#65350,10.);
#10355=VECTOR('',#65351,10.);
#10356=VECTOR('',#65354,10.);
#10357=VECTOR('',#65355,10.);
#10358=VECTOR('',#65356,10.);
#10359=VECTOR('',#65359,10.);
#10360=VECTOR('',#65360,10.);
#10361=VECTOR('',#65361,10.);
#10362=VECTOR('',#65364,10.);
#10363=VECTOR('',#65365,10.);
#10364=VECTOR('',#65366,10.);
#10365=VECTOR('',#65369,10.);
#10366=VECTOR('',#65370,10.);
#10367=VECTOR('',#65373,10.);
#10368=VECTOR('',#65374,10.);
#10369=VECTOR('',#65375,10.);
#10370=VECTOR('',#65376,10.);
#10371=VECTOR('',#65377,10.);
#10372=VECTOR('',#65378,10.);
#10373=VECTOR('',#65379,10.);
#10374=VECTOR('',#65380,10.);
#10375=VECTOR('',#65381,10.);
#10376=VECTOR('',#65384,10.);
#10377=VECTOR('',#65385,10.);
#10378=VECTOR('',#65386,10.);
#10379=VECTOR('',#65389,10.);
#10380=VECTOR('',#65390,10.);
#10381=VECTOR('',#65391,10.);
#10382=VECTOR('',#65394,10.);
#10383=VECTOR('',#65395,10.);
#10384=VECTOR('',#65396,10.);
#10385=VECTOR('',#65401,10.);
#10386=VECTOR('',#65402,10.);
#10387=VECTOR('',#65403,10.);
#10388=VECTOR('',#65404,10.);
#10389=VECTOR('',#65405,10.);
#10390=VECTOR('',#65406,10.);
#10391=VECTOR('',#65407,10.);
#10392=VECTOR('',#65408,10.);
#10393=VECTOR('',#65411,10.);
#10394=VECTOR('',#65412,10.);
#10395=VECTOR('',#65413,10.);
#10396=VECTOR('',#65416,10.);
#10397=VECTOR('',#65417,10.);
#10398=VECTOR('',#65418,10.);
#10399=VECTOR('',#65421,10.);
#10400=VECTOR('',#65422,10.);
#10401=VECTOR('',#65423,10.);
#10402=VECTOR('',#65424,10.);
#10403=VECTOR('',#65425,10.);
#10404=VECTOR('',#65426,10.);
#10405=VECTOR('',#65427,10.);
#10406=VECTOR('',#65428,10.);
#10407=VECTOR('',#65429,10.);
#10408=VECTOR('',#65430,10.);
#10409=VECTOR('',#65433,10.);
#10410=VECTOR('',#65434,10.);
#10411=VECTOR('',#65435,10.);
#10412=VECTOR('',#65438,10.);
#10413=VECTOR('',#65439,10.);
#10414=VECTOR('',#65440,10.);
#10415=VECTOR('',#65443,10.);
#10416=VECTOR('',#65444,10.);
#10417=VECTOR('',#65445,10.);
#10418=VECTOR('',#65448,10.);
#10419=VECTOR('',#65449,10.);
#10420=VECTOR('',#65454,10.);
#10421=VECTOR('',#65455,10.);
#10422=VECTOR('',#65456,10.);
#10423=VECTOR('',#65457,10.);
#10424=VECTOR('',#65460,10.);
#10425=VECTOR('',#65461,10.);
#10426=VECTOR('',#65462,10.);
#10427=VECTOR('',#65465,10.);
#10428=VECTOR('',#65466,10.);
#10429=VECTOR('',#65467,10.);
#10430=VECTOR('',#65470,10.);
#10431=VECTOR('',#65471,10.);
#10432=VECTOR('',#65478,4.75);
#10433=VECTOR('',#65485,4.5);
#10434=VECTOR('',#65488,10.);
#10435=VECTOR('',#65491,10.);
#10436=VECTOR('',#65494,10.);
#10437=VECTOR('',#65497,10.);
#10438=VECTOR('',#65524,4.75);
#10439=VECTOR('',#65529,10.);
#10440=VECTOR('',#65532,10.);
#10441=VECTOR('',#65535,10.);
#10442=VECTOR('',#65538,10.);
#10443=VECTOR('',#65547,4.75);
#10444=VECTOR('',#65554,4.5);
#10445=VECTOR('',#65557,4.75);
#10446=VECTOR('',#65560,4.75);
#10447=VECTOR('',#65567,4.5);
#10448=VECTOR('',#65570,4.75);
#10449=VECTOR('',#65573,4.75);
#10450=VECTOR('',#65580,4.5);
#10451=VECTOR('',#65583,4.75);
#10452=VECTOR('',#65588,1.5);
#10453=VECTOR('',#65591,3.);
#10454=VECTOR('',#65596,1.5);
#10455=VECTOR('',#65599,3.);
#10456=VECTOR('',#65604,1.525);
#10457=VECTOR('',#65607,3.175);
#10458=VECTOR('',#65612,3.05);
#10459=VECTOR('',#65617,1.525);
#10460=VECTOR('',#65620,3.175);
#10461=VECTOR('',#65625,3.05);
#10462=VECTOR('',#65630,1.525);
#10463=VECTOR('',#65633,3.175);
#10464=VECTOR('',#65638,3.05);
#10465=VECTOR('',#65643,1.525);
#10466=VECTOR('',#65646,3.175);
#10467=VECTOR('',#65651,3.05);
#10468=VECTOR('',#65656,20.025);
#10469=VECTOR('',#65661,10.);
#10470=VECTOR('',#65664,10.);
#10471=VECTOR('',#65667,10.);
#10472=VECTOR('',#65668,10.);
#10473=VECTOR('',#65671,10.);
#10474=VECTOR('',#65676,10.);
#10475=VECTOR('',#65677,10.);
#10476=VECTOR('',#65680,10.);
#10477=VECTOR('',#65685,10.);
#10478=VECTOR('',#65686,10.);
#10479=VECTOR('',#65689,10.);
#10480=VECTOR('',#65694,10.);
#10481=VECTOR('',#65697,10.);
#10482=VECTOR('',#65698,10.);
#10483=VECTOR('',#65699,10.);
#10484=VECTOR('',#65702,10.);
#10485=VECTOR('',#65707,10.);
#10486=VECTOR('',#65708,10.);
#10487=VECTOR('',#65711,10.);
#10488=VECTOR('',#65716,10.);
#10489=VECTOR('',#65717,10.);
#10490=VECTOR('',#65720,10.);
#10491=VECTOR('',#65723,10.);
#10492=VECTOR('',#65726,10.);
#10493=VECTOR('',#65729,10.);
#10494=VECTOR('',#65730,10.);
#10495=VECTOR('',#65733,10.);
#10496=VECTOR('',#65738,10.);
#10497=VECTOR('',#65739,10.);
#10498=VECTOR('',#65746,10.);
#10499=VECTOR('',#65749,10.);
#10500=VECTOR('',#65752,10.);
#12735=PLANE('',#54217);
#12736=PLANE('',#54218);
#12737=PLANE('',#54219);
#12738=PLANE('',#54220);
#12739=PLANE('',#54221);
#12740=PLANE('',#54222);
#12741=PLANE('',#54223);
#12742=PLANE('',#54224);
#12743=PLANE('',#54225);
#12744=PLANE('',#54226);
#12745=PLANE('',#54227);
#12746=PLANE('',#54228);
#12747=PLANE('',#54229);
#12748=PLANE('',#54230);
#12749=PLANE('',#54231);
#12750=PLANE('',#54232);
#12751=PLANE('',#54233);
#12752=PLANE('',#54234);
#12753=PLANE('',#54235);
#12754=PLANE('',#54236);
#12755=PLANE('',#54237);
#12756=PLANE('',#54238);
#12757=PLANE('',#54239);
#12758=PLANE('',#54240);
#12759=PLANE('',#54241);
#12760=PLANE('',#54242);
#12761=PLANE('',#54243);
#12762=PLANE('',#54244);
#12763=PLANE('',#54245);
#12764=PLANE('',#54246);
#12765=PLANE('',#54247);
#12766=PLANE('',#54248);
#12767=PLANE('',#54249);
#12768=PLANE('',#54250);
#12769=PLANE('',#54251);
#12770=PLANE('',#54252);
#12771=PLANE('',#54253);
#12772=PLANE('',#54254);
#12773=PLANE('',#54255);
#12774=PLANE('',#54256);
#12775=PLANE('',#54257);
#12776=PLANE('',#54258);
#12777=PLANE('',#54259);
#12778=PLANE('',#54260);
#12779=PLANE('',#54261);
#12780=PLANE('',#54262);
#12781=PLANE('',#54263);
#12782=PLANE('',#54264);
#12783=PLANE('',#54265);
#12784=PLANE('',#54266);
#12785=PLANE('',#54267);
#12786=PLANE('',#54268);
#12787=PLANE('',#54269);
#12788=PLANE('',#54270);
#12789=PLANE('',#54271);
#12790=PLANE('',#54272);
#12791=PLANE('',#54273);
#12792=PLANE('',#54274);
#12793=PLANE('',#54275);
#12794=PLANE('',#54276);
#12795=PLANE('',#54277);
#12796=PLANE('',#54278);
#12797=PLANE('',#54279);
#12798=PLANE('',#54280);
#12799=PLANE('',#54281);
#12800=PLANE('',#54282);
#12801=PLANE('',#54283);
#12802=PLANE('',#54284);
#12803=PLANE('',#54285);
#12804=PLANE('',#54286);
#12805=PLANE('',#54287);
#12806=PLANE('',#54288);
#12807=PLANE('',#54289);
#12808=PLANE('',#54290);
#12809=PLANE('',#54291);
#12810=PLANE('',#54292);
#12811=PLANE('',#54293);
#12812=PLANE('',#54294);
#12813=PLANE('',#54295);
#12814=PLANE('',#54296);
#12815=PLANE('',#54297);
#12816=PLANE('',#54298);
#12817=PLANE('',#54299);
#12818=PLANE('',#54300);
#12819=PLANE('',#54301);
#12820=PLANE('',#54302);
#12821=PLANE('',#54303);
#12822=PLANE('',#54304);
#12823=PLANE('',#54305);
#12824=PLANE('',#54306);
#12825=PLANE('',#54307);
#12826=PLANE('',#54308);
#12827=PLANE('',#54309);
#12828=PLANE('',#54310);
#12829=PLANE('',#54311);
#12830=PLANE('',#54312);
#12831=PLANE('',#54313);
#12832=PLANE('',#54314);
#12833=PLANE('',#54315);
#12834=PLANE('',#54316);
#12835=PLANE('',#54317);
#12836=PLANE('',#54318);
#12837=PLANE('',#54319);
#12838=PLANE('',#54320);
#12839=PLANE('',#54321);
#12840=PLANE('',#54322);
#12841=PLANE('',#54323);
#12842=PLANE('',#54324);
#12843=PLANE('',#54325);
#12844=PLANE('',#54326);
#12845=PLANE('',#54327);
#12846=PLANE('',#54328);
#12847=PLANE('',#54329);
#12848=PLANE('',#54330);
#12849=PLANE('',#54331);
#12850=PLANE('',#54332);
#12851=PLANE('',#54333);
#12852=PLANE('',#54334);
#12853=PLANE('',#54335);
#12854=PLANE('',#54336);
#12855=PLANE('',#54337);
#12856=PLANE('',#54338);
#12857=PLANE('',#54339);
#12858=PLANE('',#54340);
#12859=PLANE('',#54341);
#12860=PLANE('',#54342);
#12861=PLANE('',#54343);
#12862=PLANE('',#54344);
#12863=PLANE('',#54345);
#12864=PLANE('',#54346);
#12865=PLANE('',#54347);
#12866=PLANE('',#54348);
#12867=PLANE('',#54349);
#12868=PLANE('',#54350);
#12869=PLANE('',#54351);
#12870=PLANE('',#54352);
#12871=PLANE('',#54353);
#12872=PLANE('',#54354);
#12873=PLANE('',#54355);
#12874=PLANE('',#54356);
#12875=PLANE('',#54357);
#12876=PLANE('',#54358);
#12877=PLANE('',#54359);
#12878=PLANE('',#54360);
#12879=PLANE('',#54361);
#12880=PLANE('',#54362);
#12881=PLANE('',#54363);
#12882=PLANE('',#54364);
#12883=PLANE('',#54365);
#12884=PLANE('',#54366);
#12885=PLANE('',#54367);
#12886=PLANE('',#54373);
#12887=PLANE('',#54390);
#12888=PLANE('',#54441);
#12889=PLANE('',#54444);
#12890=PLANE('',#54447);
#12891=PLANE('',#54450);
#12892=PLANE('',#54453);
#12893=PLANE('',#54454);
#12894=PLANE('',#54457);
#12895=PLANE('',#54460);
#12896=PLANE('',#54462);
#12897=PLANE('',#54464);
#12898=PLANE('',#54467);
#12899=PLANE('',#54471);
#12900=PLANE('',#54473);
#15033=FACE_OUTER_BOUND('',#17745,.T.);
#15034=FACE_OUTER_BOUND('',#17746,.T.);
#15035=FACE_OUTER_BOUND('',#17747,.T.);
#15036=FACE_OUTER_BOUND('',#17748,.T.);
#15037=FACE_OUTER_BOUND('',#17749,.T.);
#15038=FACE_OUTER_BOUND('',#17750,.T.);
#15039=FACE_OUTER_BOUND('',#17751,.T.);
#15040=FACE_OUTER_BOUND('',#17752,.T.);
#15041=FACE_OUTER_BOUND('',#17753,.T.);
#15042=FACE_OUTER_BOUND('',#17754,.T.);
#15043=FACE_OUTER_BOUND('',#17755,.T.);
#15044=FACE_OUTER_BOUND('',#17756,.T.);
#15045=FACE_OUTER_BOUND('',#17757,.T.);
#15046=FACE_OUTER_BOUND('',#17758,.T.);
#15047=FACE_OUTER_BOUND('',#17759,.T.);
#15048=FACE_OUTER_BOUND('',#17760,.T.);
#15049=FACE_OUTER_BOUND('',#17761,.T.);
#15050=FACE_OUTER_BOUND('',#17762,.T.);
#15051=FACE_OUTER_BOUND('',#17763,.T.);
#15052=FACE_OUTER_BOUND('',#17764,.T.);
#15053=FACE_OUTER_BOUND('',#17765,.T.);
#15054=FACE_OUTER_BOUND('',#17766,.T.);
#15055=FACE_OUTER_BOUND('',#17767,.T.);
#15056=FACE_OUTER_BOUND('',#17768,.T.);
#15057=FACE_OUTER_BOUND('',#17769,.T.);
#15058=FACE_OUTER_BOUND('',#17770,.T.);
#15059=FACE_OUTER_BOUND('',#17771,.T.);
#15060=FACE_OUTER_BOUND('',#17772,.T.);
#15061=FACE_OUTER_BOUND('',#17773,.T.);
#15062=FACE_OUTER_BOUND('',#17774,.T.);
#15063=FACE_OUTER_BOUND('',#17775,.T.);
#15064=FACE_OUTER_BOUND('',#17776,.T.);
#15065=FACE_OUTER_BOUND('',#17777,.T.);
#15066=FACE_OUTER_BOUND('',#17778,.T.);
#15067=FACE_OUTER_BOUND('',#17779,.T.);
#15068=FACE_OUTER_BOUND('',#17780,.T.);
#15069=FACE_OUTER_BOUND('',#17781,.T.);
#15070=FACE_OUTER_BOUND('',#17782,.T.);
#15071=FACE_OUTER_BOUND('',#17783,.T.);
#15072=FACE_OUTER_BOUND('',#17784,.T.);
#15073=FACE_OUTER_BOUND('',#17785,.T.);
#15074=FACE_OUTER_BOUND('',#17786,.T.);
#15075=FACE_OUTER_BOUND('',#17787,.T.);
#15076=FACE_OUTER_BOUND('',#17788,.T.);
#15077=FACE_OUTER_BOUND('',#17789,.T.);
#15078=FACE_OUTER_BOUND('',#17790,.T.);
#15079=FACE_OUTER_BOUND('',#17791,.T.);
#15080=FACE_OUTER_BOUND('',#17792,.T.);
#15081=FACE_OUTER_BOUND('',#17793,.T.);
#15082=FACE_OUTER_BOUND('',#17794,.T.);
#15083=FACE_OUTER_BOUND('',#17795,.T.);
#15084=FACE_OUTER_BOUND('',#17796,.T.);
#15085=FACE_OUTER_BOUND('',#17797,.T.);
#15086=FACE_OUTER_BOUND('',#17798,.T.);
#15087=FACE_OUTER_BOUND('',#17799,.T.);
#15088=FACE_OUTER_BOUND('',#17800,.T.);
#15089=FACE_OUTER_BOUND('',#17801,.T.);
#15090=FACE_OUTER_BOUND('',#17802,.T.);
#15091=FACE_OUTER_BOUND('',#17803,.T.);
#15092=FACE_OUTER_BOUND('',#17804,.T.);
#15093=FACE_OUTER_BOUND('',#17805,.T.);
#15094=FACE_OUTER_BOUND('',#17806,.T.);
#15095=FACE_OUTER_BOUND('',#17807,.T.);
#15096=FACE_OUTER_BOUND('',#17808,.T.);
#15097=FACE_OUTER_BOUND('',#17809,.T.);
#15098=FACE_OUTER_BOUND('',#17810,.T.);
#15099=FACE_OUTER_BOUND('',#17811,.T.);
#15100=FACE_OUTER_BOUND('',#17812,.T.);
#15101=FACE_OUTER_BOUND('',#17813,.T.);
#15102=FACE_OUTER_BOUND('',#17814,.T.);
#15103=FACE_OUTER_BOUND('',#17815,.T.);
#15104=FACE_OUTER_BOUND('',#17816,.T.);
#15105=FACE_OUTER_BOUND('',#17817,.T.);
#15106=FACE_OUTER_BOUND('',#17818,.T.);
#15107=FACE_OUTER_BOUND('',#17819,.T.);
#15108=FACE_OUTER_BOUND('',#17820,.T.);
#15109=FACE_OUTER_BOUND('',#17821,.T.);
#15110=FACE_OUTER_BOUND('',#17822,.T.);
#15111=FACE_OUTER_BOUND('',#17823,.T.);
#15112=FACE_OUTER_BOUND('',#17824,.T.);
#15113=FACE_OUTER_BOUND('',#17825,.T.);
#15114=FACE_OUTER_BOUND('',#17826,.T.);
#15115=FACE_OUTER_BOUND('',#17827,.T.);
#15116=FACE_OUTER_BOUND('',#17828,.T.);
#15117=FACE_OUTER_BOUND('',#17829,.T.);
#15118=FACE_OUTER_BOUND('',#17830,.T.);
#15119=FACE_OUTER_BOUND('',#17831,.T.);
#15120=FACE_OUTER_BOUND('',#17832,.T.);
#15121=FACE_OUTER_BOUND('',#17833,.T.);
#15122=FACE_OUTER_BOUND('',#17834,.T.);
#15123=FACE_OUTER_BOUND('',#17835,.T.);
#15124=FACE_OUTER_BOUND('',#17836,.T.);
#15125=FACE_OUTER_BOUND('',#17837,.T.);
#15126=FACE_OUTER_BOUND('',#17838,.T.);
#15127=FACE_OUTER_BOUND('',#17839,.T.);
#15128=FACE_OUTER_BOUND('',#17840,.T.);
#15129=FACE_OUTER_BOUND('',#17841,.T.);
#15130=FACE_OUTER_BOUND('',#17842,.T.);
#15131=FACE_OUTER_BOUND('',#17843,.T.);
#15132=FACE_OUTER_BOUND('',#17844,.T.);
#15133=FACE_OUTER_BOUND('',#17845,.T.);
#15134=FACE_OUTER_BOUND('',#17846,.T.);
#15135=FACE_OUTER_BOUND('',#17847,.T.);
#15136=FACE_OUTER_BOUND('',#17848,.T.);
#15137=FACE_OUTER_BOUND('',#17849,.T.);
#15138=FACE_OUTER_BOUND('',#17850,.T.);
#15139=FACE_OUTER_BOUND('',#17851,.T.);
#15140=FACE_OUTER_BOUND('',#17852,.T.);
#15141=FACE_OUTER_BOUND('',#17853,.T.);
#15142=FACE_OUTER_BOUND('',#17854,.T.);
#15143=FACE_OUTER_BOUND('',#17855,.T.);
#15144=FACE_OUTER_BOUND('',#17856,.T.);
#15145=FACE_OUTER_BOUND('',#17857,.T.);
#15146=FACE_OUTER_BOUND('',#17858,.T.);
#15147=FACE_OUTER_BOUND('',#17859,.T.);
#15148=FACE_OUTER_BOUND('',#17860,.T.);
#15149=FACE_OUTER_BOUND('',#17861,.T.);
#15150=FACE_OUTER_BOUND('',#17862,.T.);
#15151=FACE_OUTER_BOUND('',#17863,.T.);
#15152=FACE_OUTER_BOUND('',#17864,.T.);
#15153=FACE_OUTER_BOUND('',#17865,.T.);
#15154=FACE_OUTER_BOUND('',#17866,.T.);
#15155=FACE_OUTER_BOUND('',#17867,.T.);
#15156=FACE_OUTER_BOUND('',#17868,.T.);
#15157=FACE_OUTER_BOUND('',#17869,.T.);
#15158=FACE_OUTER_BOUND('',#17870,.T.);
#15159=FACE_OUTER_BOUND('',#17871,.T.);
#15160=FACE_OUTER_BOUND('',#17872,.T.);
#15161=FACE_OUTER_BOUND('',#17873,.T.);
#15162=FACE_OUTER_BOUND('',#17874,.T.);
#15163=FACE_OUTER_BOUND('',#17875,.T.);
#15164=FACE_OUTER_BOUND('',#17876,.T.);
#15165=FACE_OUTER_BOUND('',#17877,.T.);
#15166=FACE_OUTER_BOUND('',#17878,.T.);
#15167=FACE_OUTER_BOUND('',#17879,.T.);
#15168=FACE_OUTER_BOUND('',#17880,.T.);
#15169=FACE_OUTER_BOUND('',#17881,.T.);
#15170=FACE_OUTER_BOUND('',#17882,.T.);
#15171=FACE_OUTER_BOUND('',#17883,.T.);
#15172=FACE_OUTER_BOUND('',#17884,.T.);
#15173=FACE_OUTER_BOUND('',#17885,.T.);
#15174=FACE_OUTER_BOUND('',#17886,.T.);
#15175=FACE_OUTER_BOUND('',#17887,.T.);
#15176=FACE_OUTER_BOUND('',#17888,.T.);
#15177=FACE_OUTER_BOUND('',#17889,.T.);
#15178=FACE_OUTER_BOUND('',#17890,.T.);
#15179=FACE_OUTER_BOUND('',#17891,.T.);
#15180=FACE_OUTER_BOUND('',#17892,.T.);
#15181=FACE_OUTER_BOUND('',#17893,.T.);
#15182=FACE_OUTER_BOUND('',#17894,.T.);
#15183=FACE_OUTER_BOUND('',#17895,.T.);
#15184=FACE_OUTER_BOUND('',#17896,.T.);
#15185=FACE_OUTER_BOUND('',#17897,.T.);
#15186=FACE_OUTER_BOUND('',#17898,.T.);
#15187=FACE_OUTER_BOUND('',#17899,.T.);
#15188=FACE_OUTER_BOUND('',#17900,.T.);
#15189=FACE_OUTER_BOUND('',#17901,.T.);
#15190=FACE_OUTER_BOUND('',#17902,.T.);
#15191=FACE_OUTER_BOUND('',#17903,.T.);
#15192=FACE_OUTER_BOUND('',#17904,.T.);
#15193=FACE_OUTER_BOUND('',#17905,.T.);
#15194=FACE_OUTER_BOUND('',#17906,.T.);
#15195=FACE_OUTER_BOUND('',#17907,.T.);
#15196=FACE_OUTER_BOUND('',#17908,.T.);
#15197=FACE_OUTER_BOUND('',#17909,.T.);
#15198=FACE_OUTER_BOUND('',#17910,.T.);
#15199=FACE_OUTER_BOUND('',#17911,.T.);
#15200=FACE_OUTER_BOUND('',#17912,.T.);
#15201=FACE_OUTER_BOUND('',#17913,.T.);
#15202=FACE_OUTER_BOUND('',#17914,.T.);
#15203=FACE_OUTER_BOUND('',#17915,.T.);
#15204=FACE_OUTER_BOUND('',#17916,.T.);
#15205=FACE_OUTER_BOUND('',#17917,.T.);
#15206=FACE_OUTER_BOUND('',#17918,.T.);
#15207=FACE_OUTER_BOUND('',#17919,.T.);
#15208=FACE_OUTER_BOUND('',#17920,.T.);
#15209=FACE_OUTER_BOUND('',#17921,.T.);
#15210=FACE_OUTER_BOUND('',#17922,.T.);
#15211=FACE_OUTER_BOUND('',#17923,.T.);
#15212=FACE_OUTER_BOUND('',#17924,.T.);
#15213=FACE_OUTER_BOUND('',#17925,.T.);
#15214=FACE_OUTER_BOUND('',#17926,.T.);
#15215=FACE_OUTER_BOUND('',#17927,.T.);
#15216=FACE_OUTER_BOUND('',#17928,.T.);
#15217=FACE_OUTER_BOUND('',#17929,.T.);
#15218=FACE_OUTER_BOUND('',#17930,.T.);
#15219=FACE_OUTER_BOUND('',#17931,.T.);
#15220=FACE_OUTER_BOUND('',#17932,.T.);
#15221=FACE_OUTER_BOUND('',#17933,.T.);
#15222=FACE_OUTER_BOUND('',#17934,.T.);
#15223=FACE_OUTER_BOUND('',#17935,.T.);
#15224=FACE_OUTER_BOUND('',#17936,.T.);
#15225=FACE_OUTER_BOUND('',#17937,.T.);
#15226=FACE_OUTER_BOUND('',#17938,.T.);
#15227=FACE_OUTER_BOUND('',#17939,.T.);
#15228=FACE_OUTER_BOUND('',#17940,.T.);
#15229=FACE_OUTER_BOUND('',#17941,.T.);
#15230=FACE_OUTER_BOUND('',#17942,.T.);
#15231=FACE_OUTER_BOUND('',#17943,.T.);
#15232=FACE_OUTER_BOUND('',#17944,.T.);
#15233=FACE_OUTER_BOUND('',#17945,.T.);
#15234=FACE_OUTER_BOUND('',#17946,.T.);
#15235=FACE_OUTER_BOUND('',#17947,.T.);
#15236=FACE_OUTER_BOUND('',#17948,.T.);
#15237=FACE_OUTER_BOUND('',#17949,.T.);
#15238=FACE_OUTER_BOUND('',#17950,.T.);
#15239=FACE_OUTER_BOUND('',#17951,.T.);
#15240=FACE_OUTER_BOUND('',#17952,.T.);
#15241=FACE_OUTER_BOUND('',#17953,.T.);
#15242=FACE_OUTER_BOUND('',#17954,.T.);
#15243=FACE_OUTER_BOUND('',#17955,.T.);
#15244=FACE_OUTER_BOUND('',#17956,.T.);
#15245=FACE_OUTER_BOUND('',#17957,.T.);
#15246=FACE_OUTER_BOUND('',#17958,.T.);
#15247=FACE_OUTER_BOUND('',#17959,.T.);
#15248=FACE_OUTER_BOUND('',#17960,.T.);
#15249=FACE_OUTER_BOUND('',#17961,.T.);
#15250=FACE_OUTER_BOUND('',#17962,.T.);
#15251=FACE_OUTER_BOUND('',#17963,.T.);
#15252=FACE_OUTER_BOUND('',#17964,.T.);
#15253=FACE_OUTER_BOUND('',#17965,.T.);
#15254=FACE_OUTER_BOUND('',#17966,.T.);
#15255=FACE_OUTER_BOUND('',#17967,.T.);
#15256=FACE_OUTER_BOUND('',#17968,.T.);
#15257=FACE_OUTER_BOUND('',#17969,.T.);
#15258=FACE_OUTER_BOUND('',#17970,.T.);
#15259=FACE_OUTER_BOUND('',#17971,.T.);
#15260=FACE_OUTER_BOUND('',#17972,.T.);
#15261=FACE_OUTER_BOUND('',#17973,.T.);
#15262=FACE_OUTER_BOUND('',#17974,.T.);
#15263=FACE_OUTER_BOUND('',#17975,.T.);
#15264=FACE_OUTER_BOUND('',#17976,.T.);
#15265=FACE_OUTER_BOUND('',#17977,.T.);
#15266=FACE_OUTER_BOUND('',#17978,.T.);
#15267=FACE_OUTER_BOUND('',#17979,.T.);
#15268=FACE_OUTER_BOUND('',#17980,.T.);
#15269=FACE_OUTER_BOUND('',#17981,.T.);
#15270=FACE_OUTER_BOUND('',#17982,.T.);
#15271=FACE_OUTER_BOUND('',#17983,.T.);
#15272=FACE_OUTER_BOUND('',#17984,.T.);
#15273=FACE_OUTER_BOUND('',#17985,.T.);
#15274=FACE_OUTER_BOUND('',#17986,.T.);
#15275=FACE_OUTER_BOUND('',#17987,.T.);
#15276=FACE_OUTER_BOUND('',#17988,.T.);
#15277=FACE_OUTER_BOUND('',#17989,.T.);
#15278=FACE_OUTER_BOUND('',#17990,.T.);
#15279=FACE_OUTER_BOUND('',#17991,.T.);
#15280=FACE_OUTER_BOUND('',#17992,.T.);
#15281=FACE_OUTER_BOUND('',#17993,.T.);
#15282=FACE_OUTER_BOUND('',#17994,.T.);
#15283=FACE_OUTER_BOUND('',#17995,.T.);
#15284=FACE_OUTER_BOUND('',#17996,.T.);
#15285=FACE_OUTER_BOUND('',#17997,.T.);
#15286=FACE_OUTER_BOUND('',#17998,.T.);
#15287=FACE_OUTER_BOUND('',#17999,.T.);
#15288=FACE_OUTER_BOUND('',#18000,.T.);
#15289=FACE_OUTER_BOUND('',#18001,.T.);
#15290=FACE_OUTER_BOUND('',#18002,.T.);
#15291=FACE_OUTER_BOUND('',#18003,.T.);
#15292=FACE_OUTER_BOUND('',#18004,.T.);
#15293=FACE_OUTER_BOUND('',#18005,.T.);
#15294=FACE_OUTER_BOUND('',#18006,.T.);
#15295=FACE_OUTER_BOUND('',#18007,.T.);
#15296=FACE_OUTER_BOUND('',#18008,.T.);
#15297=FACE_OUTER_BOUND('',#18009,.T.);
#15298=FACE_OUTER_BOUND('',#18010,.T.);
#15299=FACE_OUTER_BOUND('',#18011,.T.);
#15300=FACE_OUTER_BOUND('',#18012,.T.);
#15301=FACE_OUTER_BOUND('',#18013,.T.);
#15302=FACE_OUTER_BOUND('',#18014,.T.);
#15303=FACE_OUTER_BOUND('',#18015,.T.);
#15304=FACE_OUTER_BOUND('',#18016,.T.);
#15305=FACE_OUTER_BOUND('',#18017,.T.);
#15306=FACE_OUTER_BOUND('',#18018,.T.);
#15307=FACE_OUTER_BOUND('',#18019,.T.);
#15308=FACE_OUTER_BOUND('',#18020,.T.);
#15309=FACE_OUTER_BOUND('',#18021,.T.);
#15310=FACE_OUTER_BOUND('',#18022,.T.);
#15311=FACE_OUTER_BOUND('',#18023,.T.);
#15312=FACE_OUTER_BOUND('',#18024,.T.);
#15313=FACE_OUTER_BOUND('',#18025,.T.);
#15314=FACE_OUTER_BOUND('',#18026,.T.);
#15315=FACE_OUTER_BOUND('',#18027,.T.);
#15316=FACE_OUTER_BOUND('',#18028,.T.);
#15317=FACE_OUTER_BOUND('',#18029,.T.);
#15318=FACE_OUTER_BOUND('',#18030,.T.);
#15319=FACE_OUTER_BOUND('',#18031,.T.);
#15320=FACE_OUTER_BOUND('',#18032,.T.);
#15321=FACE_OUTER_BOUND('',#18033,.T.);
#15322=FACE_OUTER_BOUND('',#18034,.T.);
#15323=FACE_OUTER_BOUND('',#18035,.T.);
#15324=FACE_OUTER_BOUND('',#18036,.T.);
#15325=FACE_OUTER_BOUND('',#18037,.T.);
#15326=FACE_OUTER_BOUND('',#18038,.T.);
#15327=FACE_OUTER_BOUND('',#18039,.T.);
#15328=FACE_OUTER_BOUND('',#18040,.T.);
#15329=FACE_OUTER_BOUND('',#18041,.T.);
#15330=FACE_OUTER_BOUND('',#18042,.T.);
#15331=FACE_OUTER_BOUND('',#18043,.T.);
#15332=FACE_OUTER_BOUND('',#18044,.T.);
#15333=FACE_OUTER_BOUND('',#18045,.T.);
#15334=FACE_OUTER_BOUND('',#18046,.T.);
#15335=FACE_OUTER_BOUND('',#18047,.T.);
#15336=FACE_OUTER_BOUND('',#18048,.T.);
#15337=FACE_OUTER_BOUND('',#18049,.T.);
#15338=FACE_OUTER_BOUND('',#18050,.T.);
#15339=FACE_OUTER_BOUND('',#18051,.T.);
#15340=FACE_OUTER_BOUND('',#18052,.T.);
#15341=FACE_OUTER_BOUND('',#18053,.T.);
#15342=FACE_OUTER_BOUND('',#18054,.T.);
#15343=FACE_OUTER_BOUND('',#18055,.T.);
#15344=FACE_OUTER_BOUND('',#18056,.T.);
#15345=FACE_OUTER_BOUND('',#18057,.T.);
#15346=FACE_OUTER_BOUND('',#18058,.T.);
#15347=FACE_OUTER_BOUND('',#18059,.T.);
#15348=FACE_OUTER_BOUND('',#18060,.T.);
#15349=FACE_OUTER_BOUND('',#18061,.T.);
#15350=FACE_OUTER_BOUND('',#18085,.T.);
#15351=FACE_OUTER_BOUND('',#18086,.T.);
#15352=FACE_OUTER_BOUND('',#18087,.T.);
#15353=FACE_OUTER_BOUND('',#18100,.T.);
#15354=FACE_OUTER_BOUND('',#18101,.T.);
#15355=FACE_OUTER_BOUND('',#18106,.T.);
#15356=FACE_OUTER_BOUND('',#18107,.T.);
#15357=FACE_OUTER_BOUND('',#18108,.T.);
#15358=FACE_OUTER_BOUND('',#18109,.T.);
#15359=FACE_OUTER_BOUND('',#18110,.T.);
#15360=FACE_OUTER_BOUND('',#18111,.T.);
#15361=FACE_OUTER_BOUND('',#18112,.T.);
#15362=FACE_OUTER_BOUND('',#18113,.T.);
#15363=FACE_OUTER_BOUND('',#18114,.T.);
#15364=FACE_OUTER_BOUND('',#18115,.T.);
#15365=FACE_OUTER_BOUND('',#18116,.T.);
#15366=FACE_OUTER_BOUND('',#18117,.T.);
#15367=FACE_OUTER_BOUND('',#18118,.T.);
#15368=FACE_OUTER_BOUND('',#18119,.T.);
#15369=FACE_OUTER_BOUND('',#18120,.T.);
#15370=FACE_OUTER_BOUND('',#18121,.T.);
#15371=FACE_OUTER_BOUND('',#18122,.T.);
#15372=FACE_OUTER_BOUND('',#18123,.T.);
#15373=FACE_OUTER_BOUND('',#18124,.T.);
#15374=FACE_OUTER_BOUND('',#18125,.T.);
#15375=FACE_OUTER_BOUND('',#18126,.T.);
#15376=FACE_OUTER_BOUND('',#18127,.T.);
#15377=FACE_OUTER_BOUND('',#18128,.T.);
#15378=FACE_OUTER_BOUND('',#18129,.T.);
#15379=FACE_OUTER_BOUND('',#18130,.T.);
#15380=FACE_OUTER_BOUND('',#18131,.T.);
#15381=FACE_OUTER_BOUND('',#18132,.T.);
#15382=FACE_OUTER_BOUND('',#18133,.T.);
#15383=FACE_OUTER_BOUND('',#18134,.T.);
#15384=FACE_OUTER_BOUND('',#18135,.T.);
#15385=FACE_OUTER_BOUND('',#18136,.T.);
#15386=FACE_OUTER_BOUND('',#18137,.T.);
#15387=FACE_OUTER_BOUND('',#18138,.T.);
#15388=FACE_OUTER_BOUND('',#18139,.T.);
#15389=FACE_OUTER_BOUND('',#18140,.T.);
#15390=FACE_OUTER_BOUND('',#18141,.T.);
#15391=FACE_OUTER_BOUND('',#18142,.T.);
#15392=FACE_OUTER_BOUND('',#18143,.T.);
#15393=FACE_OUTER_BOUND('',#18144,.T.);
#15394=FACE_OUTER_BOUND('',#18145,.T.);
#15395=FACE_OUTER_BOUND('',#18146,.T.);
#15396=FACE_OUTER_BOUND('',#18147,.T.);
#15397=FACE_OUTER_BOUND('',#18148,.T.);
#15398=FACE_OUTER_BOUND('',#18149,.T.);
#15399=FACE_OUTER_BOUND('',#18150,.T.);
#15400=FACE_OUTER_BOUND('',#18151,.T.);
#15401=FACE_OUTER_BOUND('',#18152,.T.);
#15402=FACE_OUTER_BOUND('',#18153,.T.);
#15403=FACE_OUTER_BOUND('',#18154,.T.);
#15404=FACE_OUTER_BOUND('',#18155,.T.);
#15405=FACE_OUTER_BOUND('',#18156,.T.);
#17745=EDGE_LOOP('',(#43479,#43480,#43481,#43482));
#17746=EDGE_LOOP('',(#43483,#43484,#43485,#43486));
#17747=EDGE_LOOP('',(#43487,#43488,#43489,#43490));
#17748=EDGE_LOOP('',(#43491,#43492,#43493,#43494));
#17749=EDGE_LOOP('',(#43495,#43496,#43497,#43498));
#17750=EDGE_LOOP('',(#43499,#43500,#43501,#43502));
#17751=EDGE_LOOP('',(#43503,#43504,#43505,#43506));
#17752=EDGE_LOOP('',(#43507,#43508,#43509,#43510));
#17753=EDGE_LOOP('',(#43511,#43512,#43513,#43514));
#17754=EDGE_LOOP('',(#43515,#43516,#43517,#43518));
#17755=EDGE_LOOP('',(#43519,#43520,#43521,#43522));
#17756=EDGE_LOOP('',(#43523,#43524,#43525,#43526));
#17757=EDGE_LOOP('',(#43527,#43528,#43529,#43530,#43531,#43532,#43533,#43534,
#43535,#43536,#43537,#43538));
#17758=EDGE_LOOP('',(#43539,#43540,#43541,#43542));
#17759=EDGE_LOOP('',(#43543,#43544,#43545,#43546));
#17760=EDGE_LOOP('',(#43547,#43548,#43549,#43550));
#17761=EDGE_LOOP('',(#43551,#43552,#43553,#43554));
#17762=EDGE_LOOP('',(#43555,#43556,#43557,#43558));
#17763=EDGE_LOOP('',(#43559,#43560,#43561,#43562));
#17764=EDGE_LOOP('',(#43563,#43564,#43565,#43566));
#17765=EDGE_LOOP('',(#43567,#43568,#43569,#43570));
#17766=EDGE_LOOP('',(#43571,#43572,#43573,#43574));
#17767=EDGE_LOOP('',(#43575,#43576,#43577,#43578));
#17768=EDGE_LOOP('',(#43579,#43580,#43581,#43582));
#17769=EDGE_LOOP('',(#43583,#43584,#43585,#43586));
#17770=EDGE_LOOP('',(#43587,#43588,#43589,#43590));
#17771=EDGE_LOOP('',(#43591,#43592,#43593,#43594));
#17772=EDGE_LOOP('',(#43595,#43596,#43597,#43598));
#17773=EDGE_LOOP('',(#43599,#43600,#43601,#43602));
#17774=EDGE_LOOP('',(#43603,#43604,#43605,#43606));
#17775=EDGE_LOOP('',(#43607,#43608,#43609,#43610));
#17776=EDGE_LOOP('',(#43611,#43612,#43613,#43614));
#17777=EDGE_LOOP('',(#43615,#43616,#43617,#43618));
#17778=EDGE_LOOP('',(#43619,#43620,#43621,#43622));
#17779=EDGE_LOOP('',(#43623,#43624,#43625,#43626));
#17780=EDGE_LOOP('',(#43627,#43628,#43629,#43630));
#17781=EDGE_LOOP('',(#43631,#43632,#43633,#43634));
#17782=EDGE_LOOP('',(#43635,#43636,#43637,#43638));
#17783=EDGE_LOOP('',(#43639,#43640,#43641,#43642));
#17784=EDGE_LOOP('',(#43643,#43644,#43645,#43646));
#17785=EDGE_LOOP('',(#43647,#43648,#43649,#43650));
#17786=EDGE_LOOP('',(#43651,#43652,#43653,#43654));
#17787=EDGE_LOOP('',(#43655,#43656,#43657,#43658));
#17788=EDGE_LOOP('',(#43659,#43660,#43661,#43662));
#17789=EDGE_LOOP('',(#43663,#43664,#43665,#43666));
#17790=EDGE_LOOP('',(#43667,#43668,#43669,#43670));
#17791=EDGE_LOOP('',(#43671,#43672,#43673,#43674));
#17792=EDGE_LOOP('',(#43675,#43676,#43677,#43678));
#17793=EDGE_LOOP('',(#43679,#43680,#43681,#43682));
#17794=EDGE_LOOP('',(#43683,#43684,#43685,#43686));
#17795=EDGE_LOOP('',(#43687,#43688,#43689,#43690));
#17796=EDGE_LOOP('',(#43691,#43692,#43693,#43694));
#17797=EDGE_LOOP('',(#43695,#43696,#43697,#43698));
#17798=EDGE_LOOP('',(#43699,#43700,#43701,#43702,#43703,#43704,#43705,#43706,
#43707,#43708,#43709,#43710,#43711,#43712,#43713,#43714,#43715,#43716,#43717,
#43718,#43719,#43720,#43721,#43722,#43723,#43724,#43725,#43726,#43727,#43728,
#43729,#43730,#43731,#43732,#43733));
#17799=EDGE_LOOP('',(#43734,#43735,#43736,#43737));
#17800=EDGE_LOOP('',(#43738,#43739,#43740,#43741));
#17801=EDGE_LOOP('',(#43742,#43743,#43744,#43745));
#17802=EDGE_LOOP('',(#43746,#43747,#43748,#43749));
#17803=EDGE_LOOP('',(#43750,#43751,#43752,#43753));
#17804=EDGE_LOOP('',(#43754,#43755,#43756,#43757));
#17805=EDGE_LOOP('',(#43758,#43759,#43760,#43761));
#17806=EDGE_LOOP('',(#43762,#43763,#43764,#43765));
#17807=EDGE_LOOP('',(#43766,#43767,#43768,#43769));
#17808=EDGE_LOOP('',(#43770,#43771,#43772,#43773));
#17809=EDGE_LOOP('',(#43774,#43775,#43776,#43777));
#17810=EDGE_LOOP('',(#43778,#43779,#43780,#43781));
#17811=EDGE_LOOP('',(#43782,#43783,#43784,#43785));
#17812=EDGE_LOOP('',(#43786,#43787,#43788,#43789));
#17813=EDGE_LOOP('',(#43790,#43791,#43792,#43793));
#17814=EDGE_LOOP('',(#43794,#43795,#43796,#43797));
#17815=EDGE_LOOP('',(#43798,#43799,#43800,#43801));
#17816=EDGE_LOOP('',(#43802,#43803,#43804,#43805));
#17817=EDGE_LOOP('',(#43806,#43807,#43808,#43809));
#17818=EDGE_LOOP('',(#43810,#43811,#43812,#43813));
#17819=EDGE_LOOP('',(#43814,#43815,#43816,#43817));
#17820=EDGE_LOOP('',(#43818,#43819,#43820,#43821));
#17821=EDGE_LOOP('',(#43822,#43823,#43824,#43825,#43826,#43827,#43828,#43829,
#43830,#43831,#43832,#43833,#43834,#43835,#43836,#43837,#43838,#43839,#43840,
#43841,#43842,#43843));
#17822=EDGE_LOOP('',(#43844,#43845,#43846,#43847));
#17823=EDGE_LOOP('',(#43848,#43849,#43850,#43851));
#17824=EDGE_LOOP('',(#43852,#43853,#43854,#43855));
#17825=EDGE_LOOP('',(#43856,#43857,#43858,#43859));
#17826=EDGE_LOOP('',(#43860,#43861,#43862,#43863));
#17827=EDGE_LOOP('',(#43864,#43865,#43866,#43867));
#17828=EDGE_LOOP('',(#43868,#43869,#43870,#43871,#43872,#43873));
#17829=EDGE_LOOP('',(#43874,#43875,#43876,#43877));
#17830=EDGE_LOOP('',(#43878,#43879,#43880,#43881));
#17831=EDGE_LOOP('',(#43882,#43883,#43884,#43885));
#17832=EDGE_LOOP('',(#43886,#43887,#43888,#43889));
#17833=EDGE_LOOP('',(#43890,#43891,#43892,#43893));
#17834=EDGE_LOOP('',(#43894,#43895,#43896,#43897));
#17835=EDGE_LOOP('',(#43898,#43899,#43900,#43901));
#17836=EDGE_LOOP('',(#43902,#43903,#43904,#43905));
#17837=EDGE_LOOP('',(#43906,#43907,#43908,#43909,#43910,#43911,#43912,#43913));
#17838=EDGE_LOOP('',(#43914,#43915,#43916,#43917));
#17839=EDGE_LOOP('',(#43918,#43919,#43920,#43921));
#17840=EDGE_LOOP('',(#43922,#43923,#43924,#43925));
#17841=EDGE_LOOP('',(#43926,#43927,#43928,#43929));
#17842=EDGE_LOOP('',(#43930,#43931,#43932,#43933));
#17843=EDGE_LOOP('',(#43934,#43935,#43936,#43937));
#17844=EDGE_LOOP('',(#43938,#43939,#43940,#43941));
#17845=EDGE_LOOP('',(#43942,#43943,#43944,#43945));
#17846=EDGE_LOOP('',(#43946,#43947,#43948,#43949));
#17847=EDGE_LOOP('',(#43950,#43951,#43952,#43953));
#17848=EDGE_LOOP('',(#43954,#43955,#43956,#43957));
#17849=EDGE_LOOP('',(#43958,#43959,#43960,#43961));
#17850=EDGE_LOOP('',(#43962,#43963,#43964,#43965));
#17851=EDGE_LOOP('',(#43966,#43967,#43968,#43969));
#17852=EDGE_LOOP('',(#43970,#43971,#43972,#43973));
#17853=EDGE_LOOP('',(#43974,#43975,#43976,#43977));
#17854=EDGE_LOOP('',(#43978,#43979,#43980,#43981));
#17855=EDGE_LOOP('',(#43982,#43983,#43984,#43985,#43986,#43987,#43988,#43989,
#43990,#43991,#43992,#43993,#43994,#43995,#43996,#43997,#43998));
#17856=EDGE_LOOP('',(#43999,#44000,#44001,#44002));
#17857=EDGE_LOOP('',(#44003,#44004,#44005,#44006));
#17858=EDGE_LOOP('',(#44007,#44008,#44009,#44010));
#17859=EDGE_LOOP('',(#44011,#44012,#44013,#44014));
#17860=EDGE_LOOP('',(#44015,#44016,#44017,#44018));
#17861=EDGE_LOOP('',(#44019,#44020,#44021,#44022));
#17862=EDGE_LOOP('',(#44023,#44024,#44025,#44026));
#17863=EDGE_LOOP('',(#44027,#44028,#44029,#44030));
#17864=EDGE_LOOP('',(#44031,#44032,#44033,#44034));
#17865=EDGE_LOOP('',(#44035,#44036,#44037,#44038));
#17866=EDGE_LOOP('',(#44039,#44040,#44041,#44042));
#17867=EDGE_LOOP('',(#44043,#44044,#44045,#44046));
#17868=EDGE_LOOP('',(#44047,#44048,#44049,#44050));
#17869=EDGE_LOOP('',(#44051,#44052,#44053,#44054));
#17870=EDGE_LOOP('',(#44055,#44056,#44057,#44058));
#17871=EDGE_LOOP('',(#44059,#44060,#44061,#44062));
#17872=EDGE_LOOP('',(#44063,#44064,#44065,#44066));
#17873=EDGE_LOOP('',(#44067,#44068,#44069,#44070));
#17874=EDGE_LOOP('',(#44071,#44072,#44073,#44074));
#17875=EDGE_LOOP('',(#44075,#44076,#44077,#44078,#44079,#44080,#44081,#44082,
#44083,#44084,#44085,#44086,#44087,#44088,#44089,#44090,#44091,#44092,#44093));
#17876=EDGE_LOOP('',(#44094,#44095,#44096,#44097));
#17877=EDGE_LOOP('',(#44098,#44099,#44100,#44101));
#17878=EDGE_LOOP('',(#44102,#44103,#44104,#44105));
#17879=EDGE_LOOP('',(#44106,#44107,#44108,#44109));
#17880=EDGE_LOOP('',(#44110,#44111,#44112,#44113));
#17881=EDGE_LOOP('',(#44114,#44115,#44116,#44117));
#17882=EDGE_LOOP('',(#44118,#44119,#44120,#44121));
#17883=EDGE_LOOP('',(#44122,#44123,#44124,#44125));
#17884=EDGE_LOOP('',(#44126,#44127,#44128,#44129,#44130,#44131,#44132,#44133));
#17885=EDGE_LOOP('',(#44134,#44135,#44136,#44137));
#17886=EDGE_LOOP('',(#44138,#44139,#44140,#44141));
#17887=EDGE_LOOP('',(#44142,#44143,#44144,#44145));
#17888=EDGE_LOOP('',(#44146,#44147,#44148,#44149));
#17889=EDGE_LOOP('',(#44150,#44151,#44152,#44153));
#17890=EDGE_LOOP('',(#44154,#44155,#44156,#44157));
#17891=EDGE_LOOP('',(#44158,#44159,#44160,#44161));
#17892=EDGE_LOOP('',(#44162,#44163,#44164,#44165));
#17893=EDGE_LOOP('',(#44166,#44167,#44168,#44169));
#17894=EDGE_LOOP('',(#44170,#44171,#44172,#44173,#44174,#44175,#44176,#44177,
#44178));
#17895=EDGE_LOOP('',(#44179,#44180,#44181,#44182));
#17896=EDGE_LOOP('',(#44183,#44184,#44185,#44186));
#17897=EDGE_LOOP('',(#44187,#44188,#44189,#44190));
#17898=EDGE_LOOP('',(#44191,#44192,#44193,#44194));
#17899=EDGE_LOOP('',(#44195,#44196,#44197,#44198));
#17900=EDGE_LOOP('',(#44199,#44200,#44201,#44202));
#17901=EDGE_LOOP('',(#44203,#44204,#44205,#44206));
#17902=EDGE_LOOP('',(#44207,#44208,#44209,#44210));
#17903=EDGE_LOOP('',(#44211,#44212,#44213,#44214));
#17904=EDGE_LOOP('',(#44215,#44216,#44217,#44218));
#17905=EDGE_LOOP('',(#44219,#44220,#44221,#44222));
#17906=EDGE_LOOP('',(#44223,#44224,#44225,#44226));
#17907=EDGE_LOOP('',(#44227,#44228,#44229,#44230,#44231,#44232,#44233,#44234,
#44235,#44236,#44237,#44238));
#17908=EDGE_LOOP('',(#44239,#44240,#44241,#44242));
#17909=EDGE_LOOP('',(#44243,#44244,#44245,#44246));
#17910=EDGE_LOOP('',(#44247,#44248,#44249,#44250));
#17911=EDGE_LOOP('',(#44251,#44252,#44253,#44254));
#17912=EDGE_LOOP('',(#44255,#44256,#44257,#44258));
#17913=EDGE_LOOP('',(#44259,#44260,#44261,#44262));
#17914=EDGE_LOOP('',(#44263,#44264,#44265,#44266));
#17915=EDGE_LOOP('',(#44267,#44268,#44269,#44270));
#17916=EDGE_LOOP('',(#44271,#44272,#44273,#44274));
#17917=EDGE_LOOP('',(#44275,#44276,#44277,#44278,#44279,#44280,#44281,#44282,
#44283));
#17918=EDGE_LOOP('',(#44284,#44285,#44286,#44287));
#17919=EDGE_LOOP('',(#44288,#44289,#44290,#44291));
#17920=EDGE_LOOP('',(#44292,#44293,#44294,#44295));
#17921=EDGE_LOOP('',(#44296,#44297,#44298,#44299));
#17922=EDGE_LOOP('',(#44300,#44301,#44302,#44303));
#17923=EDGE_LOOP('',(#44304,#44305,#44306,#44307));
#17924=EDGE_LOOP('',(#44308,#44309,#44310,#44311));
#17925=EDGE_LOOP('',(#44312,#44313,#44314,#44315));
#17926=EDGE_LOOP('',(#44316,#44317,#44318,#44319));
#17927=EDGE_LOOP('',(#44320,#44321,#44322,#44323));
#17928=EDGE_LOOP('',(#44324,#44325,#44326,#44327));
#17929=EDGE_LOOP('',(#44328,#44329,#44330,#44331));
#17930=EDGE_LOOP('',(#44332,#44333,#44334,#44335));
#17931=EDGE_LOOP('',(#44336,#44337,#44338,#44339));
#17932=EDGE_LOOP('',(#44340,#44341,#44342,#44343));
#17933=EDGE_LOOP('',(#44344,#44345,#44346,#44347));
#17934=EDGE_LOOP('',(#44348,#44349,#44350,#44351));
#17935=EDGE_LOOP('',(#44352,#44353,#44354,#44355));
#17936=EDGE_LOOP('',(#44356,#44357,#44358,#44359));
#17937=EDGE_LOOP('',(#44360,#44361,#44362,#44363));
#17938=EDGE_LOOP('',(#44364,#44365,#44366,#44367));
#17939=EDGE_LOOP('',(#44368,#44369,#44370,#44371));
#17940=EDGE_LOOP('',(#44372,#44373,#44374,#44375));
#17941=EDGE_LOOP('',(#44376,#44377,#44378,#44379));
#17942=EDGE_LOOP('',(#44380,#44381,#44382,#44383));
#17943=EDGE_LOOP('',(#44384,#44385,#44386,#44387));
#17944=EDGE_LOOP('',(#44388,#44389,#44390,#44391));
#17945=EDGE_LOOP('',(#44392,#44393,#44394,#44395,#44396,#44397,#44398,#44399,
#44400,#44401,#44402,#44403,#44404,#44405,#44406,#44407,#44408,#44409,#44410,
#44411,#44412,#44413));
#17946=EDGE_LOOP('',(#44414,#44415,#44416,#44417));
#17947=EDGE_LOOP('',(#44418,#44419,#44420,#44421));
#17948=EDGE_LOOP('',(#44422,#44423,#44424,#44425));
#17949=EDGE_LOOP('',(#44426,#44427,#44428,#44429));
#17950=EDGE_LOOP('',(#44430,#44431,#44432,#44433));
#17951=EDGE_LOOP('',(#44434,#44435,#44436,#44437));
#17952=EDGE_LOOP('',(#44438,#44439,#44440,#44441));
#17953=EDGE_LOOP('',(#44442,#44443,#44444,#44445));
#17954=EDGE_LOOP('',(#44446,#44447,#44448,#44449));
#17955=EDGE_LOOP('',(#44450,#44451,#44452,#44453));
#17956=EDGE_LOOP('',(#44454,#44455,#44456,#44457));
#17957=EDGE_LOOP('',(#44458,#44459,#44460,#44461,#44462,#44463,#44464,#44465,
#44466,#44467,#44468));
#17958=EDGE_LOOP('',(#44469,#44470,#44471,#44472));
#17959=EDGE_LOOP('',(#44473,#44474,#44475,#44476));
#17960=EDGE_LOOP('',(#44477,#44478,#44479,#44480));
#17961=EDGE_LOOP('',(#44481,#44482,#44483,#44484));
#17962=EDGE_LOOP('',(#44485,#44486,#44487,#44488));
#17963=EDGE_LOOP('',(#44489,#44490,#44491,#44492));
#17964=EDGE_LOOP('',(#44493,#44494,#44495,#44496));
#17965=EDGE_LOOP('',(#44497,#44498,#44499,#44500));
#17966=EDGE_LOOP('',(#44501,#44502,#44503,#44504));
#17967=EDGE_LOOP('',(#44505,#44506,#44507,#44508));
#17968=EDGE_LOOP('',(#44509,#44510,#44511,#44512));
#17969=EDGE_LOOP('',(#44513,#44514,#44515,#44516));
#17970=EDGE_LOOP('',(#44517,#44518,#44519,#44520));
#17971=EDGE_LOOP('',(#44521,#44522,#44523,#44524));
#17972=EDGE_LOOP('',(#44525,#44526,#44527,#44528));
#17973=EDGE_LOOP('',(#44529,#44530,#44531,#44532,#44533,#44534,#44535,#44536,
#44537,#44538,#44539,#44540,#44541,#44542,#44543));
#17974=EDGE_LOOP('',(#44544,#44545,#44546,#44547));
#17975=EDGE_LOOP('',(#44548,#44549,#44550,#44551));
#17976=EDGE_LOOP('',(#44552,#44553,#44554,#44555));
#17977=EDGE_LOOP('',(#44556,#44557,#44558,#44559));
#17978=EDGE_LOOP('',(#44560,#44561,#44562,#44563));
#17979=EDGE_LOOP('',(#44564,#44565,#44566,#44567));
#17980=EDGE_LOOP('',(#44568,#44569,#44570,#44571));
#17981=EDGE_LOOP('',(#44572,#44573,#44574,#44575));
#17982=EDGE_LOOP('',(#44576,#44577,#44578,#44579));
#17983=EDGE_LOOP('',(#44580,#44581,#44582,#44583));
#17984=EDGE_LOOP('',(#44584,#44585,#44586,#44587));
#17985=EDGE_LOOP('',(#44588,#44589,#44590,#44591));
#17986=EDGE_LOOP('',(#44592,#44593,#44594,#44595,#44596,#44597,#44598,#44599,
#44600,#44601,#44602,#44603));
#17987=EDGE_LOOP('',(#44604,#44605,#44606,#44607));
#17988=EDGE_LOOP('',(#44608,#44609,#44610,#44611));
#17989=EDGE_LOOP('',(#44612,#44613,#44614,#44615));
#17990=EDGE_LOOP('',(#44616,#44617,#44618,#44619));
#17991=EDGE_LOOP('',(#44620,#44621,#44622,#44623));
#17992=EDGE_LOOP('',(#44624,#44625,#44626,#44627));
#17993=EDGE_LOOP('',(#44628,#44629,#44630,#44631));
#17994=EDGE_LOOP('',(#44632,#44633,#44634,#44635));
#17995=EDGE_LOOP('',(#44636,#44637,#44638,#44639));
#17996=EDGE_LOOP('',(#44640,#44641,#44642,#44643));
#17997=EDGE_LOOP('',(#44644,#44645,#44646,#44647));
#17998=EDGE_LOOP('',(#44648,#44649,#44650,#44651));
#17999=EDGE_LOOP('',(#44652,#44653,#44654,#44655));
#18000=EDGE_LOOP('',(#44656,#44657,#44658,#44659));
#18001=EDGE_LOOP('',(#44660,#44661,#44662,#44663));
#18002=EDGE_LOOP('',(#44664,#44665,#44666,#44667));
#18003=EDGE_LOOP('',(#44668,#44669,#44670,#44671,#44672,#44673,#44674,#44675,
#44676,#44677,#44678));
#18004=EDGE_LOOP('',(#44679,#44680,#44681,#44682));
#18005=EDGE_LOOP('',(#44683,#44684,#44685,#44686));
#18006=EDGE_LOOP('',(#44687,#44688,#44689,#44690));
#18007=EDGE_LOOP('',(#44691,#44692,#44693,#44694));
#18008=EDGE_LOOP('',(#44695,#44696,#44697,#44698));
#18009=EDGE_LOOP('',(#44699,#44700,#44701,#44702));
#18010=EDGE_LOOP('',(#44703,#44704,#44705,#44706));
#18011=EDGE_LOOP('',(#44707,#44708,#44709,#44710));
#18012=EDGE_LOOP('',(#44711,#44712,#44713,#44714));
#18013=EDGE_LOOP('',(#44715,#44716,#44717,#44718));
#18014=EDGE_LOOP('',(#44719,#44720,#44721,#44722));
#18015=EDGE_LOOP('',(#44723,#44724,#44725,#44726));
#18016=EDGE_LOOP('',(#44727,#44728,#44729,#44730,#44731,#44732,#44733,#44734,
#44735,#44736,#44737,#44738));
#18017=EDGE_LOOP('',(#44739,#44740,#44741,#44742));
#18018=EDGE_LOOP('',(#44743,#44744,#44745,#44746));
#18019=EDGE_LOOP('',(#44747,#44748,#44749,#44750));
#18020=EDGE_LOOP('',(#44751,#44752,#44753,#44754));
#18021=EDGE_LOOP('',(#44755,#44756,#44757,#44758));
#18022=EDGE_LOOP('',(#44759,#44760,#44761,#44762));
#18023=EDGE_LOOP('',(#44763,#44764,#44765,#44766,#44767,#44768));
#18024=EDGE_LOOP('',(#44769,#44770,#44771,#44772));
#18025=EDGE_LOOP('',(#44773,#44774,#44775,#44776));
#18026=EDGE_LOOP('',(#44777,#44778,#44779,#44780));
#18027=EDGE_LOOP('',(#44781,#44782,#44783,#44784));
#18028=EDGE_LOOP('',(#44785,#44786,#44787,#44788));
#18029=EDGE_LOOP('',(#44789,#44790,#44791,#44792));
#18030=EDGE_LOOP('',(#44793,#44794,#44795,#44796));
#18031=EDGE_LOOP('',(#44797,#44798,#44799,#44800));
#18032=EDGE_LOOP('',(#44801,#44802,#44803,#44804));
#18033=EDGE_LOOP('',(#44805,#44806,#44807,#44808));
#18034=EDGE_LOOP('',(#44809,#44810,#44811,#44812));
#18035=EDGE_LOOP('',(#44813,#44814,#44815,#44816));
#18036=EDGE_LOOP('',(#44817,#44818,#44819,#44820,#44821,#44822,#44823,#44824,
#44825,#44826,#44827,#44828));
#18037=EDGE_LOOP('',(#44829,#44830,#44831,#44832));
#18038=EDGE_LOOP('',(#44833,#44834,#44835,#44836));
#18039=EDGE_LOOP('',(#44837,#44838,#44839,#44840));
#18040=EDGE_LOOP('',(#44841,#44842,#44843,#44844));
#18041=EDGE_LOOP('',(#44845,#44846,#44847,#44848));
#18042=EDGE_LOOP('',(#44849,#44850,#44851,#44852));
#18043=EDGE_LOOP('',(#44853,#44854,#44855,#44856));
#18044=EDGE_LOOP('',(#44857,#44858,#44859,#44860));
#18045=EDGE_LOOP('',(#44861,#44862,#44863,#44864));
#18046=EDGE_LOOP('',(#44865,#44866,#44867,#44868));
#18047=EDGE_LOOP('',(#44869,#44870,#44871,#44872));
#18048=EDGE_LOOP('',(#44873,#44874,#44875,#44876));
#18049=EDGE_LOOP('',(#44877,#44878,#44879,#44880));
#18050=EDGE_LOOP('',(#44881,#44882,#44883,#44884));
#18051=EDGE_LOOP('',(#44885,#44886,#44887,#44888));
#18052=EDGE_LOOP('',(#44889,#44890,#44891,#44892));
#18053=EDGE_LOOP('',(#44893,#44894,#44895,#44896));
#18054=EDGE_LOOP('',(#44897,#44898,#44899,#44900));
#18055=EDGE_LOOP('',(#44901,#44902,#44903,#44904));
#18056=EDGE_LOOP('',(#44905,#44906,#44907,#44908,#44909,#44910,#44911,#44912,
#44913,#44914,#44915,#44916,#44917,#44918,#44919,#44920,#44921,#44922,#44923));
#18057=EDGE_LOOP('',(#44924,#44925,#44926,#44927));
#18058=EDGE_LOOP('',(#44928,#44929,#44930,#44931));
#18059=EDGE_LOOP('',(#44932,#44933,#44934,#44935));
#18060=EDGE_LOOP('',(#44936,#44937,#44938,#44939));
#18061=EDGE_LOOP('',(#44940,#44941,#44942,#44943));
#18062=EDGE_LOOP('',(#44944,#44945,#44946,#44947,#44948,#44949,#44950,#44951,
#44952,#44953,#44954,#44955,#44956,#44957,#44958,#44959,#44960,#44961,#44962));
#18063=EDGE_LOOP('',(#44963,#44964,#44965,#44966,#44967,#44968,#44969,#44970,
#44971,#44972,#44973,#44974));
#18064=EDGE_LOOP('',(#44975,#44976,#44977,#44978,#44979,#44980));
#18065=EDGE_LOOP('',(#44981,#44982,#44983,#44984,#44985,#44986,#44987,#44988,
#44989,#44990,#44991,#44992));
#18066=EDGE_LOOP('',(#44993,#44994,#44995,#44996,#44997,#44998,#44999,#45000,
#45001,#45002,#45003));
#18067=EDGE_LOOP('',(#45004,#45005,#45006,#45007));
#18068=EDGE_LOOP('',(#45008,#45009,#45010,#45011,#45012,#45013,#45014,#45015,
#45016,#45017,#45018,#45019));
#18069=EDGE_LOOP('',(#45020,#45021,#45022,#45023,#45024,#45025,#45026,#45027,
#45028,#45029,#45030,#45031,#45032,#45033,#45034));
#18070=EDGE_LOOP('',(#45035,#45036,#45037,#45038,#45039,#45040,#45041,#45042,
#45043,#45044,#45045));
#18071=EDGE_LOOP('',(#45046,#45047,#45048,#45049,#45050,#45051,#45052,#45053,
#45054,#45055,#45056,#45057,#45058,#45059,#45060,#45061,#45062,#45063,#45064,
#45065,#45066,#45067));
#18072=EDGE_LOOP('',(#45068,#45069,#45070,#45071));
#18073=EDGE_LOOP('',(#45072,#45073,#45074,#45075,#45076,#45077,#45078,#45079,
#45080));
#18074=EDGE_LOOP('',(#45081,#45082,#45083,#45084,#45085,#45086,#45087,#45088,
#45089,#45090,#45091,#45092));
#18075=EDGE_LOOP('',(#45093,#45094,#45095,#45096,#45097,#45098,#45099,#45100,
#45101));
#18076=EDGE_LOOP('',(#45102,#45103,#45104,#45105,#45106,#45107,#45108,#45109));
#18077=EDGE_LOOP('',(#45110,#45111,#45112,#45113,#45114,#45115,#45116,#45117,
#45118,#45119,#45120,#45121,#45122,#45123,#45124,#45125,#45126,#45127,#45128));
#18078=EDGE_LOOP('',(#45129,#45130,#45131,#45132,#45133,#45134,#45135,#45136,
#45137,#45138,#45139,#45140,#45141,#45142,#45143,#45144,#45145));
#18079=EDGE_LOOP('',(#45146,#45147,#45148,#45149,#45150,#45151,#45152,#45153));
#18080=EDGE_LOOP('',(#45154,#45155,#45156,#45157,#45158,#45159));
#18081=EDGE_LOOP('',(#45160,#45161,#45162,#45163,#45164,#45165,#45166,#45167,
#45168,#45169,#45170,#45171,#45172,#45173,#45174,#45175,#45176,#45177,#45178,
#45179,#45180,#45181));
#18082=EDGE_LOOP('',(#45182,#45183,#45184,#45185,#45186,#45187,#45188,#45189,
#45190,#45191,#45192,#45193,#45194,#45195,#45196,#45197,#45198,#45199,#45200,
#45201,#45202,#45203,#45204,#45205,#45206,#45207,#45208,#45209,#45210,#45211,
#45212,#45213,#45214,#45215,#45216));
#18083=EDGE_LOOP('',(#45217,#45218,#45219,#45220));
#18084=EDGE_LOOP('',(#45221,#45222,#45223,#45224,#45225,#45226,#45227,#45228,
#45229,#45230,#45231,#45232));
#18085=EDGE_LOOP('',(#45233,#45234,#45235,#45236));
#18086=EDGE_LOOP('',(#45237,#45238,#45239,#45240));
#18087=EDGE_LOOP('',(#45241,#45242,#45243,#45244,#45245,#45246,#45247,#45248));
#18088=EDGE_LOOP('',(#45249));
#18089=EDGE_LOOP('',(#45250));
#18090=EDGE_LOOP('',(#45251));
#18091=EDGE_LOOP('',(#45252));
#18092=EDGE_LOOP('',(#45253));
#18093=EDGE_LOOP('',(#45254));
#18094=EDGE_LOOP('',(#45255));
#18095=EDGE_LOOP('',(#45256));
#18096=EDGE_LOOP('',(#45257));
#18097=EDGE_LOOP('',(#45258));
#18098=EDGE_LOOP('',(#45259));
#18099=EDGE_LOOP('',(#45260,#45261,#45262,#45263));
#18100=EDGE_LOOP('',(#45264,#45265,#45266,#45267));
#18101=EDGE_LOOP('',(#45268,#45269,#45270,#45271,#45272,#45273,#45274,#45275));
#18102=EDGE_LOOP('',(#45276));
#18103=EDGE_LOOP('',(#45277));
#18104=EDGE_LOOP('',(#45278));
#18105=EDGE_LOOP('',(#45279));
#18106=EDGE_LOOP('',(#45280,#45281,#45282,#45283));
#18107=EDGE_LOOP('',(#45284,#45285,#45286,#45287));
#18108=EDGE_LOOP('',(#45288,#45289,#45290,#45291));
#18109=EDGE_LOOP('',(#45292,#45293,#45294,#45295));
#18110=EDGE_LOOP('',(#45296,#45297,#45298,#45299));
#18111=EDGE_LOOP('',(#45300,#45301,#45302,#45303));
#18112=EDGE_LOOP('',(#45304,#45305,#45306,#45307));
#18113=EDGE_LOOP('',(#45308,#45309,#45310,#45311));
#18114=EDGE_LOOP('',(#45312,#45313,#45314,#45315));
#18115=EDGE_LOOP('',(#45316,#45317,#45318));
#18116=EDGE_LOOP('',(#45319,#45320,#45321,#45322));
#18117=EDGE_LOOP('',(#45323,#45324,#45325));
#18118=EDGE_LOOP('',(#45326,#45327,#45328,#45329));
#18119=EDGE_LOOP('',(#45330,#45331,#45332));
#18120=EDGE_LOOP('',(#45333,#45334,#45335,#45336));
#18121=EDGE_LOOP('',(#45337,#45338,#45339,#45340));
#18122=EDGE_LOOP('',(#45341,#45342,#45343));
#18123=EDGE_LOOP('',(#45344,#45345,#45346,#45347));
#18124=EDGE_LOOP('',(#45348,#45349,#45350,#45351));
#18125=EDGE_LOOP('',(#45352,#45353,#45354));
#18126=EDGE_LOOP('',(#45355,#45356,#45357,#45358));
#18127=EDGE_LOOP('',(#45359,#45360,#45361,#45362));
#18128=EDGE_LOOP('',(#45363,#45364,#45365));
#18129=EDGE_LOOP('',(#45366,#45367,#45368,#45369));
#18130=EDGE_LOOP('',(#45370,#45371,#45372,#45373));
#18131=EDGE_LOOP('',(#45374,#45375,#45376,#45377));
#18132=EDGE_LOOP('',(#45378));
#18133=EDGE_LOOP('',(#45379,#45380,#45381,#45382));
#18134=EDGE_LOOP('',(#45383,#45384,#45385,#45386));
#18135=EDGE_LOOP('',(#45387,#45388,#45389,#45390));
#18136=EDGE_LOOP('',(#45391,#45392,#45393,#45394));
#18137=EDGE_LOOP('',(#45395,#45396,#45397,#45398));
#18138=EDGE_LOOP('',(#45399,#45400,#45401,#45402));
#18139=EDGE_LOOP('',(#45403,#45404,#45405,#45406));
#18140=EDGE_LOOP('',(#45407,#45408,#45409,#45410));
#18141=EDGE_LOOP('',(#45411,#45412,#45413,#45414));
#18142=EDGE_LOOP('',(#45415,#45416,#45417,#45418));
#18143=EDGE_LOOP('',(#45419,#45420,#45421,#45422));
#18144=EDGE_LOOP('',(#45423,#45424,#45425,#45426));
#18145=EDGE_LOOP('',(#45427,#45428,#45429,#45430));
#18146=EDGE_LOOP('',(#45431,#45432,#45433,#45434));
#18147=EDGE_LOOP('',(#45435,#45436,#45437,#45438));
#18148=EDGE_LOOP('',(#45439,#45440,#45441,#45442));
#18149=EDGE_LOOP('',(#45443,#45444,#45445,#45446));
#18150=EDGE_LOOP('',(#45447,#45448,#45449,#45450));
#18151=EDGE_LOOP('',(#45451,#45452,#45453,#45454));
#18152=EDGE_LOOP('',(#45455,#45456,#45457,#45458));
#18153=EDGE_LOOP('',(#45459,#45460,#45461,#45462));
#18154=EDGE_LOOP('',(#45463,#45464,#45465,#45466));
#18155=EDGE_LOOP('',(#45467,#45468,#45469,#45470));
#18156=EDGE_LOOP('',(#45471,#45472,#45473,#45474));
#19951=CIRCLE('',#54369,5.);
#19952=CIRCLE('',#54370,4.5);
#19953=CIRCLE('',#54372,4.5);
#19954=CIRCLE('',#54374,9.);
#19955=CIRCLE('',#54375,9.);
#19956=CIRCLE('',#54376,9.);
#19957=CIRCLE('',#54377,9.);
#19958=CIRCLE('',#54378,5.);
#19959=CIRCLE('',#54379,3.3);
#19960=CIRCLE('',#54380,3.3);
#19961=CIRCLE('',#54381,3.3);
#19962=CIRCLE('',#54382,3.3);
#19963=CIRCLE('',#54383,20.025);
#19964=CIRCLE('',#54384,3.);
#19965=CIRCLE('',#54385,3.);
#19966=CIRCLE('',#54386,5.);
#19967=CIRCLE('',#54387,5.);
#19968=CIRCLE('',#54389,5.);
#19969=CIRCLE('',#54391,9.5);
#19970=CIRCLE('',#54392,9.5);
#19971=CIRCLE('',#54393,9.5);
#19972=CIRCLE('',#54394,9.5);
#19973=CIRCLE('',#54395,5.);
#19974=CIRCLE('',#54396,5.);
#19975=CIRCLE('',#54397,5.);
#19976=CIRCLE('',#54399,4.5);
#19977=CIRCLE('',#54401,4.5);
#19978=CIRCLE('',#54404,4.5);
#19979=CIRCLE('',#54406,4.5);
#19980=CIRCLE('',#54409,4.5);
#19981=CIRCLE('',#54411,4.5);
#19982=CIRCLE('',#54414,3.);
#19983=CIRCLE('',#54417,3.);
#19984=CIRCLE('',#54420,3.05);
#19985=CIRCLE('',#54422,3.05);
#19986=CIRCLE('',#54425,3.05);
#19987=CIRCLE('',#54427,3.05);
#19988=CIRCLE('',#54430,3.05);
#19989=CIRCLE('',#54432,3.05);
#19990=CIRCLE('',#54435,3.05);
#19991=CIRCLE('',#54437,3.05);
#19992=CIRCLE('',#54440,20.025);
#19993=CIRCLE('',#54443,10.);
#19994=CIRCLE('',#54446,10.);
#19995=CIRCLE('',#54449,10.);
#19996=CIRCLE('',#54452,10.);
#19997=CIRCLE('',#54456,10.);
#19998=CIRCLE('',#54459,10.);
#19999=CIRCLE('',#54466,10.);
#20000=CIRCLE('',#54469,10.);
#23840=VERTEX_POINT('',#80528);
#23841=VERTEX_POINT('',#80529);
#23842=VERTEX_POINT('',#80531);
#23843=VERTEX_POINT('',#80533);
#23844=VERTEX_POINT('',#80537);
#23845=VERTEX_POINT('',#80539);
#23846=VERTEX_POINT('',#80543);
#23847=VERTEX_POINT('',#80545);
#23848=VERTEX_POINT('',#80549);
#23849=VERTEX_POINT('',#80551);
#23850=VERTEX_POINT('',#80555);
#23851=VERTEX_POINT('',#80557);
#23852=VERTEX_POINT('',#80561);
#23853=VERTEX_POINT('',#80563);
#23854=VERTEX_POINT('',#80567);
#23855=VERTEX_POINT('',#80569);
#23856=VERTEX_POINT('',#80573);
#23857=VERTEX_POINT('',#80575);
#23858=VERTEX_POINT('',#80579);
#23859=VERTEX_POINT('',#80581);
#23860=VERTEX_POINT('',#80585);
#23861=VERTEX_POINT('',#80587);
#23862=VERTEX_POINT('',#80591);
#23863=VERTEX_POINT('',#80593);
#23864=VERTEX_POINT('',#80601);
#23865=VERTEX_POINT('',#80602);
#23866=VERTEX_POINT('',#80604);
#23867=VERTEX_POINT('',#80606);
#23868=VERTEX_POINT('',#80610);
#23869=VERTEX_POINT('',#80612);
#23870=VERTEX_POINT('',#80616);
#23871=VERTEX_POINT('',#80618);
#23872=VERTEX_POINT('',#80631);
#23873=VERTEX_POINT('',#80632);
#23874=VERTEX_POINT('',#80636);
#23875=VERTEX_POINT('',#80638);
#23876=VERTEX_POINT('',#80649);
#23877=VERTEX_POINT('',#80653);
#23878=VERTEX_POINT('',#80664);
#23879=VERTEX_POINT('',#80668);
#23880=VERTEX_POINT('',#80679);
#23881=VERTEX_POINT('',#80683);
#23882=VERTEX_POINT('',#80694);
#23883=VERTEX_POINT('',#80698);
#23884=VERTEX_POINT('',#80709);
#23885=VERTEX_POINT('',#80713);
#23886=VERTEX_POINT('',#80724);
#23887=VERTEX_POINT('',#80728);
#23888=VERTEX_POINT('',#80739);
#23889=VERTEX_POINT('',#80743);
#23890=VERTEX_POINT('',#80754);
#23891=VERTEX_POINT('',#80758);
#23892=VERTEX_POINT('',#80769);
#23893=VERTEX_POINT('',#80773);
#23894=VERTEX_POINT('',#80784);
#23895=VERTEX_POINT('',#80788);
#23896=VERTEX_POINT('',#80799);
#23897=VERTEX_POINT('',#80803);
#23898=VERTEX_POINT('',#80814);
#23899=VERTEX_POINT('',#80818);
#23900=VERTEX_POINT('',#80824);
#23901=VERTEX_POINT('',#80826);
#23902=VERTEX_POINT('',#80835);
#23903=VERTEX_POINT('',#80839);
#23904=VERTEX_POINT('',#80850);
#23905=VERTEX_POINT('',#80854);
#23906=VERTEX_POINT('',#80865);
#23907=VERTEX_POINT('',#80869);
#23908=VERTEX_POINT('',#80880);
#23909=VERTEX_POINT('',#80884);
#23910=VERTEX_POINT('',#80895);
#23911=VERTEX_POINT('',#80899);
#23912=VERTEX_POINT('',#80910);
#23913=VERTEX_POINT('',#80914);
#23914=VERTEX_POINT('',#80925);
#23915=VERTEX_POINT('',#80929);
#23916=VERTEX_POINT('',#80940);
#23917=VERTEX_POINT('',#80944);
#23918=VERTEX_POINT('',#80955);
#23919=VERTEX_POINT('',#80959);
#23920=VERTEX_POINT('',#80970);
#23921=VERTEX_POINT('',#80974);
#23922=VERTEX_POINT('',#80985);
#23923=VERTEX_POINT('',#80989);
#23924=VERTEX_POINT('',#81000);
#23925=VERTEX_POINT('',#81004);
#23926=VERTEX_POINT('',#81015);
#23927=VERTEX_POINT('',#81019);
#23928=VERTEX_POINT('',#81030);
#23929=VERTEX_POINT('',#81034);
#23930=VERTEX_POINT('',#81045);
#23931=VERTEX_POINT('',#81049);
#23932=VERTEX_POINT('',#81060);
#23933=VERTEX_POINT('',#81064);
#23934=VERTEX_POINT('',#81075);
#23935=VERTEX_POINT('',#81079);
#23936=VERTEX_POINT('',#81090);
#23937=VERTEX_POINT('',#81094);
#23938=VERTEX_POINT('',#81100);
#23939=VERTEX_POINT('',#81102);
#23940=VERTEX_POINT('',#81111);
#23941=VERTEX_POINT('',#81115);
#23942=VERTEX_POINT('',#81139);
#23943=VERTEX_POINT('',#81140);
#23944=VERTEX_POINT('',#81144);
#23945=VERTEX_POINT('',#81146);
#23946=VERTEX_POINT('',#81157);
#23947=VERTEX_POINT('',#81161);
#23948=VERTEX_POINT('',#81172);
#23949=VERTEX_POINT('',#81176);
#23950=VERTEX_POINT('',#81187);
#23951=VERTEX_POINT('',#81191);
#23952=VERTEX_POINT('',#81202);
#23953=VERTEX_POINT('',#81206);
#23954=VERTEX_POINT('',#81217);
#23955=VERTEX_POINT('',#81221);
#23956=VERTEX_POINT('',#81232);
#23957=VERTEX_POINT('',#81236);
#23958=VERTEX_POINT('',#81247);
#23959=VERTEX_POINT('',#81251);
#23960=VERTEX_POINT('',#81257);
#23961=VERTEX_POINT('',#81259);
#23962=VERTEX_POINT('',#81268);
#23963=VERTEX_POINT('',#81272);
#23964=VERTEX_POINT('',#81283);
#23965=VERTEX_POINT('',#81287);
#23966=VERTEX_POINT('',#81298);
#23967=VERTEX_POINT('',#81302);
#23968=VERTEX_POINT('',#81313);
#23969=VERTEX_POINT('',#81317);
#23970=VERTEX_POINT('',#81328);
#23971=VERTEX_POINT('',#81332);
#23972=VERTEX_POINT('',#81343);
#23973=VERTEX_POINT('',#81347);
#23974=VERTEX_POINT('',#81358);
#23975=VERTEX_POINT('',#81362);
#23976=VERTEX_POINT('',#81373);
#23977=VERTEX_POINT('',#81377);
#23978=VERTEX_POINT('',#81388);
#23979=VERTEX_POINT('',#81392);
#23980=VERTEX_POINT('',#81403);
#23981=VERTEX_POINT('',#81407);
#23982=VERTEX_POINT('',#81413);
#23983=VERTEX_POINT('',#81415);
#23984=VERTEX_POINT('',#81424);
#23985=VERTEX_POINT('',#81428);
#23986=VERTEX_POINT('',#81447);
#23987=VERTEX_POINT('',#81448);
#23988=VERTEX_POINT('',#81450);
#23989=VERTEX_POINT('',#81452);
#23990=VERTEX_POINT('',#81456);
#23991=VERTEX_POINT('',#81458);
#23992=VERTEX_POINT('',#81462);
#23993=VERTEX_POINT('',#81464);
#23994=VERTEX_POINT('',#81468);
#23995=VERTEX_POINT('',#81470);
#23996=VERTEX_POINT('',#81474);
#23997=VERTEX_POINT('',#81476);
#23998=VERTEX_POINT('',#81484);
#23999=VERTEX_POINT('',#81485);
#24000=VERTEX_POINT('',#81487);
#24001=VERTEX_POINT('',#81489);
#24002=VERTEX_POINT('',#81493);
#24003=VERTEX_POINT('',#81495);
#24004=VERTEX_POINT('',#81499);
#24005=VERTEX_POINT('',#81501);
#24006=VERTEX_POINT('',#81505);
#24007=VERTEX_POINT('',#81507);
#24008=VERTEX_POINT('',#81511);
#24009=VERTEX_POINT('',#81513);
#24010=VERTEX_POINT('',#81517);
#24011=VERTEX_POINT('',#81519);
#24012=VERTEX_POINT('',#81523);
#24013=VERTEX_POINT('',#81525);
#24014=VERTEX_POINT('',#81538);
#24015=VERTEX_POINT('',#81539);
#24016=VERTEX_POINT('',#81543);
#24017=VERTEX_POINT('',#81545);
#24018=VERTEX_POINT('',#81556);
#24019=VERTEX_POINT('',#81560);
#24020=VERTEX_POINT('',#81571);
#24021=VERTEX_POINT('',#81575);
#24022=VERTEX_POINT('',#81586);
#24023=VERTEX_POINT('',#81590);
#24024=VERTEX_POINT('',#81596);
#24025=VERTEX_POINT('',#81598);
#24026=VERTEX_POINT('',#81602);
#24027=VERTEX_POINT('',#81604);
#24028=VERTEX_POINT('',#81608);
#24029=VERTEX_POINT('',#81610);
#24030=VERTEX_POINT('',#81619);
#24031=VERTEX_POINT('',#81623);
#24032=VERTEX_POINT('',#81634);
#24033=VERTEX_POINT('',#81638);
#24034=VERTEX_POINT('',#81649);
#24035=VERTEX_POINT('',#81653);
#24036=VERTEX_POINT('',#81664);
#24037=VERTEX_POINT('',#81668);
#24038=VERTEX_POINT('',#81679);
#24039=VERTEX_POINT('',#81683);
#24040=VERTEX_POINT('',#81694);
#24041=VERTEX_POINT('',#81698);
#24042=VERTEX_POINT('',#81704);
#24043=VERTEX_POINT('',#81706);
#24044=VERTEX_POINT('',#81710);
#24045=VERTEX_POINT('',#81712);
#24046=VERTEX_POINT('',#81716);
#24047=VERTEX_POINT('',#81718);
#24048=VERTEX_POINT('',#81735);
#24049=VERTEX_POINT('',#81736);
#24050=VERTEX_POINT('',#81738);
#24051=VERTEX_POINT('',#81740);
#24052=VERTEX_POINT('',#81749);
#24053=VERTEX_POINT('',#81753);
#24054=VERTEX_POINT('',#81764);
#24055=VERTEX_POINT('',#81768);
#24056=VERTEX_POINT('',#81779);
#24057=VERTEX_POINT('',#81783);
#24058=VERTEX_POINT('',#81794);
#24059=VERTEX_POINT('',#81798);
#24060=VERTEX_POINT('',#81804);
#24061=VERTEX_POINT('',#81806);
#24062=VERTEX_POINT('',#81810);
#24063=VERTEX_POINT('',#81812);
#24064=VERTEX_POINT('',#81816);
#24065=VERTEX_POINT('',#81818);
#24066=VERTEX_POINT('',#81827);
#24067=VERTEX_POINT('',#81831);
#24068=VERTEX_POINT('',#81842);
#24069=VERTEX_POINT('',#81846);
#24070=VERTEX_POINT('',#81857);
#24071=VERTEX_POINT('',#81861);
#24072=VERTEX_POINT('',#81872);
#24073=VERTEX_POINT('',#81876);
#24074=VERTEX_POINT('',#81887);
#24075=VERTEX_POINT('',#81891);
#24076=VERTEX_POINT('',#81902);
#24077=VERTEX_POINT('',#81906);
#24078=VERTEX_POINT('',#81917);
#24079=VERTEX_POINT('',#81921);
#24080=VERTEX_POINT('',#81927);
#24081=VERTEX_POINT('',#81929);
#24082=VERTEX_POINT('',#81933);
#24083=VERTEX_POINT('',#81935);
#24084=VERTEX_POINT('',#81939);
#24085=VERTEX_POINT('',#81941);
#24086=VERTEX_POINT('',#81949);
#24087=VERTEX_POINT('',#81950);
#24088=VERTEX_POINT('',#81952);
#24089=VERTEX_POINT('',#81954);
#24090=VERTEX_POINT('',#81958);
#24091=VERTEX_POINT('',#81960);
#24092=VERTEX_POINT('',#81964);
#24093=VERTEX_POINT('',#81966);
#24094=VERTEX_POINT('',#81970);
#24095=VERTEX_POINT('',#81972);
#24096=VERTEX_POINT('',#81976);
#24097=VERTEX_POINT('',#81978);
#24098=VERTEX_POINT('',#81982);
#24099=VERTEX_POINT('',#81984);
#24100=VERTEX_POINT('',#81988);
#24101=VERTEX_POINT('',#81990);
#24102=VERTEX_POINT('',#82003);
#24103=VERTEX_POINT('',#82004);
#24104=VERTEX_POINT('',#82008);
#24105=VERTEX_POINT('',#82010);
#24106=VERTEX_POINT('',#82021);
#24107=VERTEX_POINT('',#82025);
#24108=VERTEX_POINT('',#82031);
#24109=VERTEX_POINT('',#82033);
#24110=VERTEX_POINT('',#82042);
#24111=VERTEX_POINT('',#82046);
#24112=VERTEX_POINT('',#82057);
#24113=VERTEX_POINT('',#82061);
#24114=VERTEX_POINT('',#82067);
#24115=VERTEX_POINT('',#82069);
#24116=VERTEX_POINT('',#82073);
#24117=VERTEX_POINT('',#82075);
#24118=VERTEX_POINT('',#82079);
#24119=VERTEX_POINT('',#82081);
#24120=VERTEX_POINT('',#82094);
#24121=VERTEX_POINT('',#82095);
#24122=VERTEX_POINT('',#82099);
#24123=VERTEX_POINT('',#82101);
#24124=VERTEX_POINT('',#82112);
#24125=VERTEX_POINT('',#82116);
#24126=VERTEX_POINT('',#82127);
#24127=VERTEX_POINT('',#82131);
#24128=VERTEX_POINT('',#82142);
#24129=VERTEX_POINT('',#82146);
#24130=VERTEX_POINT('',#82157);
#24131=VERTEX_POINT('',#82161);
#24132=VERTEX_POINT('',#82172);
#24133=VERTEX_POINT('',#82176);
#24134=VERTEX_POINT('',#82187);
#24135=VERTEX_POINT('',#82191);
#24136=VERTEX_POINT('',#82202);
#24137=VERTEX_POINT('',#82206);
#24138=VERTEX_POINT('',#82217);
#24139=VERTEX_POINT('',#82221);
#24140=VERTEX_POINT('',#82232);
#24141=VERTEX_POINT('',#82236);
#24142=VERTEX_POINT('',#82247);
#24143=VERTEX_POINT('',#82251);
#24144=VERTEX_POINT('',#82275);
#24145=VERTEX_POINT('',#82276);
#24146=VERTEX_POINT('',#82280);
#24147=VERTEX_POINT('',#82282);
#24148=VERTEX_POINT('',#82293);
#24149=VERTEX_POINT('',#82297);
#24150=VERTEX_POINT('',#82303);
#24151=VERTEX_POINT('',#82305);
#24152=VERTEX_POINT('',#82314);
#24153=VERTEX_POINT('',#82318);
#24154=VERTEX_POINT('',#82329);
#24155=VERTEX_POINT('',#82333);
#24156=VERTEX_POINT('',#82339);
#24157=VERTEX_POINT('',#82341);
#24158=VERTEX_POINT('',#82345);
#24159=VERTEX_POINT('',#82347);
#24160=VERTEX_POINT('',#82351);
#24161=VERTEX_POINT('',#82353);
#24162=VERTEX_POINT('',#82361);
#24163=VERTEX_POINT('',#82362);
#24164=VERTEX_POINT('',#82364);
#24165=VERTEX_POINT('',#82366);
#24166=VERTEX_POINT('',#82370);
#24167=VERTEX_POINT('',#82372);
#24168=VERTEX_POINT('',#82376);
#24169=VERTEX_POINT('',#82378);
#24170=VERTEX_POINT('',#82391);
#24171=VERTEX_POINT('',#82392);
#24172=VERTEX_POINT('',#82396);
#24173=VERTEX_POINT('',#82398);
#24174=VERTEX_POINT('',#82409);
#24175=VERTEX_POINT('',#82413);
#24176=VERTEX_POINT('',#82424);
#24177=VERTEX_POINT('',#82428);
#24178=VERTEX_POINT('',#82439);
#24179=VERTEX_POINT('',#82443);
#24180=VERTEX_POINT('',#82454);
#24181=VERTEX_POINT('',#82458);
#24182=VERTEX_POINT('',#82464);
#24183=VERTEX_POINT('',#82466);
#24184=VERTEX_POINT('',#82470);
#24185=VERTEX_POINT('',#82472);
#24186=VERTEX_POINT('',#82476);
#24187=VERTEX_POINT('',#82478);
#24188=VERTEX_POINT('',#82482);
#24189=VERTEX_POINT('',#82484);
#24190=VERTEX_POINT('',#82488);
#24191=VERTEX_POINT('',#82490);
#24192=VERTEX_POINT('',#82494);
#24193=VERTEX_POINT('',#82496);
#24194=VERTEX_POINT('',#82505);
#24195=VERTEX_POINT('',#82509);
#24196=VERTEX_POINT('',#82520);
#24197=VERTEX_POINT('',#82524);
#24198=VERTEX_POINT('',#82535);
#24199=VERTEX_POINT('',#82539);
#24200=VERTEX_POINT('',#82550);
#24201=VERTEX_POINT('',#82554);
#24202=VERTEX_POINT('',#82565);
#24203=VERTEX_POINT('',#82569);
#24204=VERTEX_POINT('',#82580);
#24205=VERTEX_POINT('',#82584);
#24206=VERTEX_POINT('',#82595);
#24207=VERTEX_POINT('',#82599);
#24208=VERTEX_POINT('',#82610);
#24209=VERTEX_POINT('',#82614);
#24210=VERTEX_POINT('',#82620);
#24211=VERTEX_POINT('',#82622);
#24212=VERTEX_POINT('',#82631);
#24213=VERTEX_POINT('',#82635);
#24214=VERTEX_POINT('',#82659);
#24215=VERTEX_POINT('',#82660);
#24216=VERTEX_POINT('',#82664);
#24217=VERTEX_POINT('',#82666);
#24218=VERTEX_POINT('',#82677);
#24219=VERTEX_POINT('',#82681);
#24220=VERTEX_POINT('',#82692);
#24221=VERTEX_POINT('',#82696);
#24222=VERTEX_POINT('',#82707);
#24223=VERTEX_POINT('',#82711);
#24224=VERTEX_POINT('',#82722);
#24225=VERTEX_POINT('',#82726);
#24226=VERTEX_POINT('',#82737);
#24227=VERTEX_POINT('',#82741);
#24228=VERTEX_POINT('',#82752);
#24229=VERTEX_POINT('',#82756);
#24230=VERTEX_POINT('',#82767);
#24231=VERTEX_POINT('',#82771);
#24232=VERTEX_POINT('',#82782);
#24233=VERTEX_POINT('',#82786);
#24234=VERTEX_POINT('',#82797);
#24235=VERTEX_POINT('',#82801);
#24236=VERTEX_POINT('',#82825);
#24237=VERTEX_POINT('',#82826);
#24238=VERTEX_POINT('',#82830);
#24239=VERTEX_POINT('',#82832);
#24240=VERTEX_POINT('',#82843);
#24241=VERTEX_POINT('',#82847);
#24242=VERTEX_POINT('',#82858);
#24243=VERTEX_POINT('',#82862);
#24244=VERTEX_POINT('',#82873);
#24245=VERTEX_POINT('',#82877);
#24246=VERTEX_POINT('',#82888);
#24247=VERTEX_POINT('',#82892);
#24248=VERTEX_POINT('',#82903);
#24249=VERTEX_POINT('',#82907);
#24250=VERTEX_POINT('',#82918);
#24251=VERTEX_POINT('',#82922);
#24252=VERTEX_POINT('',#82933);
#24253=VERTEX_POINT('',#82937);
#24254=VERTEX_POINT('',#82948);
#24255=VERTEX_POINT('',#82952);
#24256=VERTEX_POINT('',#82963);
#24257=VERTEX_POINT('',#82967);
#24258=VERTEX_POINT('',#82978);
#24259=VERTEX_POINT('',#82982);
#24260=VERTEX_POINT('',#82988);
#24261=VERTEX_POINT('',#82990);
#24262=VERTEX_POINT('',#82999);
#24263=VERTEX_POINT('',#83003);
#24264=VERTEX_POINT('',#83014);
#24265=VERTEX_POINT('',#83018);
#24266=VERTEX_POINT('',#83037);
#24267=VERTEX_POINT('',#83038);
#24268=VERTEX_POINT('',#83040);
#24269=VERTEX_POINT('',#83042);
#24270=VERTEX_POINT('',#83046);
#24271=VERTEX_POINT('',#83048);
#24272=VERTEX_POINT('',#83052);
#24273=VERTEX_POINT('',#83054);
#24274=VERTEX_POINT('',#83058);
#24275=VERTEX_POINT('',#83060);
#24276=VERTEX_POINT('',#83064);
#24277=VERTEX_POINT('',#83066);
#24278=VERTEX_POINT('',#83070);
#24279=VERTEX_POINT('',#83072);
#24280=VERTEX_POINT('',#83076);
#24281=VERTEX_POINT('',#83078);
#24282=VERTEX_POINT('',#83082);
#24283=VERTEX_POINT('',#83084);
#24284=VERTEX_POINT('',#83088);
#24285=VERTEX_POINT('',#83090);
#24286=VERTEX_POINT('',#83094);
#24287=VERTEX_POINT('',#83096);
#24288=VERTEX_POINT('',#83100);
#24289=VERTEX_POINT('',#83102);
#24290=VERTEX_POINT('',#83110);
#24291=VERTEX_POINT('',#83111);
#24292=VERTEX_POINT('',#83113);
#24293=VERTEX_POINT('',#83115);
#24294=VERTEX_POINT('',#83119);
#24295=VERTEX_POINT('',#83121);
#24296=VERTEX_POINT('',#83125);
#24297=VERTEX_POINT('',#83127);
#24298=VERTEX_POINT('',#83140);
#24299=VERTEX_POINT('',#83141);
#24300=VERTEX_POINT('',#83145);
#24301=VERTEX_POINT('',#83147);
#24302=VERTEX_POINT('',#83158);
#24303=VERTEX_POINT('',#83162);
#24304=VERTEX_POINT('',#83173);
#24305=VERTEX_POINT('',#83177);
#24306=VERTEX_POINT('',#83188);
#24307=VERTEX_POINT('',#83192);
#24308=VERTEX_POINT('',#83203);
#24309=VERTEX_POINT('',#83207);
#24310=VERTEX_POINT('',#83218);
#24311=VERTEX_POINT('',#83222);
#24312=VERTEX_POINT('',#83233);
#24313=VERTEX_POINT('',#83237);
#24314=VERTEX_POINT('',#83248);
#24315=VERTEX_POINT('',#83252);
#24316=VERTEX_POINT('',#83263);
#24317=VERTEX_POINT('',#83267);
#24318=VERTEX_POINT('',#83278);
#24319=VERTEX_POINT('',#83282);
#24320=VERTEX_POINT('',#83301);
#24321=VERTEX_POINT('',#83302);
#24322=VERTEX_POINT('',#83304);
#24323=VERTEX_POINT('',#83306);
#24324=VERTEX_POINT('',#83310);
#24325=VERTEX_POINT('',#83312);
#24326=VERTEX_POINT('',#83316);
#24327=VERTEX_POINT('',#83318);
#24328=VERTEX_POINT('',#83322);
#24329=VERTEX_POINT('',#83324);
#24330=VERTEX_POINT('',#83328);
#24331=VERTEX_POINT('',#83330);
#24332=VERTEX_POINT('',#83334);
#24333=VERTEX_POINT('',#83336);
#24334=VERTEX_POINT('',#83340);
#24335=VERTEX_POINT('',#83342);
#24336=VERTEX_POINT('',#83346);
#24337=VERTEX_POINT('',#83348);
#24338=VERTEX_POINT('',#83352);
#24339=VERTEX_POINT('',#83354);
#24340=VERTEX_POINT('',#83358);
#24341=VERTEX_POINT('',#83360);
#24342=VERTEX_POINT('',#83364);
#24343=VERTEX_POINT('',#83366);
#24344=VERTEX_POINT('',#83374);
#24345=VERTEX_POINT('',#83375);
#24346=VERTEX_POINT('',#83377);
#24347=VERTEX_POINT('',#83379);
#24348=VERTEX_POINT('',#83383);
#24349=VERTEX_POINT('',#83385);
#24350=VERTEX_POINT('',#83389);
#24351=VERTEX_POINT('',#83391);
#24352=VERTEX_POINT('',#83395);
#24353=VERTEX_POINT('',#83397);
#24354=VERTEX_POINT('',#83401);
#24355=VERTEX_POINT('',#83403);
#24356=VERTEX_POINT('',#83416);
#24357=VERTEX_POINT('',#83417);
#24358=VERTEX_POINT('',#83421);
#24359=VERTEX_POINT('',#83423);
#24360=VERTEX_POINT('',#83434);
#24361=VERTEX_POINT('',#83438);
#24362=VERTEX_POINT('',#83449);
#24363=VERTEX_POINT('',#83453);
#24364=VERTEX_POINT('',#83464);
#24365=VERTEX_POINT('',#83468);
#24366=VERTEX_POINT('',#83479);
#24367=VERTEX_POINT('',#83483);
#24368=VERTEX_POINT('',#83494);
#24369=VERTEX_POINT('',#83498);
#24370=VERTEX_POINT('',#83509);
#24371=VERTEX_POINT('',#83513);
#24372=VERTEX_POINT('',#83524);
#24373=VERTEX_POINT('',#83528);
#24374=VERTEX_POINT('',#83534);
#24375=VERTEX_POINT('',#83536);
#24376=VERTEX_POINT('',#83540);
#24377=VERTEX_POINT('',#83542);
#24378=VERTEX_POINT('',#83546);
#24379=VERTEX_POINT('',#83548);
#24380=VERTEX_POINT('',#83565);
#24381=VERTEX_POINT('',#83566);
#24382=VERTEX_POINT('',#83568);
#24383=VERTEX_POINT('',#83570);
#24384=VERTEX_POINT('',#83579);
#24385=VERTEX_POINT('',#83583);
#24386=VERTEX_POINT('',#83594);
#24387=VERTEX_POINT('',#83598);
#24388=VERTEX_POINT('',#83609);
#24389=VERTEX_POINT('',#83613);
#24390=VERTEX_POINT('',#83624);
#24391=VERTEX_POINT('',#83628);
#24392=VERTEX_POINT('',#83634);
#24393=VERTEX_POINT('',#83636);
#24394=VERTEX_POINT('',#83640);
#24395=VERTEX_POINT('',#83642);
#24396=VERTEX_POINT('',#83646);
#24397=VERTEX_POINT('',#83648);
#24398=VERTEX_POINT('',#83657);
#24399=VERTEX_POINT('',#83661);
#24400=VERTEX_POINT('',#83672);
#24401=VERTEX_POINT('',#83676);
#24402=VERTEX_POINT('',#83687);
#24403=VERTEX_POINT('',#83691);
#24404=VERTEX_POINT('',#83702);
#24405=VERTEX_POINT('',#83706);
#24406=VERTEX_POINT('',#83717);
#24407=VERTEX_POINT('',#83721);
#24408=VERTEX_POINT('',#83732);
#24409=VERTEX_POINT('',#83736);
#24410=VERTEX_POINT('',#83747);
#24411=VERTEX_POINT('',#83751);
#24412=VERTEX_POINT('',#83757);
#24413=VERTEX_POINT('',#83759);
#24414=VERTEX_POINT('',#83763);
#24415=VERTEX_POINT('',#83765);
#24416=VERTEX_POINT('',#83769);
#24417=VERTEX_POINT('',#83771);
#24418=VERTEX_POINT('',#83779);
#24419=VERTEX_POINT('',#83780);
#24420=VERTEX_POINT('',#83782);
#24421=VERTEX_POINT('',#83784);
#24422=VERTEX_POINT('',#83788);
#24423=VERTEX_POINT('',#83790);
#24424=VERTEX_POINT('',#83794);
#24425=VERTEX_POINT('',#83796);
#24426=VERTEX_POINT('',#83804);
#24427=VERTEX_POINT('',#83806);
#24428=VERTEX_POINT('',#83810);
#24429=VERTEX_POINT('',#83814);
#24430=VERTEX_POINT('',#83815);
#24431=VERTEX_POINT('',#83817);
#24432=VERTEX_POINT('',#83819);
#24433=VERTEX_POINT('',#83821);
#24434=VERTEX_POINT('',#83823);
#24435=VERTEX_POINT('',#83825);
#24436=VERTEX_POINT('',#83827);
#24437=VERTEX_POINT('',#83830);
#24438=VERTEX_POINT('',#83832);
#24439=VERTEX_POINT('',#83834);
#24440=VERTEX_POINT('',#83836);
#24441=VERTEX_POINT('',#83838);
#24442=VERTEX_POINT('',#83840);
#24443=VERTEX_POINT('',#83842);
#24444=VERTEX_POINT('',#83844);
#24445=VERTEX_POINT('',#83846);
#24446=VERTEX_POINT('',#83848);
#24447=VERTEX_POINT('',#83851);
#24448=VERTEX_POINT('',#83855);
#24449=VERTEX_POINT('',#83856);
#24450=VERTEX_POINT('',#83858);
#24451=VERTEX_POINT('',#83860);
#24452=VERTEX_POINT('',#83862);
#24453=VERTEX_POINT('',#83864);
#24454=VERTEX_POINT('',#83866);
#24455=VERTEX_POINT('',#83868);
#24456=VERTEX_POINT('',#83871);
#24457=VERTEX_POINT('',#83873);
#24458=VERTEX_POINT('',#83875);
#24459=VERTEX_POINT('',#83878);
#24460=VERTEX_POINT('',#83882);
#24461=VERTEX_POINT('',#83888);
#24462=VERTEX_POINT('',#83892);
#24463=VERTEX_POINT('',#83898);
#24464=VERTEX_POINT('',#83902);
#24465=VERTEX_POINT('',#83908);
#24466=VERTEX_POINT('',#83910);
#24467=VERTEX_POINT('',#83915);
#24468=VERTEX_POINT('',#83917);
#24469=VERTEX_POINT('',#83922);
#24470=VERTEX_POINT('',#83924);
#24471=VERTEX_POINT('',#83927);
#24472=VERTEX_POINT('',#83933);
#24473=VERTEX_POINT('',#83935);
#24474=VERTEX_POINT('',#83938);
#24475=VERTEX_POINT('',#83944);
#24476=VERTEX_POINT('',#83946);
#24477=VERTEX_POINT('',#83949);
#24478=VERTEX_POINT('',#83955);
#24479=VERTEX_POINT('',#83957);
#24480=VERTEX_POINT('',#83960);
#24481=VERTEX_POINT('',#83966);
#24482=VERTEX_POINT('',#83971);
#24483=VERTEX_POINT('',#83973);
#24484=VERTEX_POINT('',#83977);
#24485=VERTEX_POINT('',#83981);
#24486=VERTEX_POINT('',#83985);
#24487=VERTEX_POINT('',#83989);
#24488=VERTEX_POINT('',#83993);
#24489=VERTEX_POINT('',#83997);
#24490=VERTEX_POINT('',#84003);
#24491=VERTEX_POINT('',#84005);
#24492=VERTEX_POINT('',#84009);
#24493=VERTEX_POINT('',#84013);
#24494=VERTEX_POINT('',#84017);
#24495=VERTEX_POINT('',#84030);
#24496=VERTEX_POINT('',#84034);
#24497=VERTEX_POINT('',#84038);
#30601=EDGE_CURVE('',#23840,#23841,#5357,.T.);
#30602=EDGE_CURVE('',#23840,#23842,#5358,.T.);
#30603=EDGE_CURVE('',#23842,#23843,#5359,.T.);
#30604=EDGE_CURVE('',#23841,#23843,#5360,.T.);
#30605=EDGE_CURVE('',#23844,#23840,#5361,.T.);
#30606=EDGE_CURVE('',#23844,#23845,#5362,.T.);
#30607=EDGE_CURVE('',#23845,#23842,#5363,.T.);
#30608=EDGE_CURVE('',#23846,#23844,#5364,.T.);
#30609=EDGE_CURVE('',#23846,#23847,#5365,.T.);
#30610=EDGE_CURVE('',#23847,#23845,#5366,.T.);
#30611=EDGE_CURVE('',#23848,#23846,#5367,.T.);
#30612=EDGE_CURVE('',#23848,#23849,#5368,.T.);
#30613=EDGE_CURVE('',#23849,#23847,#5369,.T.);
#30614=EDGE_CURVE('',#23850,#23848,#5370,.T.);
#30615=EDGE_CURVE('',#23850,#23851,#5371,.T.);
#30616=EDGE_CURVE('',#23851,#23849,#5372,.T.);
#30617=EDGE_CURVE('',#23852,#23850,#5373,.T.);
#30618=EDGE_CURVE('',#23852,#23853,#5374,.T.);
#30619=EDGE_CURVE('',#23853,#23851,#5375,.T.);
#30620=EDGE_CURVE('',#23854,#23852,#5376,.T.);
#30621=EDGE_CURVE('',#23854,#23855,#5377,.T.);
#30622=EDGE_CURVE('',#23855,#23853,#5378,.T.);
#30623=EDGE_CURVE('',#23856,#23854,#5379,.T.);
#30624=EDGE_CURVE('',#23856,#23857,#5380,.T.);
#30625=EDGE_CURVE('',#23857,#23855,#5381,.T.);
#30626=EDGE_CURVE('',#23858,#23856,#5382,.T.);
#30627=EDGE_CURVE('',#23858,#23859,#5383,.T.);
#30628=EDGE_CURVE('',#23859,#23857,#5384,.T.);
#30629=EDGE_CURVE('',#23860,#23858,#5385,.T.);
#30630=EDGE_CURVE('',#23860,#23861,#5386,.T.);
#30631=EDGE_CURVE('',#23861,#23859,#5387,.T.);
#30632=EDGE_CURVE('',#23862,#23860,#5388,.T.);
#30633=EDGE_CURVE('',#23862,#23863,#5389,.T.);
#30634=EDGE_CURVE('',#23863,#23861,#5390,.T.);
#30635=EDGE_CURVE('',#23841,#23862,#5391,.T.);
#30636=EDGE_CURVE('',#23843,#23863,#5392,.T.);
#30637=EDGE_CURVE('',#23864,#23865,#5393,.T.);
#30638=EDGE_CURVE('',#23864,#23866,#5394,.T.);
#30639=EDGE_CURVE('',#23866,#23867,#5395,.T.);
#30640=EDGE_CURVE('',#23865,#23867,#5396,.T.);
#30641=EDGE_CURVE('',#23868,#23864,#5397,.T.);
#30642=EDGE_CURVE('',#23868,#23869,#5398,.T.);
#30643=EDGE_CURVE('',#23869,#23866,#5399,.T.);
#30644=EDGE_CURVE('',#23870,#23868,#5400,.T.);
#30645=EDGE_CURVE('',#23870,#23871,#5401,.T.);
#30646=EDGE_CURVE('',#23871,#23869,#5402,.T.);
#30647=EDGE_CURVE('',#23865,#23870,#5403,.T.);
#30648=EDGE_CURVE('',#23867,#23871,#5404,.T.);
#30649=EDGE_CURVE('',#23872,#23873,#147,.T.);
#30650=EDGE_CURVE('',#23872,#23874,#5405,.T.);
#30651=EDGE_CURVE('',#23874,#23875,#148,.T.);
#30652=EDGE_CURVE('',#23873,#23875,#5406,.T.);
#30653=EDGE_CURVE('',#23876,#23872,#149,.T.);
#30654=EDGE_CURVE('',#23876,#23877,#5407,.T.);
#30655=EDGE_CURVE('',#23877,#23874,#150,.T.);
#30656=EDGE_CURVE('',#23878,#23876,#151,.T.);
#30657=EDGE_CURVE('',#23878,#23879,#5408,.T.);
#30658=EDGE_CURVE('',#23879,#23877,#152,.T.);
#30659=EDGE_CURVE('',#23880,#23878,#153,.T.);
#30660=EDGE_CURVE('',#23880,#23881,#5409,.T.);
#30661=EDGE_CURVE('',#23881,#23879,#154,.T.);
#30662=EDGE_CURVE('',#23882,#23880,#155,.T.);
#30663=EDGE_CURVE('',#23882,#23883,#5410,.T.);
#30664=EDGE_CURVE('',#23883,#23881,#156,.T.);
#30665=EDGE_CURVE('',#23884,#23882,#157,.T.);
#30666=EDGE_CURVE('',#23884,#23885,#5411,.T.);
#30667=EDGE_CURVE('',#23885,#23883,#158,.T.);
#30668=EDGE_CURVE('',#23886,#23884,#159,.T.);
#30669=EDGE_CURVE('',#23886,#23887,#5412,.T.);
#30670=EDGE_CURVE('',#23887,#23885,#160,.T.);
#30671=EDGE_CURVE('',#23888,#23886,#161,.T.);
#30672=EDGE_CURVE('',#23888,#23889,#5413,.T.);
#30673=EDGE_CURVE('',#23889,#23887,#162,.T.);
#30674=EDGE_CURVE('',#23890,#23888,#163,.T.);
#30675=EDGE_CURVE('',#23890,#23891,#5414,.T.);
#30676=EDGE_CURVE('',#23891,#23889,#164,.T.);
#30677=EDGE_CURVE('',#23892,#23890,#165,.T.);
#30678=EDGE_CURVE('',#23892,#23893,#5415,.T.);
#30679=EDGE_CURVE('',#23893,#23891,#166,.T.);
#30680=EDGE_CURVE('',#23894,#23892,#167,.T.);
#30681=EDGE_CURVE('',#23894,#23895,#5416,.T.);
#30682=EDGE_CURVE('',#23895,#23893,#168,.T.);
#30683=EDGE_CURVE('',#23896,#23894,#169,.T.);
#30684=EDGE_CURVE('',#23896,#23897,#5417,.T.);
#30685=EDGE_CURVE('',#23897,#23895,#170,.T.);
#30686=EDGE_CURVE('',#23898,#23896,#171,.T.);
#30687=EDGE_CURVE('',#23898,#23899,#5418,.T.);
#30688=EDGE_CURVE('',#23899,#23897,#172,.T.);
#30689=EDGE_CURVE('',#23900,#23898,#5419,.T.);
#30690=EDGE_CURVE('',#23900,#23901,#5420,.T.);
#30691=EDGE_CURVE('',#23901,#23899,#5421,.T.);
#30692=EDGE_CURVE('',#23902,#23900,#173,.T.);
#30693=EDGE_CURVE('',#23902,#23903,#5422,.T.);
#30694=EDGE_CURVE('',#23903,#23901,#174,.T.);
#30695=EDGE_CURVE('',#23904,#23902,#175,.T.);
#30696=EDGE_CURVE('',#23904,#23905,#5423,.T.);
#30697=EDGE_CURVE('',#23905,#23903,#176,.T.);
#30698=EDGE_CURVE('',#23906,#23904,#177,.T.);
#30699=EDGE_CURVE('',#23906,#23907,#5424,.T.);
#30700=EDGE_CURVE('',#23907,#23905,#178,.T.);
#30701=EDGE_CURVE('',#23908,#23906,#179,.T.);
#30702=EDGE_CURVE('',#23908,#23909,#5425,.T.);
#30703=EDGE_CURVE('',#23909,#23907,#180,.T.);
#30704=EDGE_CURVE('',#23910,#23908,#181,.T.);
#30705=EDGE_CURVE('',#23910,#23911,#5426,.T.);
#30706=EDGE_CURVE('',#23911,#23909,#182,.T.);
#30707=EDGE_CURVE('',#23912,#23910,#183,.T.);
#30708=EDGE_CURVE('',#23912,#23913,#5427,.T.);
#30709=EDGE_CURVE('',#23913,#23911,#184,.T.);
#30710=EDGE_CURVE('',#23914,#23912,#185,.T.);
#30711=EDGE_CURVE('',#23914,#23915,#5428,.T.);
#30712=EDGE_CURVE('',#23915,#23913,#186,.T.);
#30713=EDGE_CURVE('',#23916,#23914,#187,.T.);
#30714=EDGE_CURVE('',#23916,#23917,#5429,.T.);
#30715=EDGE_CURVE('',#23917,#23915,#188,.T.);
#30716=EDGE_CURVE('',#23918,#23916,#189,.T.);
#30717=EDGE_CURVE('',#23918,#23919,#5430,.T.);
#30718=EDGE_CURVE('',#23919,#23917,#190,.T.);
#30719=EDGE_CURVE('',#23920,#23918,#191,.T.);
#30720=EDGE_CURVE('',#23920,#23921,#5431,.T.);
#30721=EDGE_CURVE('',#23921,#23919,#192,.T.);
#30722=EDGE_CURVE('',#23922,#23920,#193,.T.);
#30723=EDGE_CURVE('',#23922,#23923,#5432,.T.);
#30724=EDGE_CURVE('',#23923,#23921,#194,.T.);
#30725=EDGE_CURVE('',#23924,#23922,#195,.T.);
#30726=EDGE_CURVE('',#23924,#23925,#5433,.T.);
#30727=EDGE_CURVE('',#23925,#23923,#196,.T.);
#30728=EDGE_CURVE('',#23926,#23924,#197,.T.);
#30729=EDGE_CURVE('',#23926,#23927,#5434,.T.);
#30730=EDGE_CURVE('',#23927,#23925,#198,.T.);
#30731=EDGE_CURVE('',#23928,#23926,#199,.T.);
#30732=EDGE_CURVE('',#23928,#23929,#5435,.T.);
#30733=EDGE_CURVE('',#23929,#23927,#200,.T.);
#30734=EDGE_CURVE('',#23930,#23928,#201,.T.);
#30735=EDGE_CURVE('',#23930,#23931,#5436,.T.);
#30736=EDGE_CURVE('',#23931,#23929,#202,.T.);
#30737=EDGE_CURVE('',#23932,#23930,#203,.T.);
#30738=EDGE_CURVE('',#23932,#23933,#5437,.T.);
#30739=EDGE_CURVE('',#23933,#23931,#204,.T.);
#30740=EDGE_CURVE('',#23934,#23932,#205,.T.);
#30741=EDGE_CURVE('',#23934,#23935,#5438,.T.);
#30742=EDGE_CURVE('',#23935,#23933,#206,.T.);
#30743=EDGE_CURVE('',#23936,#23934,#207,.T.);
#30744=EDGE_CURVE('',#23936,#23937,#5439,.T.);
#30745=EDGE_CURVE('',#23937,#23935,#208,.T.);
#30746=EDGE_CURVE('',#23938,#23936,#5440,.T.);
#30747=EDGE_CURVE('',#23938,#23939,#5441,.T.);
#30748=EDGE_CURVE('',#23939,#23937,#5442,.T.);
#30749=EDGE_CURVE('',#23940,#23938,#209,.T.);
#30750=EDGE_CURVE('',#23940,#23941,#5443,.T.);
#30751=EDGE_CURVE('',#23941,#23939,#210,.T.);
#30752=EDGE_CURVE('',#23873,#23940,#211,.T.);
#30753=EDGE_CURVE('',#23875,#23941,#212,.T.);
#30754=EDGE_CURVE('',#23942,#23943,#213,.T.);
#30755=EDGE_CURVE('',#23942,#23944,#5444,.T.);
#30756=EDGE_CURVE('',#23944,#23945,#214,.T.);
#30757=EDGE_CURVE('',#23943,#23945,#5445,.T.);
#30758=EDGE_CURVE('',#23946,#23942,#215,.T.);
#30759=EDGE_CURVE('',#23946,#23947,#5446,.T.);
#30760=EDGE_CURVE('',#23947,#23944,#216,.T.);
#30761=EDGE_CURVE('',#23948,#23946,#217,.T.);
#30762=EDGE_CURVE('',#23948,#23949,#5447,.T.);
#30763=EDGE_CURVE('',#23949,#23947,#218,.T.);
#30764=EDGE_CURVE('',#23950,#23948,#219,.T.);
#30765=EDGE_CURVE('',#23950,#23951,#5448,.T.);
#30766=EDGE_CURVE('',#23951,#23949,#220,.T.);
#30767=EDGE_CURVE('',#23952,#23950,#221,.T.);
#30768=EDGE_CURVE('',#23952,#23953,#5449,.T.);
#30769=EDGE_CURVE('',#23953,#23951,#222,.T.);
#30770=EDGE_CURVE('',#23954,#23952,#223,.T.);
#30771=EDGE_CURVE('',#23954,#23955,#5450,.T.);
#30772=EDGE_CURVE('',#23955,#23953,#224,.T.);
#30773=EDGE_CURVE('',#23956,#23954,#225,.T.);
#30774=EDGE_CURVE('',#23956,#23957,#5451,.T.);
#30775=EDGE_CURVE('',#23957,#23955,#226,.T.);
#30776=EDGE_CURVE('',#23958,#23956,#227,.T.);
#30777=EDGE_CURVE('',#23958,#23959,#5452,.T.);
#30778=EDGE_CURVE('',#23959,#23957,#228,.T.);
#30779=EDGE_CURVE('',#23960,#23958,#5453,.T.);
#30780=EDGE_CURVE('',#23960,#23961,#5454,.T.);
#30781=EDGE_CURVE('',#23961,#23959,#5455,.T.);
#30782=EDGE_CURVE('',#23962,#23960,#229,.T.);
#30783=EDGE_CURVE('',#23962,#23963,#5456,.T.);
#30784=EDGE_CURVE('',#23963,#23961,#230,.T.);
#30785=EDGE_CURVE('',#23964,#23962,#231,.T.);
#30786=EDGE_CURVE('',#23964,#23965,#5457,.T.);
#30787=EDGE_CURVE('',#23965,#23963,#232,.T.);
#30788=EDGE_CURVE('',#23966,#23964,#233,.T.);
#30789=EDGE_CURVE('',#23966,#23967,#5458,.T.);
#30790=EDGE_CURVE('',#23967,#23965,#234,.T.);
#30791=EDGE_CURVE('',#23968,#23966,#235,.T.);
#30792=EDGE_CURVE('',#23968,#23969,#5459,.T.);
#30793=EDGE_CURVE('',#23969,#23967,#236,.T.);
#30794=EDGE_CURVE('',#23970,#23968,#237,.T.);
#30795=EDGE_CURVE('',#23970,#23971,#5460,.T.);
#30796=EDGE_CURVE('',#23971,#23969,#238,.T.);
#30797=EDGE_CURVE('',#23972,#23970,#239,.T.);
#30798=EDGE_CURVE('',#23972,#23973,#5461,.T.);
#30799=EDGE_CURVE('',#23973,#23971,#240,.T.);
#30800=EDGE_CURVE('',#23974,#23972,#241,.T.);
#30801=EDGE_CURVE('',#23974,#23975,#5462,.T.);
#30802=EDGE_CURVE('',#23975,#23973,#242,.T.);
#30803=EDGE_CURVE('',#23976,#23974,#243,.T.);
#30804=EDGE_CURVE('',#23976,#23977,#5463,.T.);
#30805=EDGE_CURVE('',#23977,#23975,#244,.T.);
#30806=EDGE_CURVE('',#23978,#23976,#245,.T.);
#30807=EDGE_CURVE('',#23978,#23979,#5464,.T.);
#30808=EDGE_CURVE('',#23979,#23977,#246,.T.);
#30809=EDGE_CURVE('',#23980,#23978,#247,.T.);
#30810=EDGE_CURVE('',#23980,#23981,#5465,.T.);
#30811=EDGE_CURVE('',#23981,#23979,#248,.T.);
#30812=EDGE_CURVE('',#23982,#23980,#5466,.T.);
#30813=EDGE_CURVE('',#23982,#23983,#5467,.T.);
#30814=EDGE_CURVE('',#23983,#23981,#5468,.T.);
#30815=EDGE_CURVE('',#23984,#23982,#249,.T.);
#30816=EDGE_CURVE('',#23984,#23985,#5469,.T.);
#30817=EDGE_CURVE('',#23985,#23983,#250,.T.);
#30818=EDGE_CURVE('',#23943,#23984,#251,.T.);
#30819=EDGE_CURVE('',#23945,#23985,#252,.T.);
#30820=EDGE_CURVE('',#23986,#23987,#5470,.T.);
#30821=EDGE_CURVE('',#23986,#23988,#5471,.T.);
#30822=EDGE_CURVE('',#23988,#23989,#5472,.T.);
#30823=EDGE_CURVE('',#23987,#23989,#5473,.T.);
#30824=EDGE_CURVE('',#23990,#23986,#5474,.T.);
#30825=EDGE_CURVE('',#23990,#23991,#5475,.T.);
#30826=EDGE_CURVE('',#23991,#23988,#5476,.T.);
#30827=EDGE_CURVE('',#23992,#23990,#5477,.T.);
#30828=EDGE_CURVE('',#23992,#23993,#5478,.T.);
#30829=EDGE_CURVE('',#23993,#23991,#5479,.T.);
#30830=EDGE_CURVE('',#23994,#23992,#5480,.T.);
#30831=EDGE_CURVE('',#23994,#23995,#5481,.T.);
#30832=EDGE_CURVE('',#23995,#23993,#5482,.T.);
#30833=EDGE_CURVE('',#23996,#23994,#5483,.T.);
#30834=EDGE_CURVE('',#23996,#23997,#5484,.T.);
#30835=EDGE_CURVE('',#23997,#23995,#5485,.T.);
#30836=EDGE_CURVE('',#23987,#23996,#5486,.T.);
#30837=EDGE_CURVE('',#23989,#23997,#5487,.T.);
#30838=EDGE_CURVE('',#23998,#23999,#5488,.T.);
#30839=EDGE_CURVE('',#23998,#24000,#5489,.T.);
#30840=EDGE_CURVE('',#24000,#24001,#5490,.T.);
#30841=EDGE_CURVE('',#23999,#24001,#5491,.T.);
#30842=EDGE_CURVE('',#24002,#23998,#5492,.T.);
#30843=EDGE_CURVE('',#24002,#24003,#5493,.T.);
#30844=EDGE_CURVE('',#24003,#24000,#5494,.T.);
#30845=EDGE_CURVE('',#24004,#24002,#5495,.T.);
#30846=EDGE_CURVE('',#24004,#24005,#5496,.T.);
#30847=EDGE_CURVE('',#24005,#24003,#5497,.T.);
#30848=EDGE_CURVE('',#24006,#24004,#5498,.T.);
#30849=EDGE_CURVE('',#24006,#24007,#5499,.T.);
#30850=EDGE_CURVE('',#24007,#24005,#5500,.T.);
#30851=EDGE_CURVE('',#24008,#24006,#5501,.T.);
#30852=EDGE_CURVE('',#24008,#24009,#5502,.T.);
#30853=EDGE_CURVE('',#24009,#24007,#5503,.T.);
#30854=EDGE_CURVE('',#24010,#24008,#5504,.T.);
#30855=EDGE_CURVE('',#24010,#24011,#5505,.T.);
#30856=EDGE_CURVE('',#24011,#24009,#5506,.T.);
#30857=EDGE_CURVE('',#24012,#24010,#5507,.T.);
#30858=EDGE_CURVE('',#24012,#24013,#5508,.T.);
#30859=EDGE_CURVE('',#24013,#24011,#5509,.T.);
#30860=EDGE_CURVE('',#23999,#24012,#5510,.T.);
#30861=EDGE_CURVE('',#24001,#24013,#5511,.T.);
#30862=EDGE_CURVE('',#24014,#24015,#253,.T.);
#30863=EDGE_CURVE('',#24014,#24016,#5512,.T.);
#30864=EDGE_CURVE('',#24016,#24017,#254,.T.);
#30865=EDGE_CURVE('',#24015,#24017,#5513,.T.);
#30866=EDGE_CURVE('',#24018,#24014,#255,.T.);
#30867=EDGE_CURVE('',#24018,#24019,#5514,.T.);
#30868=EDGE_CURVE('',#24019,#24016,#256,.T.);
#30869=EDGE_CURVE('',#24020,#24018,#257,.T.);
#30870=EDGE_CURVE('',#24020,#24021,#5515,.T.);
#30871=EDGE_CURVE('',#24021,#24019,#258,.T.);
#30872=EDGE_CURVE('',#24022,#24020,#259,.T.);
#30873=EDGE_CURVE('',#24022,#24023,#5516,.T.);
#30874=EDGE_CURVE('',#24023,#24021,#260,.T.);
#30875=EDGE_CURVE('',#24024,#24022,#5517,.T.);
#30876=EDGE_CURVE('',#24024,#24025,#5518,.T.);
#30877=EDGE_CURVE('',#24025,#24023,#5519,.T.);
#30878=EDGE_CURVE('',#24026,#24024,#5520,.T.);
#30879=EDGE_CURVE('',#24026,#24027,#5521,.T.);
#30880=EDGE_CURVE('',#24027,#24025,#5522,.T.);
#30881=EDGE_CURVE('',#24028,#24026,#5523,.T.);
#30882=EDGE_CURVE('',#24028,#24029,#5524,.T.);
#30883=EDGE_CURVE('',#24029,#24027,#5525,.T.);
#30884=EDGE_CURVE('',#24030,#24028,#261,.T.);
#30885=EDGE_CURVE('',#24030,#24031,#5526,.T.);
#30886=EDGE_CURVE('',#24031,#24029,#262,.T.);
#30887=EDGE_CURVE('',#24032,#24030,#263,.T.);
#30888=EDGE_CURVE('',#24032,#24033,#5527,.T.);
#30889=EDGE_CURVE('',#24033,#24031,#264,.T.);
#30890=EDGE_CURVE('',#24034,#24032,#265,.T.);
#30891=EDGE_CURVE('',#24034,#24035,#5528,.T.);
#30892=EDGE_CURVE('',#24035,#24033,#266,.T.);
#30893=EDGE_CURVE('',#24036,#24034,#267,.T.);
#30894=EDGE_CURVE('',#24036,#24037,#5529,.T.);
#30895=EDGE_CURVE('',#24037,#24035,#268,.T.);
#30896=EDGE_CURVE('',#24038,#24036,#269,.T.);
#30897=EDGE_CURVE('',#24038,#24039,#5530,.T.);
#30898=EDGE_CURVE('',#24039,#24037,#270,.T.);
#30899=EDGE_CURVE('',#24040,#24038,#271,.T.);
#30900=EDGE_CURVE('',#24040,#24041,#5531,.T.);
#30901=EDGE_CURVE('',#24041,#24039,#272,.T.);
#30902=EDGE_CURVE('',#24042,#24040,#5532,.T.);
#30903=EDGE_CURVE('',#24042,#24043,#5533,.T.);
#30904=EDGE_CURVE('',#24043,#24041,#5534,.T.);
#30905=EDGE_CURVE('',#24044,#24042,#5535,.T.);
#30906=EDGE_CURVE('',#24044,#24045,#5536,.T.);
#30907=EDGE_CURVE('',#24045,#24043,#5537,.T.);
#30908=EDGE_CURVE('',#24046,#24044,#5538,.T.);
#30909=EDGE_CURVE('',#24046,#24047,#5539,.T.);
#30910=EDGE_CURVE('',#24047,#24045,#5540,.T.);
#30911=EDGE_CURVE('',#24015,#24046,#273,.T.);
#30912=EDGE_CURVE('',#24017,#24047,#274,.T.);
#30913=EDGE_CURVE('',#24048,#24049,#5541,.T.);
#30914=EDGE_CURVE('',#24048,#24050,#5542,.T.);
#30915=EDGE_CURVE('',#24050,#24051,#5543,.T.);
#30916=EDGE_CURVE('',#24049,#24051,#5544,.T.);
#30917=EDGE_CURVE('',#24052,#24048,#275,.T.);
#30918=EDGE_CURVE('',#24052,#24053,#5545,.T.);
#30919=EDGE_CURVE('',#24053,#24050,#276,.T.);
#30920=EDGE_CURVE('',#24054,#24052,#277,.T.);
#30921=EDGE_CURVE('',#24054,#24055,#5546,.T.);
#30922=EDGE_CURVE('',#24055,#24053,#278,.T.);
#30923=EDGE_CURVE('',#24056,#24054,#279,.T.);
#30924=EDGE_CURVE('',#24056,#24057,#5547,.T.);
#30925=EDGE_CURVE('',#24057,#24055,#280,.T.);
#30926=EDGE_CURVE('',#24058,#24056,#281,.T.);
#30927=EDGE_CURVE('',#24058,#24059,#5548,.T.);
#30928=EDGE_CURVE('',#24059,#24057,#282,.T.);
#30929=EDGE_CURVE('',#24060,#24058,#5549,.T.);
#30930=EDGE_CURVE('',#24060,#24061,#5550,.T.);
#30931=EDGE_CURVE('',#24061,#24059,#5551,.T.);
#30932=EDGE_CURVE('',#24062,#24060,#5552,.T.);
#30933=EDGE_CURVE('',#24062,#24063,#5553,.T.);
#30934=EDGE_CURVE('',#24063,#24061,#5554,.T.);
#30935=EDGE_CURVE('',#24064,#24062,#5555,.T.);
#30936=EDGE_CURVE('',#24064,#24065,#5556,.T.);
#30937=EDGE_CURVE('',#24065,#24063,#5557,.T.);
#30938=EDGE_CURVE('',#24066,#24064,#283,.T.);
#30939=EDGE_CURVE('',#24066,#24067,#5558,.T.);
#30940=EDGE_CURVE('',#24067,#24065,#284,.T.);
#30941=EDGE_CURVE('',#24068,#24066,#285,.T.);
#30942=EDGE_CURVE('',#24068,#24069,#5559,.T.);
#30943=EDGE_CURVE('',#24069,#24067,#286,.T.);
#30944=EDGE_CURVE('',#24070,#24068,#287,.T.);
#30945=EDGE_CURVE('',#24070,#24071,#5560,.T.);
#30946=EDGE_CURVE('',#24071,#24069,#288,.T.);
#30947=EDGE_CURVE('',#24072,#24070,#289,.T.);
#30948=EDGE_CURVE('',#24072,#24073,#5561,.T.);
#30949=EDGE_CURVE('',#24073,#24071,#290,.T.);
#30950=EDGE_CURVE('',#24074,#24072,#291,.T.);
#30951=EDGE_CURVE('',#24074,#24075,#5562,.T.);
#30952=EDGE_CURVE('',#24075,#24073,#292,.T.);
#30953=EDGE_CURVE('',#24076,#24074,#293,.T.);
#30954=EDGE_CURVE('',#24076,#24077,#5563,.T.);
#30955=EDGE_CURVE('',#24077,#24075,#294,.T.);
#30956=EDGE_CURVE('',#24078,#24076,#295,.T.);
#30957=EDGE_CURVE('',#24078,#24079,#5564,.T.);
#30958=EDGE_CURVE('',#24079,#24077,#296,.T.);
#30959=EDGE_CURVE('',#24080,#24078,#5565,.T.);
#30960=EDGE_CURVE('',#24080,#24081,#5566,.T.);
#30961=EDGE_CURVE('',#24081,#24079,#5567,.T.);
#30962=EDGE_CURVE('',#24082,#24080,#5568,.T.);
#30963=EDGE_CURVE('',#24082,#24083,#5569,.T.);
#30964=EDGE_CURVE('',#24083,#24081,#5570,.T.);
#30965=EDGE_CURVE('',#24084,#24082,#5571,.T.);
#30966=EDGE_CURVE('',#24084,#24085,#5572,.T.);
#30967=EDGE_CURVE('',#24085,#24083,#5573,.T.);
#30968=EDGE_CURVE('',#24049,#24084,#5574,.T.);
#30969=EDGE_CURVE('',#24051,#24085,#5575,.T.);
#30970=EDGE_CURVE('',#24086,#24087,#5576,.T.);
#30971=EDGE_CURVE('',#24086,#24088,#5577,.T.);
#30972=EDGE_CURVE('',#24088,#24089,#5578,.T.);
#30973=EDGE_CURVE('',#24087,#24089,#5579,.T.);
#30974=EDGE_CURVE('',#24090,#24086,#5580,.T.);
#30975=EDGE_CURVE('',#24090,#24091,#5581,.T.);
#30976=EDGE_CURVE('',#24091,#24088,#5582,.T.);
#30977=EDGE_CURVE('',#24092,#24090,#5583,.T.);
#30978=EDGE_CURVE('',#24092,#24093,#5584,.T.);
#30979=EDGE_CURVE('',#24093,#24091,#5585,.T.);
#30980=EDGE_CURVE('',#24094,#24092,#5586,.T.);
#30981=EDGE_CURVE('',#24094,#24095,#5587,.T.);
#30982=EDGE_CURVE('',#24095,#24093,#5588,.T.);
#30983=EDGE_CURVE('',#24096,#24094,#5589,.T.);
#30984=EDGE_CURVE('',#24096,#24097,#5590,.T.);
#30985=EDGE_CURVE('',#24097,#24095,#5591,.T.);
#30986=EDGE_CURVE('',#24098,#24096,#5592,.T.);
#30987=EDGE_CURVE('',#24098,#24099,#5593,.T.);
#30988=EDGE_CURVE('',#24099,#24097,#5594,.T.);
#30989=EDGE_CURVE('',#24100,#24098,#5595,.T.);
#30990=EDGE_CURVE('',#24100,#24101,#5596,.T.);
#30991=EDGE_CURVE('',#24101,#24099,#5597,.T.);
#30992=EDGE_CURVE('',#24087,#24100,#5598,.T.);
#30993=EDGE_CURVE('',#24089,#24101,#5599,.T.);
#30994=EDGE_CURVE('',#24102,#24103,#297,.T.);
#30995=EDGE_CURVE('',#24102,#24104,#5600,.T.);
#30996=EDGE_CURVE('',#24104,#24105,#298,.T.);
#30997=EDGE_CURVE('',#24103,#24105,#5601,.T.);
#30998=EDGE_CURVE('',#24106,#24102,#299,.T.);
#30999=EDGE_CURVE('',#24106,#24107,#5602,.T.);
#31000=EDGE_CURVE('',#24107,#24104,#300,.T.);
#31001=EDGE_CURVE('',#24108,#24106,#5603,.T.);
#31002=EDGE_CURVE('',#24108,#24109,#5604,.T.);
#31003=EDGE_CURVE('',#24109,#24107,#5605,.T.);
#31004=EDGE_CURVE('',#24110,#24108,#301,.T.);
#31005=EDGE_CURVE('',#24110,#24111,#5606,.T.);
#31006=EDGE_CURVE('',#24111,#24109,#302,.T.);
#31007=EDGE_CURVE('',#24112,#24110,#303,.T.);
#31008=EDGE_CURVE('',#24112,#24113,#5607,.T.);
#31009=EDGE_CURVE('',#24113,#24111,#304,.T.);
#31010=EDGE_CURVE('',#24114,#24112,#5608,.T.);
#31011=EDGE_CURVE('',#24114,#24115,#5609,.T.);
#31012=EDGE_CURVE('',#24115,#24113,#5610,.T.);
#31013=EDGE_CURVE('',#24116,#24114,#5611,.T.);
#31014=EDGE_CURVE('',#24116,#24117,#5612,.T.);
#31015=EDGE_CURVE('',#24117,#24115,#5613,.T.);
#31016=EDGE_CURVE('',#24118,#24116,#5614,.T.);
#31017=EDGE_CURVE('',#24118,#24119,#5615,.T.);
#31018=EDGE_CURVE('',#24119,#24117,#5616,.T.);
#31019=EDGE_CURVE('',#24103,#24118,#5617,.T.);
#31020=EDGE_CURVE('',#24105,#24119,#5618,.T.);
#31021=EDGE_CURVE('',#24120,#24121,#305,.T.);
#31022=EDGE_CURVE('',#24120,#24122,#5619,.T.);
#31023=EDGE_CURVE('',#24122,#24123,#306,.T.);
#31024=EDGE_CURVE('',#24121,#24123,#5620,.T.);
#31025=EDGE_CURVE('',#24124,#24120,#307,.T.);
#31026=EDGE_CURVE('',#24124,#24125,#5621,.T.);
#31027=EDGE_CURVE('',#24125,#24122,#308,.T.);
#31028=EDGE_CURVE('',#24126,#24124,#309,.T.);
#31029=EDGE_CURVE('',#24126,#24127,#5622,.T.);
#31030=EDGE_CURVE('',#24127,#24125,#310,.T.);
#31031=EDGE_CURVE('',#24128,#24126,#311,.T.);
#31032=EDGE_CURVE('',#24128,#24129,#5623,.T.);
#31033=EDGE_CURVE('',#24129,#24127,#312,.T.);
#31034=EDGE_CURVE('',#24130,#24128,#313,.T.);
#31035=EDGE_CURVE('',#24130,#24131,#5624,.T.);
#31036=EDGE_CURVE('',#24131,#24129,#314,.T.);
#31037=EDGE_CURVE('',#24132,#24130,#315,.T.);
#31038=EDGE_CURVE('',#24132,#24133,#5625,.T.);
#31039=EDGE_CURVE('',#24133,#24131,#316,.T.);
#31040=EDGE_CURVE('',#24134,#24132,#317,.T.);
#31041=EDGE_CURVE('',#24134,#24135,#5626,.T.);
#31042=EDGE_CURVE('',#24135,#24133,#318,.T.);
#31043=EDGE_CURVE('',#24136,#24134,#319,.T.);
#31044=EDGE_CURVE('',#24136,#24137,#5627,.T.);
#31045=EDGE_CURVE('',#24137,#24135,#320,.T.);
#31046=EDGE_CURVE('',#24138,#24136,#321,.T.);
#31047=EDGE_CURVE('',#24138,#24139,#5628,.T.);
#31048=EDGE_CURVE('',#24139,#24137,#322,.T.);
#31049=EDGE_CURVE('',#24140,#24138,#323,.T.);
#31050=EDGE_CURVE('',#24140,#24141,#5629,.T.);
#31051=EDGE_CURVE('',#24141,#24139,#324,.T.);
#31052=EDGE_CURVE('',#24142,#24140,#325,.T.);
#31053=EDGE_CURVE('',#24142,#24143,#5630,.T.);
#31054=EDGE_CURVE('',#24143,#24141,#326,.T.);
#31055=EDGE_CURVE('',#24121,#24142,#327,.T.);
#31056=EDGE_CURVE('',#24123,#24143,#328,.T.);
#31057=EDGE_CURVE('',#24144,#24145,#329,.T.);
#31058=EDGE_CURVE('',#24144,#24146,#5631,.T.);
#31059=EDGE_CURVE('',#24146,#24147,#330,.T.);
#31060=EDGE_CURVE('',#24145,#24147,#5632,.T.);
#31061=EDGE_CURVE('',#24148,#24144,#331,.T.);
#31062=EDGE_CURVE('',#24148,#24149,#5633,.T.);
#31063=EDGE_CURVE('',#24149,#24146,#332,.T.);
#31064=EDGE_CURVE('',#24150,#24148,#5634,.T.);
#31065=EDGE_CURVE('',#24150,#24151,#5635,.T.);
#31066=EDGE_CURVE('',#24151,#24149,#5636,.T.);
#31067=EDGE_CURVE('',#24152,#24150,#333,.T.);
#31068=EDGE_CURVE('',#24152,#24153,#5637,.T.);
#31069=EDGE_CURVE('',#24153,#24151,#334,.T.);
#31070=EDGE_CURVE('',#24154,#24152,#335,.T.);
#31071=EDGE_CURVE('',#24154,#24155,#5638,.T.);
#31072=EDGE_CURVE('',#24155,#24153,#336,.T.);
#31073=EDGE_CURVE('',#24156,#24154,#5639,.T.);
#31074=EDGE_CURVE('',#24156,#24157,#5640,.T.);
#31075=EDGE_CURVE('',#24157,#24155,#5641,.T.);
#31076=EDGE_CURVE('',#24158,#24156,#5642,.T.);
#31077=EDGE_CURVE('',#24158,#24159,#5643,.T.);
#31078=EDGE_CURVE('',#24159,#24157,#5644,.T.);
#31079=EDGE_CURVE('',#24160,#24158,#5645,.T.);
#31080=EDGE_CURVE('',#24160,#24161,#5646,.T.);
#31081=EDGE_CURVE('',#24161,#24159,#5647,.T.);
#31082=EDGE_CURVE('',#24145,#24160,#5648,.T.);
#31083=EDGE_CURVE('',#24147,#24161,#5649,.T.);
#31084=EDGE_CURVE('',#24162,#24163,#5650,.T.);
#31085=EDGE_CURVE('',#24162,#24164,#5651,.T.);
#31086=EDGE_CURVE('',#24164,#24165,#5652,.T.);
#31087=EDGE_CURVE('',#24163,#24165,#5653,.T.);
#31088=EDGE_CURVE('',#24166,#24162,#5654,.T.);
#31089=EDGE_CURVE('',#24166,#24167,#5655,.T.);
#31090=EDGE_CURVE('',#24167,#24164,#5656,.T.);
#31091=EDGE_CURVE('',#24168,#24166,#5657,.T.);
#31092=EDGE_CURVE('',#24168,#24169,#5658,.T.);
#31093=EDGE_CURVE('',#24169,#24167,#5659,.T.);
#31094=EDGE_CURVE('',#24163,#24168,#5660,.T.);
#31095=EDGE_CURVE('',#24165,#24169,#5661,.T.);
#31096=EDGE_CURVE('',#24170,#24171,#337,.T.);
#31097=EDGE_CURVE('',#24170,#24172,#5662,.T.);
#31098=EDGE_CURVE('',#24172,#24173,#338,.T.);
#31099=EDGE_CURVE('',#24171,#24173,#5663,.T.);
#31100=EDGE_CURVE('',#24174,#24170,#339,.T.);
#31101=EDGE_CURVE('',#24174,#24175,#5664,.T.);
#31102=EDGE_CURVE('',#24175,#24172,#340,.T.);
#31103=EDGE_CURVE('',#24176,#24174,#341,.T.);
#31104=EDGE_CURVE('',#24176,#24177,#5665,.T.);
#31105=EDGE_CURVE('',#24177,#24175,#342,.T.);
#31106=EDGE_CURVE('',#24178,#24176,#343,.T.);
#31107=EDGE_CURVE('',#24178,#24179,#5666,.T.);
#31108=EDGE_CURVE('',#24179,#24177,#344,.T.);
#31109=EDGE_CURVE('',#24180,#24178,#345,.T.);
#31110=EDGE_CURVE('',#24180,#24181,#5667,.T.);
#31111=EDGE_CURVE('',#24181,#24179,#346,.T.);
#31112=EDGE_CURVE('',#24182,#24180,#5668,.T.);
#31113=EDGE_CURVE('',#24182,#24183,#5669,.T.);
#31114=EDGE_CURVE('',#24183,#24181,#5670,.T.);
#31115=EDGE_CURVE('',#24184,#24182,#5671,.T.);
#31116=EDGE_CURVE('',#24184,#24185,#5672,.T.);
#31117=EDGE_CURVE('',#24185,#24183,#5673,.T.);
#31118=EDGE_CURVE('',#24186,#24184,#5674,.T.);
#31119=EDGE_CURVE('',#24186,#24187,#5675,.T.);
#31120=EDGE_CURVE('',#24187,#24185,#5676,.T.);
#31121=EDGE_CURVE('',#24188,#24186,#5677,.T.);
#31122=EDGE_CURVE('',#24188,#24189,#5678,.T.);
#31123=EDGE_CURVE('',#24189,#24187,#5679,.T.);
#31124=EDGE_CURVE('',#24190,#24188,#5680,.T.);
#31125=EDGE_CURVE('',#24190,#24191,#5681,.T.);
#31126=EDGE_CURVE('',#24191,#24189,#5682,.T.);
#31127=EDGE_CURVE('',#24192,#24190,#5683,.T.);
#31128=EDGE_CURVE('',#24192,#24193,#5684,.T.);
#31129=EDGE_CURVE('',#24193,#24191,#5685,.T.);
#31130=EDGE_CURVE('',#24194,#24192,#347,.T.);
#31131=EDGE_CURVE('',#24194,#24195,#5686,.T.);
#31132=EDGE_CURVE('',#24195,#24193,#348,.T.);
#31133=EDGE_CURVE('',#24196,#24194,#349,.T.);
#31134=EDGE_CURVE('',#24196,#24197,#5687,.T.);
#31135=EDGE_CURVE('',#24197,#24195,#350,.T.);
#31136=EDGE_CURVE('',#24198,#24196,#351,.T.);
#31137=EDGE_CURVE('',#24198,#24199,#5688,.T.);
#31138=EDGE_CURVE('',#24199,#24197,#352,.T.);
#31139=EDGE_CURVE('',#24200,#24198,#353,.T.);
#31140=EDGE_CURVE('',#24200,#24201,#5689,.T.);
#31141=EDGE_CURVE('',#24201,#24199,#354,.T.);
#31142=EDGE_CURVE('',#24202,#24200,#355,.T.);
#31143=EDGE_CURVE('',#24202,#24203,#5690,.T.);
#31144=EDGE_CURVE('',#24203,#24201,#356,.T.);
#31145=EDGE_CURVE('',#24204,#24202,#357,.T.);
#31146=EDGE_CURVE('',#24204,#24205,#5691,.T.);
#31147=EDGE_CURVE('',#24205,#24203,#358,.T.);
#31148=EDGE_CURVE('',#24206,#24204,#359,.T.);
#31149=EDGE_CURVE('',#24206,#24207,#5692,.T.);
#31150=EDGE_CURVE('',#24207,#24205,#360,.T.);
#31151=EDGE_CURVE('',#24208,#24206,#361,.T.);
#31152=EDGE_CURVE('',#24208,#24209,#5693,.T.);
#31153=EDGE_CURVE('',#24209,#24207,#362,.T.);
#31154=EDGE_CURVE('',#24210,#24208,#5694,.T.);
#31155=EDGE_CURVE('',#24210,#24211,#5695,.T.);
#31156=EDGE_CURVE('',#24211,#24209,#5696,.T.);
#31157=EDGE_CURVE('',#24212,#24210,#363,.T.);
#31158=EDGE_CURVE('',#24212,#24213,#5697,.T.);
#31159=EDGE_CURVE('',#24213,#24211,#364,.T.);
#31160=EDGE_CURVE('',#24171,#24212,#365,.T.);
#31161=EDGE_CURVE('',#24173,#24213,#366,.T.);
#31162=EDGE_CURVE('',#24214,#24215,#367,.T.);
#31163=EDGE_CURVE('',#24214,#24216,#5698,.T.);
#31164=EDGE_CURVE('',#24216,#24217,#368,.T.);
#31165=EDGE_CURVE('',#24215,#24217,#5699,.T.);
#31166=EDGE_CURVE('',#24218,#24214,#369,.T.);
#31167=EDGE_CURVE('',#24218,#24219,#5700,.T.);
#31168=EDGE_CURVE('',#24219,#24216,#370,.T.);
#31169=EDGE_CURVE('',#24220,#24218,#371,.T.);
#31170=EDGE_CURVE('',#24220,#24221,#5701,.T.);
#31171=EDGE_CURVE('',#24221,#24219,#372,.T.);
#31172=EDGE_CURVE('',#24222,#24220,#373,.T.);
#31173=EDGE_CURVE('',#24222,#24223,#5702,.T.);
#31174=EDGE_CURVE('',#24223,#24221,#374,.T.);
#31175=EDGE_CURVE('',#24224,#24222,#375,.T.);
#31176=EDGE_CURVE('',#24224,#24225,#5703,.T.);
#31177=EDGE_CURVE('',#24225,#24223,#376,.T.);
#31178=EDGE_CURVE('',#24226,#24224,#377,.T.);
#31179=EDGE_CURVE('',#24226,#24227,#5704,.T.);
#31180=EDGE_CURVE('',#24227,#24225,#378,.T.);
#31181=EDGE_CURVE('',#24228,#24226,#379,.T.);
#31182=EDGE_CURVE('',#24228,#24229,#5705,.T.);
#31183=EDGE_CURVE('',#24229,#24227,#380,.T.);
#31184=EDGE_CURVE('',#24230,#24228,#381,.T.);
#31185=EDGE_CURVE('',#24230,#24231,#5706,.T.);
#31186=EDGE_CURVE('',#24231,#24229,#382,.T.);
#31187=EDGE_CURVE('',#24232,#24230,#383,.T.);
#31188=EDGE_CURVE('',#24232,#24233,#5707,.T.);
#31189=EDGE_CURVE('',#24233,#24231,#384,.T.);
#31190=EDGE_CURVE('',#24234,#24232,#385,.T.);
#31191=EDGE_CURVE('',#24234,#24235,#5708,.T.);
#31192=EDGE_CURVE('',#24235,#24233,#386,.T.);
#31193=EDGE_CURVE('',#24215,#24234,#387,.T.);
#31194=EDGE_CURVE('',#24217,#24235,#388,.T.);
#31195=EDGE_CURVE('',#24236,#24237,#389,.T.);
#31196=EDGE_CURVE('',#24236,#24238,#5709,.T.);
#31197=EDGE_CURVE('',#24238,#24239,#390,.T.);
#31198=EDGE_CURVE('',#24237,#24239,#5710,.T.);
#31199=EDGE_CURVE('',#24240,#24236,#391,.T.);
#31200=EDGE_CURVE('',#24240,#24241,#5711,.T.);
#31201=EDGE_CURVE('',#24241,#24238,#392,.T.);
#31202=EDGE_CURVE('',#24242,#24240,#393,.T.);
#31203=EDGE_CURVE('',#24242,#24243,#5712,.T.);
#31204=EDGE_CURVE('',#24243,#24241,#394,.T.);
#31205=EDGE_CURVE('',#24244,#24242,#395,.T.);
#31206=EDGE_CURVE('',#24244,#24245,#5713,.T.);
#31207=EDGE_CURVE('',#24245,#24243,#396,.T.);
#31208=EDGE_CURVE('',#24246,#24244,#397,.T.);
#31209=EDGE_CURVE('',#24246,#24247,#5714,.T.);
#31210=EDGE_CURVE('',#24247,#24245,#398,.T.);
#31211=EDGE_CURVE('',#24248,#24246,#399,.T.);
#31212=EDGE_CURVE('',#24248,#24249,#5715,.T.);
#31213=EDGE_CURVE('',#24249,#24247,#400,.T.);
#31214=EDGE_CURVE('',#24250,#24248,#401,.T.);
#31215=EDGE_CURVE('',#24250,#24251,#5716,.T.);
#31216=EDGE_CURVE('',#24251,#24249,#402,.T.);
#31217=EDGE_CURVE('',#24252,#24250,#403,.T.);
#31218=EDGE_CURVE('',#24252,#24253,#5717,.T.);
#31219=EDGE_CURVE('',#24253,#24251,#404,.T.);
#31220=EDGE_CURVE('',#24254,#24252,#405,.T.);
#31221=EDGE_CURVE('',#24254,#24255,#5718,.T.);
#31222=EDGE_CURVE('',#24255,#24253,#406,.T.);
#31223=EDGE_CURVE('',#24256,#24254,#407,.T.);
#31224=EDGE_CURVE('',#24256,#24257,#5719,.T.);
#31225=EDGE_CURVE('',#24257,#24255,#408,.T.);
#31226=EDGE_CURVE('',#24258,#24256,#409,.T.);
#31227=EDGE_CURVE('',#24258,#24259,#5720,.T.);
#31228=EDGE_CURVE('',#24259,#24257,#410,.T.);
#31229=EDGE_CURVE('',#24260,#24258,#5721,.T.);
#31230=EDGE_CURVE('',#24260,#24261,#5722,.T.);
#31231=EDGE_CURVE('',#24261,#24259,#5723,.T.);
#31232=EDGE_CURVE('',#24262,#24260,#411,.T.);
#31233=EDGE_CURVE('',#24262,#24263,#5724,.T.);
#31234=EDGE_CURVE('',#24263,#24261,#412,.T.);
#31235=EDGE_CURVE('',#24264,#24262,#413,.T.);
#31236=EDGE_CURVE('',#24264,#24265,#5725,.T.);
#31237=EDGE_CURVE('',#24265,#24263,#414,.T.);
#31238=EDGE_CURVE('',#24237,#24264,#415,.T.);
#31239=EDGE_CURVE('',#24239,#24265,#416,.T.);
#31240=EDGE_CURVE('',#24266,#24267,#5726,.T.);
#31241=EDGE_CURVE('',#24266,#24268,#5727,.T.);
#31242=EDGE_CURVE('',#24268,#24269,#5728,.T.);
#31243=EDGE_CURVE('',#24267,#24269,#5729,.T.);
#31244=EDGE_CURVE('',#24270,#24266,#5730,.T.);
#31245=EDGE_CURVE('',#24270,#24271,#5731,.T.);
#31246=EDGE_CURVE('',#24271,#24268,#5732,.T.);
#31247=EDGE_CURVE('',#24272,#24270,#5733,.T.);
#31248=EDGE_CURVE('',#24272,#24273,#5734,.T.);
#31249=EDGE_CURVE('',#24273,#24271,#5735,.T.);
#31250=EDGE_CURVE('',#24274,#24272,#5736,.T.);
#31251=EDGE_CURVE('',#24274,#24275,#5737,.T.);
#31252=EDGE_CURVE('',#24275,#24273,#5738,.T.);
#31253=EDGE_CURVE('',#24276,#24274,#5739,.T.);
#31254=EDGE_CURVE('',#24276,#24277,#5740,.T.);
#31255=EDGE_CURVE('',#24277,#24275,#5741,.T.);
#31256=EDGE_CURVE('',#24278,#24276,#5742,.T.);
#31257=EDGE_CURVE('',#24278,#24279,#5743,.T.);
#31258=EDGE_CURVE('',#24279,#24277,#5744,.T.);
#31259=EDGE_CURVE('',#24280,#24278,#5745,.T.);
#31260=EDGE_CURVE('',#24280,#24281,#5746,.T.);
#31261=EDGE_CURVE('',#24281,#24279,#5747,.T.);
#31262=EDGE_CURVE('',#24282,#24280,#5748,.T.);
#31263=EDGE_CURVE('',#24282,#24283,#5749,.T.);
#31264=EDGE_CURVE('',#24283,#24281,#5750,.T.);
#31265=EDGE_CURVE('',#24284,#24282,#5751,.T.);
#31266=EDGE_CURVE('',#24284,#24285,#5752,.T.);
#31267=EDGE_CURVE('',#24285,#24283,#5753,.T.);
#31268=EDGE_CURVE('',#24286,#24284,#5754,.T.);
#31269=EDGE_CURVE('',#24286,#24287,#5755,.T.);
#31270=EDGE_CURVE('',#24287,#24285,#5756,.T.);
#31271=EDGE_CURVE('',#24288,#24286,#5757,.T.);
#31272=EDGE_CURVE('',#24288,#24289,#5758,.T.);
#31273=EDGE_CURVE('',#24289,#24287,#5759,.T.);
#31274=EDGE_CURVE('',#24267,#24288,#5760,.T.);
#31275=EDGE_CURVE('',#24269,#24289,#5761,.T.);
#31276=EDGE_CURVE('',#24290,#24291,#5762,.T.);
#31277=EDGE_CURVE('',#24290,#24292,#5763,.T.);
#31278=EDGE_CURVE('',#24292,#24293,#5764,.T.);
#31279=EDGE_CURVE('',#24291,#24293,#5765,.T.);
#31280=EDGE_CURVE('',#24294,#24290,#5766,.T.);
#31281=EDGE_CURVE('',#24294,#24295,#5767,.T.);
#31282=EDGE_CURVE('',#24295,#24292,#5768,.T.);
#31283=EDGE_CURVE('',#24296,#24294,#5769,.T.);
#31284=EDGE_CURVE('',#24296,#24297,#5770,.T.);
#31285=EDGE_CURVE('',#24297,#24295,#5771,.T.);
#31286=EDGE_CURVE('',#24291,#24296,#5772,.T.);
#31287=EDGE_CURVE('',#24293,#24297,#5773,.T.);
#31288=EDGE_CURVE('',#24298,#24299,#417,.T.);
#31289=EDGE_CURVE('',#24298,#24300,#5774,.T.);
#31290=EDGE_CURVE('',#24300,#24301,#418,.T.);
#31291=EDGE_CURVE('',#24299,#24301,#5775,.T.);
#31292=EDGE_CURVE('',#24302,#24298,#419,.T.);
#31293=EDGE_CURVE('',#24302,#24303,#5776,.T.);
#31294=EDGE_CURVE('',#24303,#24300,#420,.T.);
#31295=EDGE_CURVE('',#24304,#24302,#421,.T.);
#31296=EDGE_CURVE('',#24304,#24305,#5777,.T.);
#31297=EDGE_CURVE('',#24305,#24303,#422,.T.);
#31298=EDGE_CURVE('',#24306,#24304,#423,.T.);
#31299=EDGE_CURVE('',#24306,#24307,#5778,.T.);
#31300=EDGE_CURVE('',#24307,#24305,#424,.T.);
#31301=EDGE_CURVE('',#24308,#24306,#425,.T.);
#31302=EDGE_CURVE('',#24308,#24309,#5779,.T.);
#31303=EDGE_CURVE('',#24309,#24307,#426,.T.);
#31304=EDGE_CURVE('',#24310,#24308,#427,.T.);
#31305=EDGE_CURVE('',#24310,#24311,#5780,.T.);
#31306=EDGE_CURVE('',#24311,#24309,#428,.T.);
#31307=EDGE_CURVE('',#24312,#24310,#429,.T.);
#31308=EDGE_CURVE('',#24312,#24313,#5781,.T.);
#31309=EDGE_CURVE('',#24313,#24311,#430,.T.);
#31310=EDGE_CURVE('',#24314,#24312,#431,.T.);
#31311=EDGE_CURVE('',#24314,#24315,#5782,.T.);
#31312=EDGE_CURVE('',#24315,#24313,#432,.T.);
#31313=EDGE_CURVE('',#24316,#24314,#433,.T.);
#31314=EDGE_CURVE('',#24316,#24317,#5783,.T.);
#31315=EDGE_CURVE('',#24317,#24315,#434,.T.);
#31316=EDGE_CURVE('',#24318,#24316,#435,.T.);
#31317=EDGE_CURVE('',#24318,#24319,#5784,.T.);
#31318=EDGE_CURVE('',#24319,#24317,#436,.T.);
#31319=EDGE_CURVE('',#24299,#24318,#437,.T.);
#31320=EDGE_CURVE('',#24301,#24319,#438,.T.);
#31321=EDGE_CURVE('',#24320,#24321,#5785,.T.);
#31322=EDGE_CURVE('',#24320,#24322,#5786,.T.);
#31323=EDGE_CURVE('',#24322,#24323,#5787,.T.);
#31324=EDGE_CURVE('',#24321,#24323,#5788,.T.);
#31325=EDGE_CURVE('',#24324,#24320,#5789,.T.);
#31326=EDGE_CURVE('',#24324,#24325,#5790,.T.);
#31327=EDGE_CURVE('',#24325,#24322,#5791,.T.);
#31328=EDGE_CURVE('',#24326,#24324,#5792,.T.);
#31329=EDGE_CURVE('',#24326,#24327,#5793,.T.);
#31330=EDGE_CURVE('',#24327,#24325,#5794,.T.);
#31331=EDGE_CURVE('',#24328,#24326,#5795,.T.);
#31332=EDGE_CURVE('',#24328,#24329,#5796,.T.);
#31333=EDGE_CURVE('',#24329,#24327,#5797,.T.);
#31334=EDGE_CURVE('',#24330,#24328,#5798,.T.);
#31335=EDGE_CURVE('',#24330,#24331,#5799,.T.);
#31336=EDGE_CURVE('',#24331,#24329,#5800,.T.);
#31337=EDGE_CURVE('',#24332,#24330,#5801,.T.);
#31338=EDGE_CURVE('',#24332,#24333,#5802,.T.);
#31339=EDGE_CURVE('',#24333,#24331,#5803,.T.);
#31340=EDGE_CURVE('',#24334,#24332,#5804,.T.);
#31341=EDGE_CURVE('',#24334,#24335,#5805,.T.);
#31342=EDGE_CURVE('',#24335,#24333,#5806,.T.);
#31343=EDGE_CURVE('',#24336,#24334,#5807,.T.);
#31344=EDGE_CURVE('',#24336,#24337,#5808,.T.);
#31345=EDGE_CURVE('',#24337,#24335,#5809,.T.);
#31346=EDGE_CURVE('',#24338,#24336,#5810,.T.);
#31347=EDGE_CURVE('',#24338,#24339,#5811,.T.);
#31348=EDGE_CURVE('',#24339,#24337,#5812,.T.);
#31349=EDGE_CURVE('',#24340,#24338,#5813,.T.);
#31350=EDGE_CURVE('',#24340,#24341,#5814,.T.);
#31351=EDGE_CURVE('',#24341,#24339,#5815,.T.);
#31352=EDGE_CURVE('',#24342,#24340,#5816,.T.);
#31353=EDGE_CURVE('',#24342,#24343,#5817,.T.);
#31354=EDGE_CURVE('',#24343,#24341,#5818,.T.);
#31355=EDGE_CURVE('',#24321,#24342,#5819,.T.);
#31356=EDGE_CURVE('',#24323,#24343,#5820,.T.);
#31357=EDGE_CURVE('',#24344,#24345,#5821,.T.);
#31358=EDGE_CURVE('',#24344,#24346,#5822,.T.);
#31359=EDGE_CURVE('',#24346,#24347,#5823,.T.);
#31360=EDGE_CURVE('',#24345,#24347,#5824,.T.);
#31361=EDGE_CURVE('',#24348,#24344,#5825,.T.);
#31362=EDGE_CURVE('',#24348,#24349,#5826,.T.);
#31363=EDGE_CURVE('',#24349,#24346,#5827,.T.);
#31364=EDGE_CURVE('',#24350,#24348,#5828,.T.);
#31365=EDGE_CURVE('',#24350,#24351,#5829,.T.);
#31366=EDGE_CURVE('',#24351,#24349,#5830,.T.);
#31367=EDGE_CURVE('',#24352,#24350,#5831,.T.);
#31368=EDGE_CURVE('',#24352,#24353,#5832,.T.);
#31369=EDGE_CURVE('',#24353,#24351,#5833,.T.);
#31370=EDGE_CURVE('',#24354,#24352,#5834,.T.);
#31371=EDGE_CURVE('',#24354,#24355,#5835,.T.);
#31372=EDGE_CURVE('',#24355,#24353,#5836,.T.);
#31373=EDGE_CURVE('',#24345,#24354,#5837,.T.);
#31374=EDGE_CURVE('',#24347,#24355,#5838,.T.);
#31375=EDGE_CURVE('',#24356,#24357,#439,.T.);
#31376=EDGE_CURVE('',#24356,#24358,#5839,.T.);
#31377=EDGE_CURVE('',#24358,#24359,#440,.T.);
#31378=EDGE_CURVE('',#24357,#24359,#5840,.T.);
#31379=EDGE_CURVE('',#24360,#24356,#441,.T.);
#31380=EDGE_CURVE('',#24360,#24361,#5841,.T.);
#31381=EDGE_CURVE('',#24361,#24358,#442,.T.);
#31382=EDGE_CURVE('',#24362,#24360,#443,.T.);
#31383=EDGE_CURVE('',#24362,#24363,#5842,.T.);
#31384=EDGE_CURVE('',#24363,#24361,#444,.T.);
#31385=EDGE_CURVE('',#24364,#24362,#445,.T.);
#31386=EDGE_CURVE('',#24364,#24365,#5843,.T.);
#31387=EDGE_CURVE('',#24365,#24363,#446,.T.);
#31388=EDGE_CURVE('',#24366,#24364,#447,.T.);
#31389=EDGE_CURVE('',#24366,#24367,#5844,.T.);
#31390=EDGE_CURVE('',#24367,#24365,#448,.T.);
#31391=EDGE_CURVE('',#24368,#24366,#449,.T.);
#31392=EDGE_CURVE('',#24368,#24369,#5845,.T.);
#31393=EDGE_CURVE('',#24369,#24367,#450,.T.);
#31394=EDGE_CURVE('',#24370,#24368,#451,.T.);
#31395=EDGE_CURVE('',#24370,#24371,#5846,.T.);
#31396=EDGE_CURVE('',#24371,#24369,#452,.T.);
#31397=EDGE_CURVE('',#24372,#24370,#453,.T.);
#31398=EDGE_CURVE('',#24372,#24373,#5847,.T.);
#31399=EDGE_CURVE('',#24373,#24371,#454,.T.);
#31400=EDGE_CURVE('',#24374,#24372,#5848,.T.);
#31401=EDGE_CURVE('',#24374,#24375,#5849,.T.);
#31402=EDGE_CURVE('',#24375,#24373,#5850,.T.);
#31403=EDGE_CURVE('',#24376,#24374,#5851,.T.);
#31404=EDGE_CURVE('',#24376,#24377,#5852,.T.);
#31405=EDGE_CURVE('',#24377,#24375,#5853,.T.);
#31406=EDGE_CURVE('',#24378,#24376,#5854,.T.);
#31407=EDGE_CURVE('',#24378,#24379,#5855,.T.);
#31408=EDGE_CURVE('',#24379,#24377,#5856,.T.);
#31409=EDGE_CURVE('',#24357,#24378,#455,.T.);
#31410=EDGE_CURVE('',#24359,#24379,#456,.T.);
#31411=EDGE_CURVE('',#24380,#24381,#5857,.T.);
#31412=EDGE_CURVE('',#24380,#24382,#5858,.T.);
#31413=EDGE_CURVE('',#24382,#24383,#5859,.T.);
#31414=EDGE_CURVE('',#24381,#24383,#5860,.T.);
#31415=EDGE_CURVE('',#24384,#24380,#457,.T.);
#31416=EDGE_CURVE('',#24384,#24385,#5861,.T.);
#31417=EDGE_CURVE('',#24385,#24382,#458,.T.);
#31418=EDGE_CURVE('',#24386,#24384,#459,.T.);
#31419=EDGE_CURVE('',#24386,#24387,#5862,.T.);
#31420=EDGE_CURVE('',#24387,#24385,#460,.T.);
#31421=EDGE_CURVE('',#24388,#24386,#461,.T.);
#31422=EDGE_CURVE('',#24388,#24389,#5863,.T.);
#31423=EDGE_CURVE('',#24389,#24387,#462,.T.);
#31424=EDGE_CURVE('',#24390,#24388,#463,.T.);
#31425=EDGE_CURVE('',#24390,#24391,#5864,.T.);
#31426=EDGE_CURVE('',#24391,#24389,#464,.T.);
#31427=EDGE_CURVE('',#24392,#24390,#5865,.T.);
#31428=EDGE_CURVE('',#24392,#24393,#5866,.T.);
#31429=EDGE_CURVE('',#24393,#24391,#5867,.T.);
#31430=EDGE_CURVE('',#24394,#24392,#5868,.T.);
#31431=EDGE_CURVE('',#24394,#24395,#5869,.T.);
#31432=EDGE_CURVE('',#24395,#24393,#5870,.T.);
#31433=EDGE_CURVE('',#24396,#24394,#5871,.T.);
#31434=EDGE_CURVE('',#24396,#24397,#5872,.T.);
#31435=EDGE_CURVE('',#24397,#24395,#5873,.T.);
#31436=EDGE_CURVE('',#24398,#24396,#465,.T.);
#31437=EDGE_CURVE('',#24398,#24399,#5874,.T.);
#31438=EDGE_CURVE('',#24399,#24397,#466,.T.);
#31439=EDGE_CURVE('',#24400,#24398,#467,.T.);
#31440=EDGE_CURVE('',#24400,#24401,#5875,.T.);
#31441=EDGE_CURVE('',#24401,#24399,#468,.T.);
#31442=EDGE_CURVE('',#24402,#24400,#469,.T.);
#31443=EDGE_CURVE('',#24402,#24403,#5876,.T.);
#31444=EDGE_CURVE('',#24403,#24401,#470,.T.);
#31445=EDGE_CURVE('',#24404,#24402,#471,.T.);
#31446=EDGE_CURVE('',#24404,#24405,#5877,.T.);
#31447=EDGE_CURVE('',#24405,#24403,#472,.T.);
#31448=EDGE_CURVE('',#24406,#24404,#473,.T.);
#31449=EDGE_CURVE('',#24406,#24407,#5878,.T.);
#31450=EDGE_CURVE('',#24407,#24405,#474,.T.);
#31451=EDGE_CURVE('',#24408,#24406,#475,.T.);
#31452=EDGE_CURVE('',#24408,#24409,#5879,.T.);
#31453=EDGE_CURVE('',#24409,#24407,#476,.T.);
#31454=EDGE_CURVE('',#24410,#24408,#477,.T.);
#31455=EDGE_CURVE('',#24410,#24411,#5880,.T.);
#31456=EDGE_CURVE('',#24411,#24409,#478,.T.);
#31457=EDGE_CURVE('',#24412,#24410,#5881,.T.);
#31458=EDGE_CURVE('',#24412,#24413,#5882,.T.);
#31459=EDGE_CURVE('',#24413,#24411,#5883,.T.);
#31460=EDGE_CURVE('',#24414,#24412,#5884,.T.);
#31461=EDGE_CURVE('',#24414,#24415,#5885,.T.);
#31462=EDGE_CURVE('',#24415,#24413,#5886,.T.);
#31463=EDGE_CURVE('',#24416,#24414,#5887,.T.);
#31464=EDGE_CURVE('',#24416,#24417,#5888,.T.);
#31465=EDGE_CURVE('',#24417,#24415,#5889,.T.);
#31466=EDGE_CURVE('',#24381,#24416,#5890,.T.);
#31467=EDGE_CURVE('',#24383,#24417,#5891,.T.);
#31468=EDGE_CURVE('',#24418,#24419,#5892,.T.);
#31469=EDGE_CURVE('',#24420,#24418,#5893,.T.);
#31470=EDGE_CURVE('',#24421,#24420,#5894,.T.);
#31471=EDGE_CURVE('',#24421,#24419,#5895,.T.);
#31472=EDGE_CURVE('',#24419,#24422,#5896,.T.);
#31473=EDGE_CURVE('',#24423,#24421,#5897,.T.);
#31474=EDGE_CURVE('',#24423,#24422,#5898,.T.);
#31475=EDGE_CURVE('',#24422,#24424,#5899,.T.);
#31476=EDGE_CURVE('',#24425,#24423,#5900,.T.);
#31477=EDGE_CURVE('',#24425,#24424,#5901,.T.);
#31478=EDGE_CURVE('',#24424,#24418,#5902,.T.);
#31479=EDGE_CURVE('',#24420,#24425,#5903,.T.);
#31480=EDGE_CURVE('',#24426,#24426,#19951,.T.);
#31481=EDGE_CURVE('',#24426,#24427,#5904,.T.);
#31482=EDGE_CURVE('',#24427,#24427,#19952,.T.);
#31483=EDGE_CURVE('',#24428,#24428,#19953,.T.);
#31484=EDGE_CURVE('',#24428,#24427,#5905,.T.);
#31485=EDGE_CURVE('',#24429,#24430,#5906,.T.);
#31486=EDGE_CURVE('',#24431,#24429,#19954,.T.);
#31487=EDGE_CURVE('',#24432,#24431,#5907,.T.);
#31488=EDGE_CURVE('',#24433,#24432,#19955,.T.);
#31489=EDGE_CURVE('',#24434,#24433,#5908,.T.);
#31490=EDGE_CURVE('',#24435,#24434,#19956,.T.);
#31491=EDGE_CURVE('',#24436,#24435,#5909,.T.);
#31492=EDGE_CURVE('',#24430,#24436,#19957,.T.);
#31493=EDGE_CURVE('',#24437,#24437,#19958,.T.);
#31494=EDGE_CURVE('',#24438,#24438,#19959,.T.);
#31495=EDGE_CURVE('',#24439,#24439,#19960,.T.);
#31496=EDGE_CURVE('',#24440,#24440,#19961,.T.);
#31497=EDGE_CURVE('',#24441,#24441,#19962,.T.);
#31498=EDGE_CURVE('',#24442,#24442,#19963,.T.);
#31499=EDGE_CURVE('',#24443,#24443,#19964,.T.);
#31500=EDGE_CURVE('',#24444,#24444,#19965,.T.);
#31501=EDGE_CURVE('',#24445,#24445,#19966,.T.);
#31502=EDGE_CURVE('',#24446,#24446,#19967,.T.);
#31503=EDGE_CURVE('',#24447,#24447,#19968,.T.);
#31504=EDGE_CURVE('',#24447,#24428,#5910,.T.);
#31505=EDGE_CURVE('',#24448,#24449,#19969,.T.);
#31506=EDGE_CURVE('',#24450,#24448,#5911,.T.);
#31507=EDGE_CURVE('',#24451,#24450,#19970,.T.);
#31508=EDGE_CURVE('',#24452,#24451,#5912,.T.);
#31509=EDGE_CURVE('',#24453,#24452,#19971,.T.);
#31510=EDGE_CURVE('',#24454,#24453,#5913,.T.);
#31511=EDGE_CURVE('',#24455,#24454,#19972,.T.);
#31512=EDGE_CURVE('',#24449,#24455,#5914,.T.);
#31513=EDGE_CURVE('',#24456,#24456,#19973,.T.);
#31514=EDGE_CURVE('',#24457,#24457,#19974,.T.);
#31515=EDGE_CURVE('',#24458,#24458,#19975,.T.);
#31516=EDGE_CURVE('',#24446,#24459,#5915,.T.);
#31517=EDGE_CURVE('',#24459,#24459,#19976,.T.);
#31518=EDGE_CURVE('',#24460,#24460,#19977,.T.);
#31519=EDGE_CURVE('',#24460,#24459,#5916,.T.);
#31520=EDGE_CURVE('',#24456,#24460,#5917,.T.);
#31521=EDGE_CURVE('',#24437,#24461,#5918,.T.);
#31522=EDGE_CURVE('',#24461,#24461,#19978,.T.);
#31523=EDGE_CURVE('',#24462,#24462,#19979,.T.);
#31524=EDGE_CURVE('',#24462,#24461,#5919,.T.);
#31525=EDGE_CURVE('',#24458,#24462,#5920,.T.);
#31526=EDGE_CURVE('',#24445,#24463,#5921,.T.);
#31527=EDGE_CURVE('',#24463,#24463,#19980,.T.);
#31528=EDGE_CURVE('',#24464,#24464,#19981,.T.);
#31529=EDGE_CURVE('',#24464,#24463,#5922,.T.);
#31530=EDGE_CURVE('',#24457,#24464,#5923,.T.);
#31531=EDGE_CURVE('',#24465,#24465,#19982,.T.);
#31532=EDGE_CURVE('',#24465,#24466,#5924,.T.);
#31533=EDGE_CURVE('',#24444,#24465,#5925,.T.);
#31534=EDGE_CURVE('',#24467,#24467,#19983,.T.);
#31535=EDGE_CURVE('',#24467,#24468,#5926,.T.);
#31536=EDGE_CURVE('',#24443,#24467,#5927,.T.);
#31537=EDGE_CURVE('',#24469,#24469,#19984,.T.);
#31538=EDGE_CURVE('',#24469,#24470,#5928,.T.);
#31539=EDGE_CURVE('',#24438,#24471,#5929,.T.);
#31540=EDGE_CURVE('',#24471,#24471,#19985,.T.);
#31541=EDGE_CURVE('',#24471,#24469,#5930,.T.);
#31542=EDGE_CURVE('',#24472,#24472,#19986,.T.);
#31543=EDGE_CURVE('',#24472,#24473,#5931,.T.);
#31544=EDGE_CURVE('',#24439,#24474,#5932,.T.);
#31545=EDGE_CURVE('',#24474,#24474,#19987,.T.);
#31546=EDGE_CURVE('',#24474,#24472,#5933,.T.);
#31547=EDGE_CURVE('',#24475,#24475,#19988,.T.);
#31548=EDGE_CURVE('',#24475,#24476,#5934,.T.);
#31549=EDGE_CURVE('',#24440,#24477,#5935,.T.);
#31550=EDGE_CURVE('',#24477,#24477,#19989,.T.);
#31551=EDGE_CURVE('',#24477,#24475,#5936,.T.);
#31552=EDGE_CURVE('',#24478,#24478,#19990,.T.);
#31553=EDGE_CURVE('',#24478,#24479,#5937,.T.);
#31554=EDGE_CURVE('',#24441,#24480,#5938,.T.);
#31555=EDGE_CURVE('',#24480,#24480,#19991,.T.);
#31556=EDGE_CURVE('',#24480,#24478,#5939,.T.);
#31557=EDGE_CURVE('',#24481,#24481,#19992,.T.);
#31558=EDGE_CURVE('',#24481,#24442,#5940,.T.);
#31559=EDGE_CURVE('',#24449,#24482,#5941,.T.);
#31560=EDGE_CURVE('',#24482,#24483,#19993,.T.);
#31561=EDGE_CURVE('',#24483,#24448,#5942,.T.);
#31562=EDGE_CURVE('',#24455,#24484,#5943,.T.);
#31563=EDGE_CURVE('',#24484,#24482,#5944,.T.);
#31564=EDGE_CURVE('',#24454,#24485,#5945,.T.);
#31565=EDGE_CURVE('',#24485,#24484,#19994,.T.);
#31566=EDGE_CURVE('',#24453,#24486,#5946,.T.);
#31567=EDGE_CURVE('',#24486,#24485,#5947,.T.);
#31568=EDGE_CURVE('',#24452,#24487,#5948,.T.);
#31569=EDGE_CURVE('',#24487,#24486,#19995,.T.);
#31570=EDGE_CURVE('',#24451,#24488,#5949,.T.);
#31571=EDGE_CURVE('',#24488,#24487,#5950,.T.);
#31572=EDGE_CURVE('',#24450,#24489,#5951,.T.);
#31573=EDGE_CURVE('',#24489,#24488,#19996,.T.);
#31574=EDGE_CURVE('',#24483,#24489,#5952,.T.);
#31575=EDGE_CURVE('',#24488,#24490,#5953,.T.);
#31576=EDGE_CURVE('',#24491,#24490,#5954,.T.);
#31577=EDGE_CURVE('',#24487,#24491,#5955,.T.);
#31578=EDGE_CURVE('',#24489,#24492,#5956,.T.);
#31579=EDGE_CURVE('',#24490,#24492,#19997,.T.);
#31580=EDGE_CURVE('',#24483,#24493,#5957,.T.);
#31581=EDGE_CURVE('',#24492,#24493,#5958,.T.);
#31582=EDGE_CURVE('',#24482,#24494,#5959,.T.);
#31583=EDGE_CURVE('',#24493,#24494,#19998,.T.);
#31584=EDGE_CURVE('',#24490,#24429,#5960,.T.);
#31585=EDGE_CURVE('',#24430,#24491,#5961,.T.);
#31586=EDGE_CURVE('',#24492,#24431,#5962,.T.);
#31587=EDGE_CURVE('',#24493,#24432,#5963,.T.);
#31588=EDGE_CURVE('',#24494,#24433,#5964,.T.);
#31589=EDGE_CURVE('',#24495,#24434,#5965,.T.);
#31590=EDGE_CURVE('',#24494,#24495,#5966,.T.);
#31591=EDGE_CURVE('',#24496,#24435,#5967,.T.);
#31592=EDGE_CURVE('',#24495,#24496,#19999,.T.);
#31593=EDGE_CURVE('',#24497,#24436,#5968,.T.);
#31594=EDGE_CURVE('',#24496,#24497,#5969,.T.);
#31595=EDGE_CURVE('',#24497,#24491,#20000,.T.);
#31596=EDGE_CURVE('',#24486,#24497,#5970,.T.);
#31597=EDGE_CURVE('',#24485,#24496,#5971,.T.);
#31598=EDGE_CURVE('',#24484,#24495,#5972,.T.);
#43479=ORIENTED_EDGE('',*,*,#30601,.F.);
#43480=ORIENTED_EDGE('',*,*,#30602,.T.);
#43481=ORIENTED_EDGE('',*,*,#30603,.T.);
#43482=ORIENTED_EDGE('',*,*,#30604,.F.);
#43483=ORIENTED_EDGE('',*,*,#30605,.F.);
#43484=ORIENTED_EDGE('',*,*,#30606,.T.);
#43485=ORIENTED_EDGE('',*,*,#30607,.T.);
#43486=ORIENTED_EDGE('',*,*,#30602,.F.);
#43487=ORIENTED_EDGE('',*,*,#30608,.F.);
#43488=ORIENTED_EDGE('',*,*,#30609,.T.);
#43489=ORIENTED_EDGE('',*,*,#30610,.T.);
#43490=ORIENTED_EDGE('',*,*,#30606,.F.);
#43491=ORIENTED_EDGE('',*,*,#30611,.F.);
#43492=ORIENTED_EDGE('',*,*,#30612,.T.);
#43493=ORIENTED_EDGE('',*,*,#30613,.T.);
#43494=ORIENTED_EDGE('',*,*,#30609,.F.);
#43495=ORIENTED_EDGE('',*,*,#30614,.F.);
#43496=ORIENTED_EDGE('',*,*,#30615,.T.);
#43497=ORIENTED_EDGE('',*,*,#30616,.T.);
#43498=ORIENTED_EDGE('',*,*,#30612,.F.);
#43499=ORIENTED_EDGE('',*,*,#30617,.F.);
#43500=ORIENTED_EDGE('',*,*,#30618,.T.);
#43501=ORIENTED_EDGE('',*,*,#30619,.T.);
#43502=ORIENTED_EDGE('',*,*,#30615,.F.);
#43503=ORIENTED_EDGE('',*,*,#30620,.F.);
#43504=ORIENTED_EDGE('',*,*,#30621,.T.);
#43505=ORIENTED_EDGE('',*,*,#30622,.T.);
#43506=ORIENTED_EDGE('',*,*,#30618,.F.);
#43507=ORIENTED_EDGE('',*,*,#30623,.F.);
#43508=ORIENTED_EDGE('',*,*,#30624,.T.);
#43509=ORIENTED_EDGE('',*,*,#30625,.T.);
#43510=ORIENTED_EDGE('',*,*,#30621,.F.);
#43511=ORIENTED_EDGE('',*,*,#30626,.F.);
#43512=ORIENTED_EDGE('',*,*,#30627,.T.);
#43513=ORIENTED_EDGE('',*,*,#30628,.T.);
#43514=ORIENTED_EDGE('',*,*,#30624,.F.);
#43515=ORIENTED_EDGE('',*,*,#30629,.F.);
#43516=ORIENTED_EDGE('',*,*,#30630,.T.);
#43517=ORIENTED_EDGE('',*,*,#30631,.T.);
#43518=ORIENTED_EDGE('',*,*,#30627,.F.);
#43519=ORIENTED_EDGE('',*,*,#30632,.F.);
#43520=ORIENTED_EDGE('',*,*,#30633,.T.);
#43521=ORIENTED_EDGE('',*,*,#30634,.T.);
#43522=ORIENTED_EDGE('',*,*,#30630,.F.);
#43523=ORIENTED_EDGE('',*,*,#30635,.F.);
#43524=ORIENTED_EDGE('',*,*,#30604,.T.);
#43525=ORIENTED_EDGE('',*,*,#30636,.T.);
#43526=ORIENTED_EDGE('',*,*,#30633,.F.);
#43527=ORIENTED_EDGE('',*,*,#30636,.F.);
#43528=ORIENTED_EDGE('',*,*,#30603,.F.);
#43529=ORIENTED_EDGE('',*,*,#30607,.F.);
#43530=ORIENTED_EDGE('',*,*,#30610,.F.);
#43531=ORIENTED_EDGE('',*,*,#30613,.F.);
#43532=ORIENTED_EDGE('',*,*,#30616,.F.);
#43533=ORIENTED_EDGE('',*,*,#30619,.F.);
#43534=ORIENTED_EDGE('',*,*,#30622,.F.);
#43535=ORIENTED_EDGE('',*,*,#30625,.F.);
#43536=ORIENTED_EDGE('',*,*,#30628,.F.);
#43537=ORIENTED_EDGE('',*,*,#30631,.F.);
#43538=ORIENTED_EDGE('',*,*,#30634,.F.);
#43539=ORIENTED_EDGE('',*,*,#30637,.F.);
#43540=ORIENTED_EDGE('',*,*,#30638,.T.);
#43541=ORIENTED_EDGE('',*,*,#30639,.T.);
#43542=ORIENTED_EDGE('',*,*,#30640,.F.);
#43543=ORIENTED_EDGE('',*,*,#30641,.F.);
#43544=ORIENTED_EDGE('',*,*,#30642,.T.);
#43545=ORIENTED_EDGE('',*,*,#30643,.T.);
#43546=ORIENTED_EDGE('',*,*,#30638,.F.);
#43547=ORIENTED_EDGE('',*,*,#30644,.F.);
#43548=ORIENTED_EDGE('',*,*,#30645,.T.);
#43549=ORIENTED_EDGE('',*,*,#30646,.T.);
#43550=ORIENTED_EDGE('',*,*,#30642,.F.);
#43551=ORIENTED_EDGE('',*,*,#30647,.F.);
#43552=ORIENTED_EDGE('',*,*,#30640,.T.);
#43553=ORIENTED_EDGE('',*,*,#30648,.T.);
#43554=ORIENTED_EDGE('',*,*,#30645,.F.);
#43555=ORIENTED_EDGE('',*,*,#30648,.F.);
#43556=ORIENTED_EDGE('',*,*,#30639,.F.);
#43557=ORIENTED_EDGE('',*,*,#30643,.F.);
#43558=ORIENTED_EDGE('',*,*,#30646,.F.);
#43559=ORIENTED_EDGE('',*,*,#30649,.F.);
#43560=ORIENTED_EDGE('',*,*,#30650,.T.);
#43561=ORIENTED_EDGE('',*,*,#30651,.T.);
#43562=ORIENTED_EDGE('',*,*,#30652,.F.);
#43563=ORIENTED_EDGE('',*,*,#30653,.F.);
#43564=ORIENTED_EDGE('',*,*,#30654,.T.);
#43565=ORIENTED_EDGE('',*,*,#30655,.T.);
#43566=ORIENTED_EDGE('',*,*,#30650,.F.);
#43567=ORIENTED_EDGE('',*,*,#30656,.F.);
#43568=ORIENTED_EDGE('',*,*,#30657,.T.);
#43569=ORIENTED_EDGE('',*,*,#30658,.T.);
#43570=ORIENTED_EDGE('',*,*,#30654,.F.);
#43571=ORIENTED_EDGE('',*,*,#30659,.F.);
#43572=ORIENTED_EDGE('',*,*,#30660,.T.);
#43573=ORIENTED_EDGE('',*,*,#30661,.T.);
#43574=ORIENTED_EDGE('',*,*,#30657,.F.);
#43575=ORIENTED_EDGE('',*,*,#30662,.F.);
#43576=ORIENTED_EDGE('',*,*,#30663,.T.);
#43577=ORIENTED_EDGE('',*,*,#30664,.T.);
#43578=ORIENTED_EDGE('',*,*,#30660,.F.);
#43579=ORIENTED_EDGE('',*,*,#30665,.F.);
#43580=ORIENTED_EDGE('',*,*,#30666,.T.);
#43581=ORIENTED_EDGE('',*,*,#30667,.T.);
#43582=ORIENTED_EDGE('',*,*,#30663,.F.);
#43583=ORIENTED_EDGE('',*,*,#30668,.F.);
#43584=ORIENTED_EDGE('',*,*,#30669,.T.);
#43585=ORIENTED_EDGE('',*,*,#30670,.T.);
#43586=ORIENTED_EDGE('',*,*,#30666,.F.);
#43587=ORIENTED_EDGE('',*,*,#30671,.F.);
#43588=ORIENTED_EDGE('',*,*,#30672,.T.);
#43589=ORIENTED_EDGE('',*,*,#30673,.T.);
#43590=ORIENTED_EDGE('',*,*,#30669,.F.);
#43591=ORIENTED_EDGE('',*,*,#30674,.F.);
#43592=ORIENTED_EDGE('',*,*,#30675,.T.);
#43593=ORIENTED_EDGE('',*,*,#30676,.T.);
#43594=ORIENTED_EDGE('',*,*,#30672,.F.);
#43595=ORIENTED_EDGE('',*,*,#30677,.F.);
#43596=ORIENTED_EDGE('',*,*,#30678,.T.);
#43597=ORIENTED_EDGE('',*,*,#30679,.T.);
#43598=ORIENTED_EDGE('',*,*,#30675,.F.);
#43599=ORIENTED_EDGE('',*,*,#30680,.F.);
#43600=ORIENTED_EDGE('',*,*,#30681,.T.);
#43601=ORIENTED_EDGE('',*,*,#30682,.T.);
#43602=ORIENTED_EDGE('',*,*,#30678,.F.);
#43603=ORIENTED_EDGE('',*,*,#30683,.F.);
#43604=ORIENTED_EDGE('',*,*,#30684,.T.);
#43605=ORIENTED_EDGE('',*,*,#30685,.T.);
#43606=ORIENTED_EDGE('',*,*,#30681,.F.);
#43607=ORIENTED_EDGE('',*,*,#30686,.F.);
#43608=ORIENTED_EDGE('',*,*,#30687,.T.);
#43609=ORIENTED_EDGE('',*,*,#30688,.T.);
#43610=ORIENTED_EDGE('',*,*,#30684,.F.);
#43611=ORIENTED_EDGE('',*,*,#30689,.F.);
#43612=ORIENTED_EDGE('',*,*,#30690,.T.);
#43613=ORIENTED_EDGE('',*,*,#30691,.T.);
#43614=ORIENTED_EDGE('',*,*,#30687,.F.);
#43615=ORIENTED_EDGE('',*,*,#30692,.F.);
#43616=ORIENTED_EDGE('',*,*,#30693,.T.);
#43617=ORIENTED_EDGE('',*,*,#30694,.T.);
#43618=ORIENTED_EDGE('',*,*,#30690,.F.);
#43619=ORIENTED_EDGE('',*,*,#30695,.F.);
#43620=ORIENTED_EDGE('',*,*,#30696,.T.);
#43621=ORIENTED_EDGE('',*,*,#30697,.T.);
#43622=ORIENTED_EDGE('',*,*,#30693,.F.);
#43623=ORIENTED_EDGE('',*,*,#30698,.F.);
#43624=ORIENTED_EDGE('',*,*,#30699,.T.);
#43625=ORIENTED_EDGE('',*,*,#30700,.T.);
#43626=ORIENTED_EDGE('',*,*,#30696,.F.);
#43627=ORIENTED_EDGE('',*,*,#30701,.F.);
#43628=ORIENTED_EDGE('',*,*,#30702,.T.);
#43629=ORIENTED_EDGE('',*,*,#30703,.T.);
#43630=ORIENTED_EDGE('',*,*,#30699,.F.);
#43631=ORIENTED_EDGE('',*,*,#30704,.F.);
#43632=ORIENTED_EDGE('',*,*,#30705,.T.);
#43633=ORIENTED_EDGE('',*,*,#30706,.T.);
#43634=ORIENTED_EDGE('',*,*,#30702,.F.);
#43635=ORIENTED_EDGE('',*,*,#30707,.F.);
#43636=ORIENTED_EDGE('',*,*,#30708,.T.);
#43637=ORIENTED_EDGE('',*,*,#30709,.T.);
#43638=ORIENTED_EDGE('',*,*,#30705,.F.);
#43639=ORIENTED_EDGE('',*,*,#30710,.F.);
#43640=ORIENTED_EDGE('',*,*,#30711,.T.);
#43641=ORIENTED_EDGE('',*,*,#30712,.T.);
#43642=ORIENTED_EDGE('',*,*,#30708,.F.);
#43643=ORIENTED_EDGE('',*,*,#30713,.F.);
#43644=ORIENTED_EDGE('',*,*,#30714,.T.);
#43645=ORIENTED_EDGE('',*,*,#30715,.T.);
#43646=ORIENTED_EDGE('',*,*,#30711,.F.);
#43647=ORIENTED_EDGE('',*,*,#30716,.F.);
#43648=ORIENTED_EDGE('',*,*,#30717,.T.);
#43649=ORIENTED_EDGE('',*,*,#30718,.T.);
#43650=ORIENTED_EDGE('',*,*,#30714,.F.);
#43651=ORIENTED_EDGE('',*,*,#30719,.F.);
#43652=ORIENTED_EDGE('',*,*,#30720,.T.);
#43653=ORIENTED_EDGE('',*,*,#30721,.T.);
#43654=ORIENTED_EDGE('',*,*,#30717,.F.);
#43655=ORIENTED_EDGE('',*,*,#30722,.F.);
#43656=ORIENTED_EDGE('',*,*,#30723,.T.);
#43657=ORIENTED_EDGE('',*,*,#30724,.T.);
#43658=ORIENTED_EDGE('',*,*,#30720,.F.);
#43659=ORIENTED_EDGE('',*,*,#30725,.F.);
#43660=ORIENTED_EDGE('',*,*,#30726,.T.);
#43661=ORIENTED_EDGE('',*,*,#30727,.T.);
#43662=ORIENTED_EDGE('',*,*,#30723,.F.);
#43663=ORIENTED_EDGE('',*,*,#30728,.F.);
#43664=ORIENTED_EDGE('',*,*,#30729,.T.);
#43665=ORIENTED_EDGE('',*,*,#30730,.T.);
#43666=ORIENTED_EDGE('',*,*,#30726,.F.);
#43667=ORIENTED_EDGE('',*,*,#30731,.F.);
#43668=ORIENTED_EDGE('',*,*,#30732,.T.);
#43669=ORIENTED_EDGE('',*,*,#30733,.T.);
#43670=ORIENTED_EDGE('',*,*,#30729,.F.);
#43671=ORIENTED_EDGE('',*,*,#30734,.F.);
#43672=ORIENTED_EDGE('',*,*,#30735,.T.);
#43673=ORIENTED_EDGE('',*,*,#30736,.T.);
#43674=ORIENTED_EDGE('',*,*,#30732,.F.);
#43675=ORIENTED_EDGE('',*,*,#30737,.F.);
#43676=ORIENTED_EDGE('',*,*,#30738,.T.);
#43677=ORIENTED_EDGE('',*,*,#30739,.T.);
#43678=ORIENTED_EDGE('',*,*,#30735,.F.);
#43679=ORIENTED_EDGE('',*,*,#30740,.F.);
#43680=ORIENTED_EDGE('',*,*,#30741,.T.);
#43681=ORIENTED_EDGE('',*,*,#30742,.T.);
#43682=ORIENTED_EDGE('',*,*,#30738,.F.);
#43683=ORIENTED_EDGE('',*,*,#30743,.F.);
#43684=ORIENTED_EDGE('',*,*,#30744,.T.);
#43685=ORIENTED_EDGE('',*,*,#30745,.T.);
#43686=ORIENTED_EDGE('',*,*,#30741,.F.);
#43687=ORIENTED_EDGE('',*,*,#30746,.F.);
#43688=ORIENTED_EDGE('',*,*,#30747,.T.);
#43689=ORIENTED_EDGE('',*,*,#30748,.T.);
#43690=ORIENTED_EDGE('',*,*,#30744,.F.);
#43691=ORIENTED_EDGE('',*,*,#30749,.F.);
#43692=ORIENTED_EDGE('',*,*,#30750,.T.);
#43693=ORIENTED_EDGE('',*,*,#30751,.T.);
#43694=ORIENTED_EDGE('',*,*,#30747,.F.);
#43695=ORIENTED_EDGE('',*,*,#30752,.F.);
#43696=ORIENTED_EDGE('',*,*,#30652,.T.);
#43697=ORIENTED_EDGE('',*,*,#30753,.T.);
#43698=ORIENTED_EDGE('',*,*,#30750,.F.);
#43699=ORIENTED_EDGE('',*,*,#30753,.F.);
#43700=ORIENTED_EDGE('',*,*,#30651,.F.);
#43701=ORIENTED_EDGE('',*,*,#30655,.F.);
#43702=ORIENTED_EDGE('',*,*,#30658,.F.);
#43703=ORIENTED_EDGE('',*,*,#30661,.F.);
#43704=ORIENTED_EDGE('',*,*,#30664,.F.);
#43705=ORIENTED_EDGE('',*,*,#30667,.F.);
#43706=ORIENTED_EDGE('',*,*,#30670,.F.);
#43707=ORIENTED_EDGE('',*,*,#30673,.F.);
#43708=ORIENTED_EDGE('',*,*,#30676,.F.);
#43709=ORIENTED_EDGE('',*,*,#30679,.F.);
#43710=ORIENTED_EDGE('',*,*,#30682,.F.);
#43711=ORIENTED_EDGE('',*,*,#30685,.F.);
#43712=ORIENTED_EDGE('',*,*,#30688,.F.);
#43713=ORIENTED_EDGE('',*,*,#30691,.F.);
#43714=ORIENTED_EDGE('',*,*,#30694,.F.);
#43715=ORIENTED_EDGE('',*,*,#30697,.F.);
#43716=ORIENTED_EDGE('',*,*,#30700,.F.);
#43717=ORIENTED_EDGE('',*,*,#30703,.F.);
#43718=ORIENTED_EDGE('',*,*,#30706,.F.);
#43719=ORIENTED_EDGE('',*,*,#30709,.F.);
#43720=ORIENTED_EDGE('',*,*,#30712,.F.);
#43721=ORIENTED_EDGE('',*,*,#30715,.F.);
#43722=ORIENTED_EDGE('',*,*,#30718,.F.);
#43723=ORIENTED_EDGE('',*,*,#30721,.F.);
#43724=ORIENTED_EDGE('',*,*,#30724,.F.);
#43725=ORIENTED_EDGE('',*,*,#30727,.F.);
#43726=ORIENTED_EDGE('',*,*,#30730,.F.);
#43727=ORIENTED_EDGE('',*,*,#30733,.F.);
#43728=ORIENTED_EDGE('',*,*,#30736,.F.);
#43729=ORIENTED_EDGE('',*,*,#30739,.F.);
#43730=ORIENTED_EDGE('',*,*,#30742,.F.);
#43731=ORIENTED_EDGE('',*,*,#30745,.F.);
#43732=ORIENTED_EDGE('',*,*,#30748,.F.);
#43733=ORIENTED_EDGE('',*,*,#30751,.F.);
#43734=ORIENTED_EDGE('',*,*,#30754,.F.);
#43735=ORIENTED_EDGE('',*,*,#30755,.T.);
#43736=ORIENTED_EDGE('',*,*,#30756,.T.);
#43737=ORIENTED_EDGE('',*,*,#30757,.F.);
#43738=ORIENTED_EDGE('',*,*,#30758,.F.);
#43739=ORIENTED_EDGE('',*,*,#30759,.T.);
#43740=ORIENTED_EDGE('',*,*,#30760,.T.);
#43741=ORIENTED_EDGE('',*,*,#30755,.F.);
#43742=ORIENTED_EDGE('',*,*,#30761,.F.);
#43743=ORIENTED_EDGE('',*,*,#30762,.T.);
#43744=ORIENTED_EDGE('',*,*,#30763,.T.);
#43745=ORIENTED_EDGE('',*,*,#30759,.F.);
#43746=ORIENTED_EDGE('',*,*,#30764,.F.);
#43747=ORIENTED_EDGE('',*,*,#30765,.T.);
#43748=ORIENTED_EDGE('',*,*,#30766,.T.);
#43749=ORIENTED_EDGE('',*,*,#30762,.F.);
#43750=ORIENTED_EDGE('',*,*,#30767,.F.);
#43751=ORIENTED_EDGE('',*,*,#30768,.T.);
#43752=ORIENTED_EDGE('',*,*,#30769,.T.);
#43753=ORIENTED_EDGE('',*,*,#30765,.F.);
#43754=ORIENTED_EDGE('',*,*,#30770,.F.);
#43755=ORIENTED_EDGE('',*,*,#30771,.T.);
#43756=ORIENTED_EDGE('',*,*,#30772,.T.);
#43757=ORIENTED_EDGE('',*,*,#30768,.F.);
#43758=ORIENTED_EDGE('',*,*,#30773,.F.);
#43759=ORIENTED_EDGE('',*,*,#30774,.T.);
#43760=ORIENTED_EDGE('',*,*,#30775,.T.);
#43761=ORIENTED_EDGE('',*,*,#30771,.F.);
#43762=ORIENTED_EDGE('',*,*,#30776,.F.);
#43763=ORIENTED_EDGE('',*,*,#30777,.T.);
#43764=ORIENTED_EDGE('',*,*,#30778,.T.);
#43765=ORIENTED_EDGE('',*,*,#30774,.F.);
#43766=ORIENTED_EDGE('',*,*,#30779,.F.);
#43767=ORIENTED_EDGE('',*,*,#30780,.T.);
#43768=ORIENTED_EDGE('',*,*,#30781,.T.);
#43769=ORIENTED_EDGE('',*,*,#30777,.F.);
#43770=ORIENTED_EDGE('',*,*,#30782,.F.);
#43771=ORIENTED_EDGE('',*,*,#30783,.T.);
#43772=ORIENTED_EDGE('',*,*,#30784,.T.);
#43773=ORIENTED_EDGE('',*,*,#30780,.F.);
#43774=ORIENTED_EDGE('',*,*,#30785,.F.);
#43775=ORIENTED_EDGE('',*,*,#30786,.T.);
#43776=ORIENTED_EDGE('',*,*,#30787,.T.);
#43777=ORIENTED_EDGE('',*,*,#30783,.F.);
#43778=ORIENTED_EDGE('',*,*,#30788,.F.);
#43779=ORIENTED_EDGE('',*,*,#30789,.T.);
#43780=ORIENTED_EDGE('',*,*,#30790,.T.);
#43781=ORIENTED_EDGE('',*,*,#30786,.F.);
#43782=ORIENTED_EDGE('',*,*,#30791,.F.);
#43783=ORIENTED_EDGE('',*,*,#30792,.T.);
#43784=ORIENTED_EDGE('',*,*,#30793,.T.);
#43785=ORIENTED_EDGE('',*,*,#30789,.F.);
#43786=ORIENTED_EDGE('',*,*,#30794,.F.);
#43787=ORIENTED_EDGE('',*,*,#30795,.T.);
#43788=ORIENTED_EDGE('',*,*,#30796,.T.);
#43789=ORIENTED_EDGE('',*,*,#30792,.F.);
#43790=ORIENTED_EDGE('',*,*,#30797,.F.);
#43791=ORIENTED_EDGE('',*,*,#30798,.T.);
#43792=ORIENTED_EDGE('',*,*,#30799,.T.);
#43793=ORIENTED_EDGE('',*,*,#30795,.F.);
#43794=ORIENTED_EDGE('',*,*,#30800,.F.);
#43795=ORIENTED_EDGE('',*,*,#30801,.T.);
#43796=ORIENTED_EDGE('',*,*,#30802,.T.);
#43797=ORIENTED_EDGE('',*,*,#30798,.F.);
#43798=ORIENTED_EDGE('',*,*,#30803,.F.);
#43799=ORIENTED_EDGE('',*,*,#30804,.T.);
#43800=ORIENTED_EDGE('',*,*,#30805,.T.);
#43801=ORIENTED_EDGE('',*,*,#30801,.F.);
#43802=ORIENTED_EDGE('',*,*,#30806,.F.);
#43803=ORIENTED_EDGE('',*,*,#30807,.T.);
#43804=ORIENTED_EDGE('',*,*,#30808,.T.);
#43805=ORIENTED_EDGE('',*,*,#30804,.F.);
#43806=ORIENTED_EDGE('',*,*,#30809,.F.);
#43807=ORIENTED_EDGE('',*,*,#30810,.T.);
#43808=ORIENTED_EDGE('',*,*,#30811,.T.);
#43809=ORIENTED_EDGE('',*,*,#30807,.F.);
#43810=ORIENTED_EDGE('',*,*,#30812,.F.);
#43811=ORIENTED_EDGE('',*,*,#30813,.T.);
#43812=ORIENTED_EDGE('',*,*,#30814,.T.);
#43813=ORIENTED_EDGE('',*,*,#30810,.F.);
#43814=ORIENTED_EDGE('',*,*,#30815,.F.);
#43815=ORIENTED_EDGE('',*,*,#30816,.T.);
#43816=ORIENTED_EDGE('',*,*,#30817,.T.);
#43817=ORIENTED_EDGE('',*,*,#30813,.F.);
#43818=ORIENTED_EDGE('',*,*,#30818,.F.);
#43819=ORIENTED_EDGE('',*,*,#30757,.T.);
#43820=ORIENTED_EDGE('',*,*,#30819,.T.);
#43821=ORIENTED_EDGE('',*,*,#30816,.F.);
#43822=ORIENTED_EDGE('',*,*,#30819,.F.);
#43823=ORIENTED_EDGE('',*,*,#30756,.F.);
#43824=ORIENTED_EDGE('',*,*,#30760,.F.);
#43825=ORIENTED_EDGE('',*,*,#30763,.F.);
#43826=ORIENTED_EDGE('',*,*,#30766,.F.);
#43827=ORIENTED_EDGE('',*,*,#30769,.F.);
#43828=ORIENTED_EDGE('',*,*,#30772,.F.);
#43829=ORIENTED_EDGE('',*,*,#30775,.F.);
#43830=ORIENTED_EDGE('',*,*,#30778,.F.);
#43831=ORIENTED_EDGE('',*,*,#30781,.F.);
#43832=ORIENTED_EDGE('',*,*,#30784,.F.);
#43833=ORIENTED_EDGE('',*,*,#30787,.F.);
#43834=ORIENTED_EDGE('',*,*,#30790,.F.);
#43835=ORIENTED_EDGE('',*,*,#30793,.F.);
#43836=ORIENTED_EDGE('',*,*,#30796,.F.);
#43837=ORIENTED_EDGE('',*,*,#30799,.F.);
#43838=ORIENTED_EDGE('',*,*,#30802,.F.);
#43839=ORIENTED_EDGE('',*,*,#30805,.F.);
#43840=ORIENTED_EDGE('',*,*,#30808,.F.);
#43841=ORIENTED_EDGE('',*,*,#30811,.F.);
#43842=ORIENTED_EDGE('',*,*,#30814,.F.);
#43843=ORIENTED_EDGE('',*,*,#30817,.F.);
#43844=ORIENTED_EDGE('',*,*,#30820,.F.);
#43845=ORIENTED_EDGE('',*,*,#30821,.T.);
#43846=ORIENTED_EDGE('',*,*,#30822,.T.);
#43847=ORIENTED_EDGE('',*,*,#30823,.F.);
#43848=ORIENTED_EDGE('',*,*,#30824,.F.);
#43849=ORIENTED_EDGE('',*,*,#30825,.T.);
#43850=ORIENTED_EDGE('',*,*,#30826,.T.);
#43851=ORIENTED_EDGE('',*,*,#30821,.F.);
#43852=ORIENTED_EDGE('',*,*,#30827,.F.);
#43853=ORIENTED_EDGE('',*,*,#30828,.T.);
#43854=ORIENTED_EDGE('',*,*,#30829,.T.);
#43855=ORIENTED_EDGE('',*,*,#30825,.F.);
#43856=ORIENTED_EDGE('',*,*,#30830,.F.);
#43857=ORIENTED_EDGE('',*,*,#30831,.T.);
#43858=ORIENTED_EDGE('',*,*,#30832,.T.);
#43859=ORIENTED_EDGE('',*,*,#30828,.F.);
#43860=ORIENTED_EDGE('',*,*,#30833,.F.);
#43861=ORIENTED_EDGE('',*,*,#30834,.T.);
#43862=ORIENTED_EDGE('',*,*,#30835,.T.);
#43863=ORIENTED_EDGE('',*,*,#30831,.F.);
#43864=ORIENTED_EDGE('',*,*,#30836,.F.);
#43865=ORIENTED_EDGE('',*,*,#30823,.T.);
#43866=ORIENTED_EDGE('',*,*,#30837,.T.);
#43867=ORIENTED_EDGE('',*,*,#30834,.F.);
#43868=ORIENTED_EDGE('',*,*,#30837,.F.);
#43869=ORIENTED_EDGE('',*,*,#30822,.F.);
#43870=ORIENTED_EDGE('',*,*,#30826,.F.);
#43871=ORIENTED_EDGE('',*,*,#30829,.F.);
#43872=ORIENTED_EDGE('',*,*,#30832,.F.);
#43873=ORIENTED_EDGE('',*,*,#30835,.F.);
#43874=ORIENTED_EDGE('',*,*,#30838,.F.);
#43875=ORIENTED_EDGE('',*,*,#30839,.T.);
#43876=ORIENTED_EDGE('',*,*,#30840,.T.);
#43877=ORIENTED_EDGE('',*,*,#30841,.F.);
#43878=ORIENTED_EDGE('',*,*,#30842,.F.);
#43879=ORIENTED_EDGE('',*,*,#30843,.T.);
#43880=ORIENTED_EDGE('',*,*,#30844,.T.);
#43881=ORIENTED_EDGE('',*,*,#30839,.F.);
#43882=ORIENTED_EDGE('',*,*,#30845,.F.);
#43883=ORIENTED_EDGE('',*,*,#30846,.T.);
#43884=ORIENTED_EDGE('',*,*,#30847,.T.);
#43885=ORIENTED_EDGE('',*,*,#30843,.F.);
#43886=ORIENTED_EDGE('',*,*,#30848,.F.);
#43887=ORIENTED_EDGE('',*,*,#30849,.T.);
#43888=ORIENTED_EDGE('',*,*,#30850,.T.);
#43889=ORIENTED_EDGE('',*,*,#30846,.F.);
#43890=ORIENTED_EDGE('',*,*,#30851,.F.);
#43891=ORIENTED_EDGE('',*,*,#30852,.T.);
#43892=ORIENTED_EDGE('',*,*,#30853,.T.);
#43893=ORIENTED_EDGE('',*,*,#30849,.F.);
#43894=ORIENTED_EDGE('',*,*,#30854,.F.);
#43895=ORIENTED_EDGE('',*,*,#30855,.T.);
#43896=ORIENTED_EDGE('',*,*,#30856,.T.);
#43897=ORIENTED_EDGE('',*,*,#30852,.F.);
#43898=ORIENTED_EDGE('',*,*,#30857,.F.);
#43899=ORIENTED_EDGE('',*,*,#30858,.T.);
#43900=ORIENTED_EDGE('',*,*,#30859,.T.);
#43901=ORIENTED_EDGE('',*,*,#30855,.F.);
#43902=ORIENTED_EDGE('',*,*,#30860,.F.);
#43903=ORIENTED_EDGE('',*,*,#30841,.T.);
#43904=ORIENTED_EDGE('',*,*,#30861,.T.);
#43905=ORIENTED_EDGE('',*,*,#30858,.F.);
#43906=ORIENTED_EDGE('',*,*,#30861,.F.);
#43907=ORIENTED_EDGE('',*,*,#30840,.F.);
#43908=ORIENTED_EDGE('',*,*,#30844,.F.);
#43909=ORIENTED_EDGE('',*,*,#30847,.F.);
#43910=ORIENTED_EDGE('',*,*,#30850,.F.);
#43911=ORIENTED_EDGE('',*,*,#30853,.F.);
#43912=ORIENTED_EDGE('',*,*,#30856,.F.);
#43913=ORIENTED_EDGE('',*,*,#30859,.F.);
#43914=ORIENTED_EDGE('',*,*,#30862,.F.);
#43915=ORIENTED_EDGE('',*,*,#30863,.T.);
#43916=ORIENTED_EDGE('',*,*,#30864,.T.);
#43917=ORIENTED_EDGE('',*,*,#30865,.F.);
#43918=ORIENTED_EDGE('',*,*,#30866,.F.);
#43919=ORIENTED_EDGE('',*,*,#30867,.T.);
#43920=ORIENTED_EDGE('',*,*,#30868,.T.);
#43921=ORIENTED_EDGE('',*,*,#30863,.F.);
#43922=ORIENTED_EDGE('',*,*,#30869,.F.);
#43923=ORIENTED_EDGE('',*,*,#30870,.T.);
#43924=ORIENTED_EDGE('',*,*,#30871,.T.);
#43925=ORIENTED_EDGE('',*,*,#30867,.F.);
#43926=ORIENTED_EDGE('',*,*,#30872,.F.);
#43927=ORIENTED_EDGE('',*,*,#30873,.T.);
#43928=ORIENTED_EDGE('',*,*,#30874,.T.);
#43929=ORIENTED_EDGE('',*,*,#30870,.F.);
#43930=ORIENTED_EDGE('',*,*,#30875,.F.);
#43931=ORIENTED_EDGE('',*,*,#30876,.T.);
#43932=ORIENTED_EDGE('',*,*,#30877,.T.);
#43933=ORIENTED_EDGE('',*,*,#30873,.F.);
#43934=ORIENTED_EDGE('',*,*,#30878,.F.);
#43935=ORIENTED_EDGE('',*,*,#30879,.T.);
#43936=ORIENTED_EDGE('',*,*,#30880,.T.);
#43937=ORIENTED_EDGE('',*,*,#30876,.F.);
#43938=ORIENTED_EDGE('',*,*,#30881,.F.);
#43939=ORIENTED_EDGE('',*,*,#30882,.T.);
#43940=ORIENTED_EDGE('',*,*,#30883,.T.);
#43941=ORIENTED_EDGE('',*,*,#30879,.F.);
#43942=ORIENTED_EDGE('',*,*,#30884,.F.);
#43943=ORIENTED_EDGE('',*,*,#30885,.T.);
#43944=ORIENTED_EDGE('',*,*,#30886,.T.);
#43945=ORIENTED_EDGE('',*,*,#30882,.F.);
#43946=ORIENTED_EDGE('',*,*,#30887,.F.);
#43947=ORIENTED_EDGE('',*,*,#30888,.T.);
#43948=ORIENTED_EDGE('',*,*,#30889,.T.);
#43949=ORIENTED_EDGE('',*,*,#30885,.F.);
#43950=ORIENTED_EDGE('',*,*,#30890,.F.);
#43951=ORIENTED_EDGE('',*,*,#30891,.T.);
#43952=ORIENTED_EDGE('',*,*,#30892,.T.);
#43953=ORIENTED_EDGE('',*,*,#30888,.F.);
#43954=ORIENTED_EDGE('',*,*,#30893,.F.);
#43955=ORIENTED_EDGE('',*,*,#30894,.T.);
#43956=ORIENTED_EDGE('',*,*,#30895,.T.);
#43957=ORIENTED_EDGE('',*,*,#30891,.F.);
#43958=ORIENTED_EDGE('',*,*,#30896,.F.);
#43959=ORIENTED_EDGE('',*,*,#30897,.T.);
#43960=ORIENTED_EDGE('',*,*,#30898,.T.);
#43961=ORIENTED_EDGE('',*,*,#30894,.F.);
#43962=ORIENTED_EDGE('',*,*,#30899,.F.);
#43963=ORIENTED_EDGE('',*,*,#30900,.T.);
#43964=ORIENTED_EDGE('',*,*,#30901,.T.);
#43965=ORIENTED_EDGE('',*,*,#30897,.F.);
#43966=ORIENTED_EDGE('',*,*,#30902,.F.);
#43967=ORIENTED_EDGE('',*,*,#30903,.T.);
#43968=ORIENTED_EDGE('',*,*,#30904,.T.);
#43969=ORIENTED_EDGE('',*,*,#30900,.F.);
#43970=ORIENTED_EDGE('',*,*,#30905,.F.);
#43971=ORIENTED_EDGE('',*,*,#30906,.T.);
#43972=ORIENTED_EDGE('',*,*,#30907,.T.);
#43973=ORIENTED_EDGE('',*,*,#30903,.F.);
#43974=ORIENTED_EDGE('',*,*,#30908,.F.);
#43975=ORIENTED_EDGE('',*,*,#30909,.T.);
#43976=ORIENTED_EDGE('',*,*,#30910,.T.);
#43977=ORIENTED_EDGE('',*,*,#30906,.F.);
#43978=ORIENTED_EDGE('',*,*,#30911,.F.);
#43979=ORIENTED_EDGE('',*,*,#30865,.T.);
#43980=ORIENTED_EDGE('',*,*,#30912,.T.);
#43981=ORIENTED_EDGE('',*,*,#30909,.F.);
#43982=ORIENTED_EDGE('',*,*,#30912,.F.);
#43983=ORIENTED_EDGE('',*,*,#30864,.F.);
#43984=ORIENTED_EDGE('',*,*,#30868,.F.);
#43985=ORIENTED_EDGE('',*,*,#30871,.F.);
#43986=ORIENTED_EDGE('',*,*,#30874,.F.);
#43987=ORIENTED_EDGE('',*,*,#30877,.F.);
#43988=ORIENTED_EDGE('',*,*,#30880,.F.);
#43989=ORIENTED_EDGE('',*,*,#30883,.F.);
#43990=ORIENTED_EDGE('',*,*,#30886,.F.);
#43991=ORIENTED_EDGE('',*,*,#30889,.F.);
#43992=ORIENTED_EDGE('',*,*,#30892,.F.);
#43993=ORIENTED_EDGE('',*,*,#30895,.F.);
#43994=ORIENTED_EDGE('',*,*,#30898,.F.);
#43995=ORIENTED_EDGE('',*,*,#30901,.F.);
#43996=ORIENTED_EDGE('',*,*,#30904,.F.);
#43997=ORIENTED_EDGE('',*,*,#30907,.F.);
#43998=ORIENTED_EDGE('',*,*,#30910,.F.);
#43999=ORIENTED_EDGE('',*,*,#30913,.F.);
#44000=ORIENTED_EDGE('',*,*,#30914,.T.);
#44001=ORIENTED_EDGE('',*,*,#30915,.T.);
#44002=ORIENTED_EDGE('',*,*,#30916,.F.);
#44003=ORIENTED_EDGE('',*,*,#30917,.F.);
#44004=ORIENTED_EDGE('',*,*,#30918,.T.);
#44005=ORIENTED_EDGE('',*,*,#30919,.T.);
#44006=ORIENTED_EDGE('',*,*,#30914,.F.);
#44007=ORIENTED_EDGE('',*,*,#30920,.F.);
#44008=ORIENTED_EDGE('',*,*,#30921,.T.);
#44009=ORIENTED_EDGE('',*,*,#30922,.T.);
#44010=ORIENTED_EDGE('',*,*,#30918,.F.);
#44011=ORIENTED_EDGE('',*,*,#30923,.F.);
#44012=ORIENTED_EDGE('',*,*,#30924,.T.);
#44013=ORIENTED_EDGE('',*,*,#30925,.T.);
#44014=ORIENTED_EDGE('',*,*,#30921,.F.);
#44015=ORIENTED_EDGE('',*,*,#30926,.F.);
#44016=ORIENTED_EDGE('',*,*,#30927,.T.);
#44017=ORIENTED_EDGE('',*,*,#30928,.T.);
#44018=ORIENTED_EDGE('',*,*,#30924,.F.);
#44019=ORIENTED_EDGE('',*,*,#30929,.F.);
#44020=ORIENTED_EDGE('',*,*,#30930,.T.);
#44021=ORIENTED_EDGE('',*,*,#30931,.T.);
#44022=ORIENTED_EDGE('',*,*,#30927,.F.);
#44023=ORIENTED_EDGE('',*,*,#30932,.F.);
#44024=ORIENTED_EDGE('',*,*,#30933,.T.);
#44025=ORIENTED_EDGE('',*,*,#30934,.T.);
#44026=ORIENTED_EDGE('',*,*,#30930,.F.);
#44027=ORIENTED_EDGE('',*,*,#30935,.F.);
#44028=ORIENTED_EDGE('',*,*,#30936,.T.);
#44029=ORIENTED_EDGE('',*,*,#30937,.T.);
#44030=ORIENTED_EDGE('',*,*,#30933,.F.);
#44031=ORIENTED_EDGE('',*,*,#30938,.F.);
#44032=ORIENTED_EDGE('',*,*,#30939,.T.);
#44033=ORIENTED_EDGE('',*,*,#30940,.T.);
#44034=ORIENTED_EDGE('',*,*,#30936,.F.);
#44035=ORIENTED_EDGE('',*,*,#30941,.F.);
#44036=ORIENTED_EDGE('',*,*,#30942,.T.);
#44037=ORIENTED_EDGE('',*,*,#30943,.T.);
#44038=ORIENTED_EDGE('',*,*,#30939,.F.);
#44039=ORIENTED_EDGE('',*,*,#30944,.F.);
#44040=ORIENTED_EDGE('',*,*,#30945,.T.);
#44041=ORIENTED_EDGE('',*,*,#30946,.T.);
#44042=ORIENTED_EDGE('',*,*,#30942,.F.);
#44043=ORIENTED_EDGE('',*,*,#30947,.F.);
#44044=ORIENTED_EDGE('',*,*,#30948,.T.);
#44045=ORIENTED_EDGE('',*,*,#30949,.T.);
#44046=ORIENTED_EDGE('',*,*,#30945,.F.);
#44047=ORIENTED_EDGE('',*,*,#30950,.F.);
#44048=ORIENTED_EDGE('',*,*,#30951,.T.);
#44049=ORIENTED_EDGE('',*,*,#30952,.T.);
#44050=ORIENTED_EDGE('',*,*,#30948,.F.);
#44051=ORIENTED_EDGE('',*,*,#30953,.F.);
#44052=ORIENTED_EDGE('',*,*,#30954,.T.);
#44053=ORIENTED_EDGE('',*,*,#30955,.T.);
#44054=ORIENTED_EDGE('',*,*,#30951,.F.);
#44055=ORIENTED_EDGE('',*,*,#30956,.F.);
#44056=ORIENTED_EDGE('',*,*,#30957,.T.);
#44057=ORIENTED_EDGE('',*,*,#30958,.T.);
#44058=ORIENTED_EDGE('',*,*,#30954,.F.);
#44059=ORIENTED_EDGE('',*,*,#30959,.F.);
#44060=ORIENTED_EDGE('',*,*,#30960,.T.);
#44061=ORIENTED_EDGE('',*,*,#30961,.T.);
#44062=ORIENTED_EDGE('',*,*,#30957,.F.);
#44063=ORIENTED_EDGE('',*,*,#30962,.F.);
#44064=ORIENTED_EDGE('',*,*,#30963,.T.);
#44065=ORIENTED_EDGE('',*,*,#30964,.T.);
#44066=ORIENTED_EDGE('',*,*,#30960,.F.);
#44067=ORIENTED_EDGE('',*,*,#30965,.F.);
#44068=ORIENTED_EDGE('',*,*,#30966,.T.);
#44069=ORIENTED_EDGE('',*,*,#30967,.T.);
#44070=ORIENTED_EDGE('',*,*,#30963,.F.);
#44071=ORIENTED_EDGE('',*,*,#30968,.F.);
#44072=ORIENTED_EDGE('',*,*,#30916,.T.);
#44073=ORIENTED_EDGE('',*,*,#30969,.T.);
#44074=ORIENTED_EDGE('',*,*,#30966,.F.);
#44075=ORIENTED_EDGE('',*,*,#30969,.F.);
#44076=ORIENTED_EDGE('',*,*,#30915,.F.);
#44077=ORIENTED_EDGE('',*,*,#30919,.F.);
#44078=ORIENTED_EDGE('',*,*,#30922,.F.);
#44079=ORIENTED_EDGE('',*,*,#30925,.F.);
#44080=ORIENTED_EDGE('',*,*,#30928,.F.);
#44081=ORIENTED_EDGE('',*,*,#30931,.F.);
#44082=ORIENTED_EDGE('',*,*,#30934,.F.);
#44083=ORIENTED_EDGE('',*,*,#30937,.F.);
#44084=ORIENTED_EDGE('',*,*,#30940,.F.);
#44085=ORIENTED_EDGE('',*,*,#30943,.F.);
#44086=ORIENTED_EDGE('',*,*,#30946,.F.);
#44087=ORIENTED_EDGE('',*,*,#30949,.F.);
#44088=ORIENTED_EDGE('',*,*,#30952,.F.);
#44089=ORIENTED_EDGE('',*,*,#30955,.F.);
#44090=ORIENTED_EDGE('',*,*,#30958,.F.);
#44091=ORIENTED_EDGE('',*,*,#30961,.F.);
#44092=ORIENTED_EDGE('',*,*,#30964,.F.);
#44093=ORIENTED_EDGE('',*,*,#30967,.F.);
#44094=ORIENTED_EDGE('',*,*,#30970,.F.);
#44095=ORIENTED_EDGE('',*,*,#30971,.T.);
#44096=ORIENTED_EDGE('',*,*,#30972,.T.);
#44097=ORIENTED_EDGE('',*,*,#30973,.F.);
#44098=ORIENTED_EDGE('',*,*,#30974,.F.);
#44099=ORIENTED_EDGE('',*,*,#30975,.T.);
#44100=ORIENTED_EDGE('',*,*,#30976,.T.);
#44101=ORIENTED_EDGE('',*,*,#30971,.F.);
#44102=ORIENTED_EDGE('',*,*,#30977,.F.);
#44103=ORIENTED_EDGE('',*,*,#30978,.T.);
#44104=ORIENTED_EDGE('',*,*,#30979,.T.);
#44105=ORIENTED_EDGE('',*,*,#30975,.F.);
#44106=ORIENTED_EDGE('',*,*,#30980,.F.);
#44107=ORIENTED_EDGE('',*,*,#30981,.T.);
#44108=ORIENTED_EDGE('',*,*,#30982,.T.);
#44109=ORIENTED_EDGE('',*,*,#30978,.F.);
#44110=ORIENTED_EDGE('',*,*,#30983,.F.);
#44111=ORIENTED_EDGE('',*,*,#30984,.T.);
#44112=ORIENTED_EDGE('',*,*,#30985,.T.);
#44113=ORIENTED_EDGE('',*,*,#30981,.F.);
#44114=ORIENTED_EDGE('',*,*,#30986,.F.);
#44115=ORIENTED_EDGE('',*,*,#30987,.T.);
#44116=ORIENTED_EDGE('',*,*,#30988,.T.);
#44117=ORIENTED_EDGE('',*,*,#30984,.F.);
#44118=ORIENTED_EDGE('',*,*,#30989,.F.);
#44119=ORIENTED_EDGE('',*,*,#30990,.T.);
#44120=ORIENTED_EDGE('',*,*,#30991,.T.);
#44121=ORIENTED_EDGE('',*,*,#30987,.F.);
#44122=ORIENTED_EDGE('',*,*,#30992,.F.);
#44123=ORIENTED_EDGE('',*,*,#30973,.T.);
#44124=ORIENTED_EDGE('',*,*,#30993,.T.);
#44125=ORIENTED_EDGE('',*,*,#30990,.F.);
#44126=ORIENTED_EDGE('',*,*,#30993,.F.);
#44127=ORIENTED_EDGE('',*,*,#30972,.F.);
#44128=ORIENTED_EDGE('',*,*,#30976,.F.);
#44129=ORIENTED_EDGE('',*,*,#30979,.F.);
#44130=ORIENTED_EDGE('',*,*,#30982,.F.);
#44131=ORIENTED_EDGE('',*,*,#30985,.F.);
#44132=ORIENTED_EDGE('',*,*,#30988,.F.);
#44133=ORIENTED_EDGE('',*,*,#30991,.F.);
#44134=ORIENTED_EDGE('',*,*,#30994,.F.);
#44135=ORIENTED_EDGE('',*,*,#30995,.T.);
#44136=ORIENTED_EDGE('',*,*,#30996,.T.);
#44137=ORIENTED_EDGE('',*,*,#30997,.F.);
#44138=ORIENTED_EDGE('',*,*,#30998,.F.);
#44139=ORIENTED_EDGE('',*,*,#30999,.T.);
#44140=ORIENTED_EDGE('',*,*,#31000,.T.);
#44141=ORIENTED_EDGE('',*,*,#30995,.F.);
#44142=ORIENTED_EDGE('',*,*,#31001,.F.);
#44143=ORIENTED_EDGE('',*,*,#31002,.T.);
#44144=ORIENTED_EDGE('',*,*,#31003,.T.);
#44145=ORIENTED_EDGE('',*,*,#30999,.F.);
#44146=ORIENTED_EDGE('',*,*,#31004,.F.);
#44147=ORIENTED_EDGE('',*,*,#31005,.T.);
#44148=ORIENTED_EDGE('',*,*,#31006,.T.);
#44149=ORIENTED_EDGE('',*,*,#31002,.F.);
#44150=ORIENTED_EDGE('',*,*,#31007,.F.);
#44151=ORIENTED_EDGE('',*,*,#31008,.T.);
#44152=ORIENTED_EDGE('',*,*,#31009,.T.);
#44153=ORIENTED_EDGE('',*,*,#31005,.F.);
#44154=ORIENTED_EDGE('',*,*,#31010,.F.);
#44155=ORIENTED_EDGE('',*,*,#31011,.T.);
#44156=ORIENTED_EDGE('',*,*,#31012,.T.);
#44157=ORIENTED_EDGE('',*,*,#31008,.F.);
#44158=ORIENTED_EDGE('',*,*,#31013,.F.);
#44159=ORIENTED_EDGE('',*,*,#31014,.T.);
#44160=ORIENTED_EDGE('',*,*,#31015,.T.);
#44161=ORIENTED_EDGE('',*,*,#31011,.F.);
#44162=ORIENTED_EDGE('',*,*,#31016,.F.);
#44163=ORIENTED_EDGE('',*,*,#31017,.T.);
#44164=ORIENTED_EDGE('',*,*,#31018,.T.);
#44165=ORIENTED_EDGE('',*,*,#31014,.F.);
#44166=ORIENTED_EDGE('',*,*,#31019,.F.);
#44167=ORIENTED_EDGE('',*,*,#30997,.T.);
#44168=ORIENTED_EDGE('',*,*,#31020,.T.);
#44169=ORIENTED_EDGE('',*,*,#31017,.F.);
#44170=ORIENTED_EDGE('',*,*,#31020,.F.);
#44171=ORIENTED_EDGE('',*,*,#30996,.F.);
#44172=ORIENTED_EDGE('',*,*,#31000,.F.);
#44173=ORIENTED_EDGE('',*,*,#31003,.F.);
#44174=ORIENTED_EDGE('',*,*,#31006,.F.);
#44175=ORIENTED_EDGE('',*,*,#31009,.F.);
#44176=ORIENTED_EDGE('',*,*,#31012,.F.);
#44177=ORIENTED_EDGE('',*,*,#31015,.F.);
#44178=ORIENTED_EDGE('',*,*,#31018,.F.);
#44179=ORIENTED_EDGE('',*,*,#31021,.F.);
#44180=ORIENTED_EDGE('',*,*,#31022,.T.);
#44181=ORIENTED_EDGE('',*,*,#31023,.T.);
#44182=ORIENTED_EDGE('',*,*,#31024,.F.);
#44183=ORIENTED_EDGE('',*,*,#31025,.F.);
#44184=ORIENTED_EDGE('',*,*,#31026,.T.);
#44185=ORIENTED_EDGE('',*,*,#31027,.T.);
#44186=ORIENTED_EDGE('',*,*,#31022,.F.);
#44187=ORIENTED_EDGE('',*,*,#31028,.F.);
#44188=ORIENTED_EDGE('',*,*,#31029,.T.);
#44189=ORIENTED_EDGE('',*,*,#31030,.T.);
#44190=ORIENTED_EDGE('',*,*,#31026,.F.);
#44191=ORIENTED_EDGE('',*,*,#31031,.F.);
#44192=ORIENTED_EDGE('',*,*,#31032,.T.);
#44193=ORIENTED_EDGE('',*,*,#31033,.T.);
#44194=ORIENTED_EDGE('',*,*,#31029,.F.);
#44195=ORIENTED_EDGE('',*,*,#31034,.F.);
#44196=ORIENTED_EDGE('',*,*,#31035,.T.);
#44197=ORIENTED_EDGE('',*,*,#31036,.T.);
#44198=ORIENTED_EDGE('',*,*,#31032,.F.);
#44199=ORIENTED_EDGE('',*,*,#31037,.F.);
#44200=ORIENTED_EDGE('',*,*,#31038,.T.);
#44201=ORIENTED_EDGE('',*,*,#31039,.T.);
#44202=ORIENTED_EDGE('',*,*,#31035,.F.);
#44203=ORIENTED_EDGE('',*,*,#31040,.F.);
#44204=ORIENTED_EDGE('',*,*,#31041,.T.);
#44205=ORIENTED_EDGE('',*,*,#31042,.T.);
#44206=ORIENTED_EDGE('',*,*,#31038,.F.);
#44207=ORIENTED_EDGE('',*,*,#31043,.F.);
#44208=ORIENTED_EDGE('',*,*,#31044,.T.);
#44209=ORIENTED_EDGE('',*,*,#31045,.T.);
#44210=ORIENTED_EDGE('',*,*,#31041,.F.);
#44211=ORIENTED_EDGE('',*,*,#31046,.F.);
#44212=ORIENTED_EDGE('',*,*,#31047,.T.);
#44213=ORIENTED_EDGE('',*,*,#31048,.T.);
#44214=ORIENTED_EDGE('',*,*,#31044,.F.);
#44215=ORIENTED_EDGE('',*,*,#31049,.F.);
#44216=ORIENTED_EDGE('',*,*,#31050,.T.);
#44217=ORIENTED_EDGE('',*,*,#31051,.T.);
#44218=ORIENTED_EDGE('',*,*,#31047,.F.);
#44219=ORIENTED_EDGE('',*,*,#31052,.F.);
#44220=ORIENTED_EDGE('',*,*,#31053,.T.);
#44221=ORIENTED_EDGE('',*,*,#31054,.T.);
#44222=ORIENTED_EDGE('',*,*,#31050,.F.);
#44223=ORIENTED_EDGE('',*,*,#31055,.F.);
#44224=ORIENTED_EDGE('',*,*,#31024,.T.);
#44225=ORIENTED_EDGE('',*,*,#31056,.T.);
#44226=ORIENTED_EDGE('',*,*,#31053,.F.);
#44227=ORIENTED_EDGE('',*,*,#31056,.F.);
#44228=ORIENTED_EDGE('',*,*,#31023,.F.);
#44229=ORIENTED_EDGE('',*,*,#31027,.F.);
#44230=ORIENTED_EDGE('',*,*,#31030,.F.);
#44231=ORIENTED_EDGE('',*,*,#31033,.F.);
#44232=ORIENTED_EDGE('',*,*,#31036,.F.);
#44233=ORIENTED_EDGE('',*,*,#31039,.F.);
#44234=ORIENTED_EDGE('',*,*,#31042,.F.);
#44235=ORIENTED_EDGE('',*,*,#31045,.F.);
#44236=ORIENTED_EDGE('',*,*,#31048,.F.);
#44237=ORIENTED_EDGE('',*,*,#31051,.F.);
#44238=ORIENTED_EDGE('',*,*,#31054,.F.);
#44239=ORIENTED_EDGE('',*,*,#31057,.F.);
#44240=ORIENTED_EDGE('',*,*,#31058,.T.);
#44241=ORIENTED_EDGE('',*,*,#31059,.T.);
#44242=ORIENTED_EDGE('',*,*,#31060,.F.);
#44243=ORIENTED_EDGE('',*,*,#31061,.F.);
#44244=ORIENTED_EDGE('',*,*,#31062,.T.);
#44245=ORIENTED_EDGE('',*,*,#31063,.T.);
#44246=ORIENTED_EDGE('',*,*,#31058,.F.);
#44247=ORIENTED_EDGE('',*,*,#31064,.F.);
#44248=ORIENTED_EDGE('',*,*,#31065,.T.);
#44249=ORIENTED_EDGE('',*,*,#31066,.T.);
#44250=ORIENTED_EDGE('',*,*,#31062,.F.);
#44251=ORIENTED_EDGE('',*,*,#31067,.F.);
#44252=ORIENTED_EDGE('',*,*,#31068,.T.);
#44253=ORIENTED_EDGE('',*,*,#31069,.T.);
#44254=ORIENTED_EDGE('',*,*,#31065,.F.);
#44255=ORIENTED_EDGE('',*,*,#31070,.F.);
#44256=ORIENTED_EDGE('',*,*,#31071,.T.);
#44257=ORIENTED_EDGE('',*,*,#31072,.T.);
#44258=ORIENTED_EDGE('',*,*,#31068,.F.);
#44259=ORIENTED_EDGE('',*,*,#31073,.F.);
#44260=ORIENTED_EDGE('',*,*,#31074,.T.);
#44261=ORIENTED_EDGE('',*,*,#31075,.T.);
#44262=ORIENTED_EDGE('',*,*,#31071,.F.);
#44263=ORIENTED_EDGE('',*,*,#31076,.F.);
#44264=ORIENTED_EDGE('',*,*,#31077,.T.);
#44265=ORIENTED_EDGE('',*,*,#31078,.T.);
#44266=ORIENTED_EDGE('',*,*,#31074,.F.);
#44267=ORIENTED_EDGE('',*,*,#31079,.F.);
#44268=ORIENTED_EDGE('',*,*,#31080,.T.);
#44269=ORIENTED_EDGE('',*,*,#31081,.T.);
#44270=ORIENTED_EDGE('',*,*,#31077,.F.);
#44271=ORIENTED_EDGE('',*,*,#31082,.F.);
#44272=ORIENTED_EDGE('',*,*,#31060,.T.);
#44273=ORIENTED_EDGE('',*,*,#31083,.T.);
#44274=ORIENTED_EDGE('',*,*,#31080,.F.);
#44275=ORIENTED_EDGE('',*,*,#31083,.F.);
#44276=ORIENTED_EDGE('',*,*,#31059,.F.);
#44277=ORIENTED_EDGE('',*,*,#31063,.F.);
#44278=ORIENTED_EDGE('',*,*,#31066,.F.);
#44279=ORIENTED_EDGE('',*,*,#31069,.F.);
#44280=ORIENTED_EDGE('',*,*,#31072,.F.);
#44281=ORIENTED_EDGE('',*,*,#31075,.F.);
#44282=ORIENTED_EDGE('',*,*,#31078,.F.);
#44283=ORIENTED_EDGE('',*,*,#31081,.F.);
#44284=ORIENTED_EDGE('',*,*,#31084,.F.);
#44285=ORIENTED_EDGE('',*,*,#31085,.T.);
#44286=ORIENTED_EDGE('',*,*,#31086,.T.);
#44287=ORIENTED_EDGE('',*,*,#31087,.F.);
#44288=ORIENTED_EDGE('',*,*,#31088,.F.);
#44289=ORIENTED_EDGE('',*,*,#31089,.T.);
#44290=ORIENTED_EDGE('',*,*,#31090,.T.);
#44291=ORIENTED_EDGE('',*,*,#31085,.F.);
#44292=ORIENTED_EDGE('',*,*,#31091,.F.);
#44293=ORIENTED_EDGE('',*,*,#31092,.T.);
#44294=ORIENTED_EDGE('',*,*,#31093,.T.);
#44295=ORIENTED_EDGE('',*,*,#31089,.F.);
#44296=ORIENTED_EDGE('',*,*,#31094,.F.);
#44297=ORIENTED_EDGE('',*,*,#31087,.T.);
#44298=ORIENTED_EDGE('',*,*,#31095,.T.);
#44299=ORIENTED_EDGE('',*,*,#31092,.F.);
#44300=ORIENTED_EDGE('',*,*,#31095,.F.);
#44301=ORIENTED_EDGE('',*,*,#31086,.F.);
#44302=ORIENTED_EDGE('',*,*,#31090,.F.);
#44303=ORIENTED_EDGE('',*,*,#31093,.F.);
#44304=ORIENTED_EDGE('',*,*,#31096,.F.);
#44305=ORIENTED_EDGE('',*,*,#31097,.T.);
#44306=ORIENTED_EDGE('',*,*,#31098,.T.);
#44307=ORIENTED_EDGE('',*,*,#31099,.F.);
#44308=ORIENTED_EDGE('',*,*,#31100,.F.);
#44309=ORIENTED_EDGE('',*,*,#31101,.T.);
#44310=ORIENTED_EDGE('',*,*,#31102,.T.);
#44311=ORIENTED_EDGE('',*,*,#31097,.F.);
#44312=ORIENTED_EDGE('',*,*,#31103,.F.);
#44313=ORIENTED_EDGE('',*,*,#31104,.T.);
#44314=ORIENTED_EDGE('',*,*,#31105,.T.);
#44315=ORIENTED_EDGE('',*,*,#31101,.F.);
#44316=ORIENTED_EDGE('',*,*,#31106,.F.);
#44317=ORIENTED_EDGE('',*,*,#31107,.T.);
#44318=ORIENTED_EDGE('',*,*,#31108,.T.);
#44319=ORIENTED_EDGE('',*,*,#31104,.F.);
#44320=ORIENTED_EDGE('',*,*,#31109,.F.);
#44321=ORIENTED_EDGE('',*,*,#31110,.T.);
#44322=ORIENTED_EDGE('',*,*,#31111,.T.);
#44323=ORIENTED_EDGE('',*,*,#31107,.F.);
#44324=ORIENTED_EDGE('',*,*,#31112,.F.);
#44325=ORIENTED_EDGE('',*,*,#31113,.T.);
#44326=ORIENTED_EDGE('',*,*,#31114,.T.);
#44327=ORIENTED_EDGE('',*,*,#31110,.F.);
#44328=ORIENTED_EDGE('',*,*,#31115,.F.);
#44329=ORIENTED_EDGE('',*,*,#31116,.T.);
#44330=ORIENTED_EDGE('',*,*,#31117,.T.);
#44331=ORIENTED_EDGE('',*,*,#31113,.F.);
#44332=ORIENTED_EDGE('',*,*,#31118,.F.);
#44333=ORIENTED_EDGE('',*,*,#31119,.T.);
#44334=ORIENTED_EDGE('',*,*,#31120,.T.);
#44335=ORIENTED_EDGE('',*,*,#31116,.F.);
#44336=ORIENTED_EDGE('',*,*,#31121,.F.);
#44337=ORIENTED_EDGE('',*,*,#31122,.T.);
#44338=ORIENTED_EDGE('',*,*,#31123,.T.);
#44339=ORIENTED_EDGE('',*,*,#31119,.F.);
#44340=ORIENTED_EDGE('',*,*,#31124,.F.);
#44341=ORIENTED_EDGE('',*,*,#31125,.T.);
#44342=ORIENTED_EDGE('',*,*,#31126,.T.);
#44343=ORIENTED_EDGE('',*,*,#31122,.F.);
#44344=ORIENTED_EDGE('',*,*,#31127,.F.);
#44345=ORIENTED_EDGE('',*,*,#31128,.T.);
#44346=ORIENTED_EDGE('',*,*,#31129,.T.);
#44347=ORIENTED_EDGE('',*,*,#31125,.F.);
#44348=ORIENTED_EDGE('',*,*,#31130,.F.);
#44349=ORIENTED_EDGE('',*,*,#31131,.T.);
#44350=ORIENTED_EDGE('',*,*,#31132,.T.);
#44351=ORIENTED_EDGE('',*,*,#31128,.F.);
#44352=ORIENTED_EDGE('',*,*,#31133,.F.);
#44353=ORIENTED_EDGE('',*,*,#31134,.T.);
#44354=ORIENTED_EDGE('',*,*,#31135,.T.);
#44355=ORIENTED_EDGE('',*,*,#31131,.F.);
#44356=ORIENTED_EDGE('',*,*,#31136,.F.);
#44357=ORIENTED_EDGE('',*,*,#31137,.T.);
#44358=ORIENTED_EDGE('',*,*,#31138,.T.);
#44359=ORIENTED_EDGE('',*,*,#31134,.F.);
#44360=ORIENTED_EDGE('',*,*,#31139,.F.);
#44361=ORIENTED_EDGE('',*,*,#31140,.T.);
#44362=ORIENTED_EDGE('',*,*,#31141,.T.);
#44363=ORIENTED_EDGE('',*,*,#31137,.F.);
#44364=ORIENTED_EDGE('',*,*,#31142,.F.);
#44365=ORIENTED_EDGE('',*,*,#31143,.T.);
#44366=ORIENTED_EDGE('',*,*,#31144,.T.);
#44367=ORIENTED_EDGE('',*,*,#31140,.F.);
#44368=ORIENTED_EDGE('',*,*,#31145,.F.);
#44369=ORIENTED_EDGE('',*,*,#31146,.T.);
#44370=ORIENTED_EDGE('',*,*,#31147,.T.);
#44371=ORIENTED_EDGE('',*,*,#31143,.F.);
#44372=ORIENTED_EDGE('',*,*,#31148,.F.);
#44373=ORIENTED_EDGE('',*,*,#31149,.T.);
#44374=ORIENTED_EDGE('',*,*,#31150,.T.);
#44375=ORIENTED_EDGE('',*,*,#31146,.F.);
#44376=ORIENTED_EDGE('',*,*,#31151,.F.);
#44377=ORIENTED_EDGE('',*,*,#31152,.T.);
#44378=ORIENTED_EDGE('',*,*,#31153,.T.);
#44379=ORIENTED_EDGE('',*,*,#31149,.F.);
#44380=ORIENTED_EDGE('',*,*,#31154,.F.);
#44381=ORIENTED_EDGE('',*,*,#31155,.T.);
#44382=ORIENTED_EDGE('',*,*,#31156,.T.);
#44383=ORIENTED_EDGE('',*,*,#31152,.F.);
#44384=ORIENTED_EDGE('',*,*,#31157,.F.);
#44385=ORIENTED_EDGE('',*,*,#31158,.T.);
#44386=ORIENTED_EDGE('',*,*,#31159,.T.);
#44387=ORIENTED_EDGE('',*,*,#31155,.F.);
#44388=ORIENTED_EDGE('',*,*,#31160,.F.);
#44389=ORIENTED_EDGE('',*,*,#31099,.T.);
#44390=ORIENTED_EDGE('',*,*,#31161,.T.);
#44391=ORIENTED_EDGE('',*,*,#31158,.F.);
#44392=ORIENTED_EDGE('',*,*,#31161,.F.);
#44393=ORIENTED_EDGE('',*,*,#31098,.F.);
#44394=ORIENTED_EDGE('',*,*,#31102,.F.);
#44395=ORIENTED_EDGE('',*,*,#31105,.F.);
#44396=ORIENTED_EDGE('',*,*,#31108,.F.);
#44397=ORIENTED_EDGE('',*,*,#31111,.F.);
#44398=ORIENTED_EDGE('',*,*,#31114,.F.);
#44399=ORIENTED_EDGE('',*,*,#31117,.F.);
#44400=ORIENTED_EDGE('',*,*,#31120,.F.);
#44401=ORIENTED_EDGE('',*,*,#31123,.F.);
#44402=ORIENTED_EDGE('',*,*,#31126,.F.);
#44403=ORIENTED_EDGE('',*,*,#31129,.F.);
#44404=ORIENTED_EDGE('',*,*,#31132,.F.);
#44405=ORIENTED_EDGE('',*,*,#31135,.F.);
#44406=ORIENTED_EDGE('',*,*,#31138,.F.);
#44407=ORIENTED_EDGE('',*,*,#31141,.F.);
#44408=ORIENTED_EDGE('',*,*,#31144,.F.);
#44409=ORIENTED_EDGE('',*,*,#31147,.F.);
#44410=ORIENTED_EDGE('',*,*,#31150,.F.);
#44411=ORIENTED_EDGE('',*,*,#31153,.F.);
#44412=ORIENTED_EDGE('',*,*,#31156,.F.);
#44413=ORIENTED_EDGE('',*,*,#31159,.F.);
#44414=ORIENTED_EDGE('',*,*,#31162,.F.);
#44415=ORIENTED_EDGE('',*,*,#31163,.T.);
#44416=ORIENTED_EDGE('',*,*,#31164,.T.);
#44417=ORIENTED_EDGE('',*,*,#31165,.F.);
#44418=ORIENTED_EDGE('',*,*,#31166,.F.);
#44419=ORIENTED_EDGE('',*,*,#31167,.T.);
#44420=ORIENTED_EDGE('',*,*,#31168,.T.);
#44421=ORIENTED_EDGE('',*,*,#31163,.F.);
#44422=ORIENTED_EDGE('',*,*,#31169,.F.);
#44423=ORIENTED_EDGE('',*,*,#31170,.T.);
#44424=ORIENTED_EDGE('',*,*,#31171,.T.);
#44425=ORIENTED_EDGE('',*,*,#31167,.F.);
#44426=ORIENTED_EDGE('',*,*,#31172,.F.);
#44427=ORIENTED_EDGE('',*,*,#31173,.T.);
#44428=ORIENTED_EDGE('',*,*,#31174,.T.);
#44429=ORIENTED_EDGE('',*,*,#31170,.F.);
#44430=ORIENTED_EDGE('',*,*,#31175,.F.);
#44431=ORIENTED_EDGE('',*,*,#31176,.T.);
#44432=ORIENTED_EDGE('',*,*,#31177,.T.);
#44433=ORIENTED_EDGE('',*,*,#31173,.F.);
#44434=ORIENTED_EDGE('',*,*,#31178,.F.);
#44435=ORIENTED_EDGE('',*,*,#31179,.T.);
#44436=ORIENTED_EDGE('',*,*,#31180,.T.);
#44437=ORIENTED_EDGE('',*,*,#31176,.F.);
#44438=ORIENTED_EDGE('',*,*,#31181,.F.);
#44439=ORIENTED_EDGE('',*,*,#31182,.T.);
#44440=ORIENTED_EDGE('',*,*,#31183,.T.);
#44441=ORIENTED_EDGE('',*,*,#31179,.F.);
#44442=ORIENTED_EDGE('',*,*,#31184,.F.);
#44443=ORIENTED_EDGE('',*,*,#31185,.T.);
#44444=ORIENTED_EDGE('',*,*,#31186,.T.);
#44445=ORIENTED_EDGE('',*,*,#31182,.F.);
#44446=ORIENTED_EDGE('',*,*,#31187,.F.);
#44447=ORIENTED_EDGE('',*,*,#31188,.T.);
#44448=ORIENTED_EDGE('',*,*,#31189,.T.);
#44449=ORIENTED_EDGE('',*,*,#31185,.F.);
#44450=ORIENTED_EDGE('',*,*,#31190,.F.);
#44451=ORIENTED_EDGE('',*,*,#31191,.T.);
#44452=ORIENTED_EDGE('',*,*,#31192,.T.);
#44453=ORIENTED_EDGE('',*,*,#31188,.F.);
#44454=ORIENTED_EDGE('',*,*,#31193,.F.);
#44455=ORIENTED_EDGE('',*,*,#31165,.T.);
#44456=ORIENTED_EDGE('',*,*,#31194,.T.);
#44457=ORIENTED_EDGE('',*,*,#31191,.F.);
#44458=ORIENTED_EDGE('',*,*,#31194,.F.);
#44459=ORIENTED_EDGE('',*,*,#31164,.F.);
#44460=ORIENTED_EDGE('',*,*,#31168,.F.);
#44461=ORIENTED_EDGE('',*,*,#31171,.F.);
#44462=ORIENTED_EDGE('',*,*,#31174,.F.);
#44463=ORIENTED_EDGE('',*,*,#31177,.F.);
#44464=ORIENTED_EDGE('',*,*,#31180,.F.);
#44465=ORIENTED_EDGE('',*,*,#31183,.F.);
#44466=ORIENTED_EDGE('',*,*,#31186,.F.);
#44467=ORIENTED_EDGE('',*,*,#31189,.F.);
#44468=ORIENTED_EDGE('',*,*,#31192,.F.);
#44469=ORIENTED_EDGE('',*,*,#31195,.F.);
#44470=ORIENTED_EDGE('',*,*,#31196,.T.);
#44471=ORIENTED_EDGE('',*,*,#31197,.T.);
#44472=ORIENTED_EDGE('',*,*,#31198,.F.);
#44473=ORIENTED_EDGE('',*,*,#31199,.F.);
#44474=ORIENTED_EDGE('',*,*,#31200,.T.);
#44475=ORIENTED_EDGE('',*,*,#31201,.T.);
#44476=ORIENTED_EDGE('',*,*,#31196,.F.);
#44477=ORIENTED_EDGE('',*,*,#31202,.F.);
#44478=ORIENTED_EDGE('',*,*,#31203,.T.);
#44479=ORIENTED_EDGE('',*,*,#31204,.T.);
#44480=ORIENTED_EDGE('',*,*,#31200,.F.);
#44481=ORIENTED_EDGE('',*,*,#31205,.F.);
#44482=ORIENTED_EDGE('',*,*,#31206,.T.);
#44483=ORIENTED_EDGE('',*,*,#31207,.T.);
#44484=ORIENTED_EDGE('',*,*,#31203,.F.);
#44485=ORIENTED_EDGE('',*,*,#31208,.F.);
#44486=ORIENTED_EDGE('',*,*,#31209,.T.);
#44487=ORIENTED_EDGE('',*,*,#31210,.T.);
#44488=ORIENTED_EDGE('',*,*,#31206,.F.);
#44489=ORIENTED_EDGE('',*,*,#31211,.F.);
#44490=ORIENTED_EDGE('',*,*,#31212,.T.);
#44491=ORIENTED_EDGE('',*,*,#31213,.T.);
#44492=ORIENTED_EDGE('',*,*,#31209,.F.);
#44493=ORIENTED_EDGE('',*,*,#31214,.F.);
#44494=ORIENTED_EDGE('',*,*,#31215,.T.);
#44495=ORIENTED_EDGE('',*,*,#31216,.T.);
#44496=ORIENTED_EDGE('',*,*,#31212,.F.);
#44497=ORIENTED_EDGE('',*,*,#31217,.F.);
#44498=ORIENTED_EDGE('',*,*,#31218,.T.);
#44499=ORIENTED_EDGE('',*,*,#31219,.T.);
#44500=ORIENTED_EDGE('',*,*,#31215,.F.);
#44501=ORIENTED_EDGE('',*,*,#31220,.F.);
#44502=ORIENTED_EDGE('',*,*,#31221,.T.);
#44503=ORIENTED_EDGE('',*,*,#31222,.T.);
#44504=ORIENTED_EDGE('',*,*,#31218,.F.);
#44505=ORIENTED_EDGE('',*,*,#31223,.F.);
#44506=ORIENTED_EDGE('',*,*,#31224,.T.);
#44507=ORIENTED_EDGE('',*,*,#31225,.T.);
#44508=ORIENTED_EDGE('',*,*,#31221,.F.);
#44509=ORIENTED_EDGE('',*,*,#31226,.F.);
#44510=ORIENTED_EDGE('',*,*,#31227,.T.);
#44511=ORIENTED_EDGE('',*,*,#31228,.T.);
#44512=ORIENTED_EDGE('',*,*,#31224,.F.);
#44513=ORIENTED_EDGE('',*,*,#31229,.F.);
#44514=ORIENTED_EDGE('',*,*,#31230,.T.);
#44515=ORIENTED_EDGE('',*,*,#31231,.T.);
#44516=ORIENTED_EDGE('',*,*,#31227,.F.);
#44517=ORIENTED_EDGE('',*,*,#31232,.F.);
#44518=ORIENTED_EDGE('',*,*,#31233,.T.);
#44519=ORIENTED_EDGE('',*,*,#31234,.T.);
#44520=ORIENTED_EDGE('',*,*,#31230,.F.);
#44521=ORIENTED_EDGE('',*,*,#31235,.F.);
#44522=ORIENTED_EDGE('',*,*,#31236,.T.);
#44523=ORIENTED_EDGE('',*,*,#31237,.T.);
#44524=ORIENTED_EDGE('',*,*,#31233,.F.);
#44525=ORIENTED_EDGE('',*,*,#31238,.F.);
#44526=ORIENTED_EDGE('',*,*,#31198,.T.);
#44527=ORIENTED_EDGE('',*,*,#31239,.T.);
#44528=ORIENTED_EDGE('',*,*,#31236,.F.);
#44529=ORIENTED_EDGE('',*,*,#31239,.F.);
#44530=ORIENTED_EDGE('',*,*,#31197,.F.);
#44531=ORIENTED_EDGE('',*,*,#31201,.F.);
#44532=ORIENTED_EDGE('',*,*,#31204,.F.);
#44533=ORIENTED_EDGE('',*,*,#31207,.F.);
#44534=ORIENTED_EDGE('',*,*,#31210,.F.);
#44535=ORIENTED_EDGE('',*,*,#31213,.F.);
#44536=ORIENTED_EDGE('',*,*,#31216,.F.);
#44537=ORIENTED_EDGE('',*,*,#31219,.F.);
#44538=ORIENTED_EDGE('',*,*,#31222,.F.);
#44539=ORIENTED_EDGE('',*,*,#31225,.F.);
#44540=ORIENTED_EDGE('',*,*,#31228,.F.);
#44541=ORIENTED_EDGE('',*,*,#31231,.F.);
#44542=ORIENTED_EDGE('',*,*,#31234,.F.);
#44543=ORIENTED_EDGE('',*,*,#31237,.F.);
#44544=ORIENTED_EDGE('',*,*,#31240,.F.);
#44545=ORIENTED_EDGE('',*,*,#31241,.T.);
#44546=ORIENTED_EDGE('',*,*,#31242,.T.);
#44547=ORIENTED_EDGE('',*,*,#31243,.F.);
#44548=ORIENTED_EDGE('',*,*,#31244,.F.);
#44549=ORIENTED_EDGE('',*,*,#31245,.T.);
#44550=ORIENTED_EDGE('',*,*,#31246,.T.);
#44551=ORIENTED_EDGE('',*,*,#31241,.F.);
#44552=ORIENTED_EDGE('',*,*,#31247,.F.);
#44553=ORIENTED_EDGE('',*,*,#31248,.T.);
#44554=ORIENTED_EDGE('',*,*,#31249,.T.);
#44555=ORIENTED_EDGE('',*,*,#31245,.F.);
#44556=ORIENTED_EDGE('',*,*,#31250,.F.);
#44557=ORIENTED_EDGE('',*,*,#31251,.T.);
#44558=ORIENTED_EDGE('',*,*,#31252,.T.);
#44559=ORIENTED_EDGE('',*,*,#31248,.F.);
#44560=ORIENTED_EDGE('',*,*,#31253,.F.);
#44561=ORIENTED_EDGE('',*,*,#31254,.T.);
#44562=ORIENTED_EDGE('',*,*,#31255,.T.);
#44563=ORIENTED_EDGE('',*,*,#31251,.F.);
#44564=ORIENTED_EDGE('',*,*,#31256,.F.);
#44565=ORIENTED_EDGE('',*,*,#31257,.T.);
#44566=ORIENTED_EDGE('',*,*,#31258,.T.);
#44567=ORIENTED_EDGE('',*,*,#31254,.F.);
#44568=ORIENTED_EDGE('',*,*,#31259,.F.);
#44569=ORIENTED_EDGE('',*,*,#31260,.T.);
#44570=ORIENTED_EDGE('',*,*,#31261,.T.);
#44571=ORIENTED_EDGE('',*,*,#31257,.F.);
#44572=ORIENTED_EDGE('',*,*,#31262,.F.);
#44573=ORIENTED_EDGE('',*,*,#31263,.T.);
#44574=ORIENTED_EDGE('',*,*,#31264,.T.);
#44575=ORIENTED_EDGE('',*,*,#31260,.F.);
#44576=ORIENTED_EDGE('',*,*,#31265,.F.);
#44577=ORIENTED_EDGE('',*,*,#31266,.T.);
#44578=ORIENTED_EDGE('',*,*,#31267,.T.);
#44579=ORIENTED_EDGE('',*,*,#31263,.F.);
#44580=ORIENTED_EDGE('',*,*,#31268,.F.);
#44581=ORIENTED_EDGE('',*,*,#31269,.T.);
#44582=ORIENTED_EDGE('',*,*,#31270,.T.);
#44583=ORIENTED_EDGE('',*,*,#31266,.F.);
#44584=ORIENTED_EDGE('',*,*,#31271,.F.);
#44585=ORIENTED_EDGE('',*,*,#31272,.T.);
#44586=ORIENTED_EDGE('',*,*,#31273,.T.);
#44587=ORIENTED_EDGE('',*,*,#31269,.F.);
#44588=ORIENTED_EDGE('',*,*,#31274,.F.);
#44589=ORIENTED_EDGE('',*,*,#31243,.T.);
#44590=ORIENTED_EDGE('',*,*,#31275,.T.);
#44591=ORIENTED_EDGE('',*,*,#31272,.F.);
#44592=ORIENTED_EDGE('',*,*,#31275,.F.);
#44593=ORIENTED_EDGE('',*,*,#31242,.F.);
#44594=ORIENTED_EDGE('',*,*,#31246,.F.);
#44595=ORIENTED_EDGE('',*,*,#31249,.F.);
#44596=ORIENTED_EDGE('',*,*,#31252,.F.);
#44597=ORIENTED_EDGE('',*,*,#31255,.F.);
#44598=ORIENTED_EDGE('',*,*,#31258,.F.);
#44599=ORIENTED_EDGE('',*,*,#31261,.F.);
#44600=ORIENTED_EDGE('',*,*,#31264,.F.);
#44601=ORIENTED_EDGE('',*,*,#31267,.F.);
#44602=ORIENTED_EDGE('',*,*,#31270,.F.);
#44603=ORIENTED_EDGE('',*,*,#31273,.F.);
#44604=ORIENTED_EDGE('',*,*,#31276,.F.);
#44605=ORIENTED_EDGE('',*,*,#31277,.T.);
#44606=ORIENTED_EDGE('',*,*,#31278,.T.);
#44607=ORIENTED_EDGE('',*,*,#31279,.F.);
#44608=ORIENTED_EDGE('',*,*,#31280,.F.);
#44609=ORIENTED_EDGE('',*,*,#31281,.T.);
#44610=ORIENTED_EDGE('',*,*,#31282,.T.);
#44611=ORIENTED_EDGE('',*,*,#31277,.F.);
#44612=ORIENTED_EDGE('',*,*,#31283,.F.);
#44613=ORIENTED_EDGE('',*,*,#31284,.T.);
#44614=ORIENTED_EDGE('',*,*,#31285,.T.);
#44615=ORIENTED_EDGE('',*,*,#31281,.F.);
#44616=ORIENTED_EDGE('',*,*,#31286,.F.);
#44617=ORIENTED_EDGE('',*,*,#31279,.T.);
#44618=ORIENTED_EDGE('',*,*,#31287,.T.);
#44619=ORIENTED_EDGE('',*,*,#31284,.F.);
#44620=ORIENTED_EDGE('',*,*,#31287,.F.);
#44621=ORIENTED_EDGE('',*,*,#31278,.F.);
#44622=ORIENTED_EDGE('',*,*,#31282,.F.);
#44623=ORIENTED_EDGE('',*,*,#31285,.F.);
#44624=ORIENTED_EDGE('',*,*,#31288,.F.);
#44625=ORIENTED_EDGE('',*,*,#31289,.T.);
#44626=ORIENTED_EDGE('',*,*,#31290,.T.);
#44627=ORIENTED_EDGE('',*,*,#31291,.F.);
#44628=ORIENTED_EDGE('',*,*,#31292,.F.);
#44629=ORIENTED_EDGE('',*,*,#31293,.T.);
#44630=ORIENTED_EDGE('',*,*,#31294,.T.);
#44631=ORIENTED_EDGE('',*,*,#31289,.F.);
#44632=ORIENTED_EDGE('',*,*,#31295,.F.);
#44633=ORIENTED_EDGE('',*,*,#31296,.T.);
#44634=ORIENTED_EDGE('',*,*,#31297,.T.);
#44635=ORIENTED_EDGE('',*,*,#31293,.F.);
#44636=ORIENTED_EDGE('',*,*,#31298,.F.);
#44637=ORIENTED_EDGE('',*,*,#31299,.T.);
#44638=ORIENTED_EDGE('',*,*,#31300,.T.);
#44639=ORIENTED_EDGE('',*,*,#31296,.F.);
#44640=ORIENTED_EDGE('',*,*,#31301,.F.);
#44641=ORIENTED_EDGE('',*,*,#31302,.T.);
#44642=ORIENTED_EDGE('',*,*,#31303,.T.);
#44643=ORIENTED_EDGE('',*,*,#31299,.F.);
#44644=ORIENTED_EDGE('',*,*,#31304,.F.);
#44645=ORIENTED_EDGE('',*,*,#31305,.T.);
#44646=ORIENTED_EDGE('',*,*,#31306,.T.);
#44647=ORIENTED_EDGE('',*,*,#31302,.F.);
#44648=ORIENTED_EDGE('',*,*,#31307,.F.);
#44649=ORIENTED_EDGE('',*,*,#31308,.T.);
#44650=ORIENTED_EDGE('',*,*,#31309,.T.);
#44651=ORIENTED_EDGE('',*,*,#31305,.F.);
#44652=ORIENTED_EDGE('',*,*,#31310,.F.);
#44653=ORIENTED_EDGE('',*,*,#31311,.T.);
#44654=ORIENTED_EDGE('',*,*,#31312,.T.);
#44655=ORIENTED_EDGE('',*,*,#31308,.F.);
#44656=ORIENTED_EDGE('',*,*,#31313,.F.);
#44657=ORIENTED_EDGE('',*,*,#31314,.T.);
#44658=ORIENTED_EDGE('',*,*,#31315,.T.);
#44659=ORIENTED_EDGE('',*,*,#31311,.F.);
#44660=ORIENTED_EDGE('',*,*,#31316,.F.);
#44661=ORIENTED_EDGE('',*,*,#31317,.T.);
#44662=ORIENTED_EDGE('',*,*,#31318,.T.);
#44663=ORIENTED_EDGE('',*,*,#31314,.F.);
#44664=ORIENTED_EDGE('',*,*,#31319,.F.);
#44665=ORIENTED_EDGE('',*,*,#31291,.T.);
#44666=ORIENTED_EDGE('',*,*,#31320,.T.);
#44667=ORIENTED_EDGE('',*,*,#31317,.F.);
#44668=ORIENTED_EDGE('',*,*,#31320,.F.);
#44669=ORIENTED_EDGE('',*,*,#31290,.F.);
#44670=ORIENTED_EDGE('',*,*,#31294,.F.);
#44671=ORIENTED_EDGE('',*,*,#31297,.F.);
#44672=ORIENTED_EDGE('',*,*,#31300,.F.);
#44673=ORIENTED_EDGE('',*,*,#31303,.F.);
#44674=ORIENTED_EDGE('',*,*,#31306,.F.);
#44675=ORIENTED_EDGE('',*,*,#31309,.F.);
#44676=ORIENTED_EDGE('',*,*,#31312,.F.);
#44677=ORIENTED_EDGE('',*,*,#31315,.F.);
#44678=ORIENTED_EDGE('',*,*,#31318,.F.);
#44679=ORIENTED_EDGE('',*,*,#31321,.F.);
#44680=ORIENTED_EDGE('',*,*,#31322,.T.);
#44681=ORIENTED_EDGE('',*,*,#31323,.T.);
#44682=ORIENTED_EDGE('',*,*,#31324,.F.);
#44683=ORIENTED_EDGE('',*,*,#31325,.F.);
#44684=ORIENTED_EDGE('',*,*,#31326,.T.);
#44685=ORIENTED_EDGE('',*,*,#31327,.T.);
#44686=ORIENTED_EDGE('',*,*,#31322,.F.);
#44687=ORIENTED_EDGE('',*,*,#31328,.F.);
#44688=ORIENTED_EDGE('',*,*,#31329,.T.);
#44689=ORIENTED_EDGE('',*,*,#31330,.T.);
#44690=ORIENTED_EDGE('',*,*,#31326,.F.);
#44691=ORIENTED_EDGE('',*,*,#31331,.F.);
#44692=ORIENTED_EDGE('',*,*,#31332,.T.);
#44693=ORIENTED_EDGE('',*,*,#31333,.T.);
#44694=ORIENTED_EDGE('',*,*,#31329,.F.);
#44695=ORIENTED_EDGE('',*,*,#31334,.F.);
#44696=ORIENTED_EDGE('',*,*,#31335,.T.);
#44697=ORIENTED_EDGE('',*,*,#31336,.T.);
#44698=ORIENTED_EDGE('',*,*,#31332,.F.);
#44699=ORIENTED_EDGE('',*,*,#31337,.F.);
#44700=ORIENTED_EDGE('',*,*,#31338,.T.);
#44701=ORIENTED_EDGE('',*,*,#31339,.T.);
#44702=ORIENTED_EDGE('',*,*,#31335,.F.);
#44703=ORIENTED_EDGE('',*,*,#31340,.F.);
#44704=ORIENTED_EDGE('',*,*,#31341,.T.);
#44705=ORIENTED_EDGE('',*,*,#31342,.T.);
#44706=ORIENTED_EDGE('',*,*,#31338,.F.);
#44707=ORIENTED_EDGE('',*,*,#31343,.F.);
#44708=ORIENTED_EDGE('',*,*,#31344,.T.);
#44709=ORIENTED_EDGE('',*,*,#31345,.T.);
#44710=ORIENTED_EDGE('',*,*,#31341,.F.);
#44711=ORIENTED_EDGE('',*,*,#31346,.F.);
#44712=ORIENTED_EDGE('',*,*,#31347,.T.);
#44713=ORIENTED_EDGE('',*,*,#31348,.T.);
#44714=ORIENTED_EDGE('',*,*,#31344,.F.);
#44715=ORIENTED_EDGE('',*,*,#31349,.F.);
#44716=ORIENTED_EDGE('',*,*,#31350,.T.);
#44717=ORIENTED_EDGE('',*,*,#31351,.T.);
#44718=ORIENTED_EDGE('',*,*,#31347,.F.);
#44719=ORIENTED_EDGE('',*,*,#31352,.F.);
#44720=ORIENTED_EDGE('',*,*,#31353,.T.);
#44721=ORIENTED_EDGE('',*,*,#31354,.T.);
#44722=ORIENTED_EDGE('',*,*,#31350,.F.);
#44723=ORIENTED_EDGE('',*,*,#31355,.F.);
#44724=ORIENTED_EDGE('',*,*,#31324,.T.);
#44725=ORIENTED_EDGE('',*,*,#31356,.T.);
#44726=ORIENTED_EDGE('',*,*,#31353,.F.);
#44727=ORIENTED_EDGE('',*,*,#31356,.F.);
#44728=ORIENTED_EDGE('',*,*,#31323,.F.);
#44729=ORIENTED_EDGE('',*,*,#31327,.F.);
#44730=ORIENTED_EDGE('',*,*,#31330,.F.);
#44731=ORIENTED_EDGE('',*,*,#31333,.F.);
#44732=ORIENTED_EDGE('',*,*,#31336,.F.);
#44733=ORIENTED_EDGE('',*,*,#31339,.F.);
#44734=ORIENTED_EDGE('',*,*,#31342,.F.);
#44735=ORIENTED_EDGE('',*,*,#31345,.F.);
#44736=ORIENTED_EDGE('',*,*,#31348,.F.);
#44737=ORIENTED_EDGE('',*,*,#31351,.F.);
#44738=ORIENTED_EDGE('',*,*,#31354,.F.);
#44739=ORIENTED_EDGE('',*,*,#31357,.F.);
#44740=ORIENTED_EDGE('',*,*,#31358,.T.);
#44741=ORIENTED_EDGE('',*,*,#31359,.T.);
#44742=ORIENTED_EDGE('',*,*,#31360,.F.);
#44743=ORIENTED_EDGE('',*,*,#31361,.F.);
#44744=ORIENTED_EDGE('',*,*,#31362,.T.);
#44745=ORIENTED_EDGE('',*,*,#31363,.T.);
#44746=ORIENTED_EDGE('',*,*,#31358,.F.);
#44747=ORIENTED_EDGE('',*,*,#31364,.F.);
#44748=ORIENTED_EDGE('',*,*,#31365,.T.);
#44749=ORIENTED_EDGE('',*,*,#31366,.T.);
#44750=ORIENTED_EDGE('',*,*,#31362,.F.);
#44751=ORIENTED_EDGE('',*,*,#31367,.F.);
#44752=ORIENTED_EDGE('',*,*,#31368,.T.);
#44753=ORIENTED_EDGE('',*,*,#31369,.T.);
#44754=ORIENTED_EDGE('',*,*,#31365,.F.);
#44755=ORIENTED_EDGE('',*,*,#31370,.F.);
#44756=ORIENTED_EDGE('',*,*,#31371,.T.);
#44757=ORIENTED_EDGE('',*,*,#31372,.T.);
#44758=ORIENTED_EDGE('',*,*,#31368,.F.);
#44759=ORIENTED_EDGE('',*,*,#31373,.F.);
#44760=ORIENTED_EDGE('',*,*,#31360,.T.);
#44761=ORIENTED_EDGE('',*,*,#31374,.T.);
#44762=ORIENTED_EDGE('',*,*,#31371,.F.);
#44763=ORIENTED_EDGE('',*,*,#31374,.F.);
#44764=ORIENTED_EDGE('',*,*,#31359,.F.);
#44765=ORIENTED_EDGE('',*,*,#31363,.F.);
#44766=ORIENTED_EDGE('',*,*,#31366,.F.);
#44767=ORIENTED_EDGE('',*,*,#31369,.F.);
#44768=ORIENTED_EDGE('',*,*,#31372,.F.);
#44769=ORIENTED_EDGE('',*,*,#31375,.F.);
#44770=ORIENTED_EDGE('',*,*,#31376,.T.);
#44771=ORIENTED_EDGE('',*,*,#31377,.T.);
#44772=ORIENTED_EDGE('',*,*,#31378,.F.);
#44773=ORIENTED_EDGE('',*,*,#31379,.F.);
#44774=ORIENTED_EDGE('',*,*,#31380,.T.);
#44775=ORIENTED_EDGE('',*,*,#31381,.T.);
#44776=ORIENTED_EDGE('',*,*,#31376,.F.);
#44777=ORIENTED_EDGE('',*,*,#31382,.F.);
#44778=ORIENTED_EDGE('',*,*,#31383,.T.);
#44779=ORIENTED_EDGE('',*,*,#31384,.T.);
#44780=ORIENTED_EDGE('',*,*,#31380,.F.);
#44781=ORIENTED_EDGE('',*,*,#31385,.F.);
#44782=ORIENTED_EDGE('',*,*,#31386,.T.);
#44783=ORIENTED_EDGE('',*,*,#31387,.T.);
#44784=ORIENTED_EDGE('',*,*,#31383,.F.);
#44785=ORIENTED_EDGE('',*,*,#31388,.F.);
#44786=ORIENTED_EDGE('',*,*,#31389,.T.);
#44787=ORIENTED_EDGE('',*,*,#31390,.T.);
#44788=ORIENTED_EDGE('',*,*,#31386,.F.);
#44789=ORIENTED_EDGE('',*,*,#31391,.F.);
#44790=ORIENTED_EDGE('',*,*,#31392,.T.);
#44791=ORIENTED_EDGE('',*,*,#31393,.T.);
#44792=ORIENTED_EDGE('',*,*,#31389,.F.);
#44793=ORIENTED_EDGE('',*,*,#31394,.F.);
#44794=ORIENTED_EDGE('',*,*,#31395,.T.);
#44795=ORIENTED_EDGE('',*,*,#31396,.T.);
#44796=ORIENTED_EDGE('',*,*,#31392,.F.);
#44797=ORIENTED_EDGE('',*,*,#31397,.F.);
#44798=ORIENTED_EDGE('',*,*,#31398,.T.);
#44799=ORIENTED_EDGE('',*,*,#31399,.T.);
#44800=ORIENTED_EDGE('',*,*,#31395,.F.);
#44801=ORIENTED_EDGE('',*,*,#31400,.F.);
#44802=ORIENTED_EDGE('',*,*,#31401,.T.);
#44803=ORIENTED_EDGE('',*,*,#31402,.T.);
#44804=ORIENTED_EDGE('',*,*,#31398,.F.);
#44805=ORIENTED_EDGE('',*,*,#31403,.F.);
#44806=ORIENTED_EDGE('',*,*,#31404,.T.);
#44807=ORIENTED_EDGE('',*,*,#31405,.T.);
#44808=ORIENTED_EDGE('',*,*,#31401,.F.);
#44809=ORIENTED_EDGE('',*,*,#31406,.F.);
#44810=ORIENTED_EDGE('',*,*,#31407,.T.);
#44811=ORIENTED_EDGE('',*,*,#31408,.T.);
#44812=ORIENTED_EDGE('',*,*,#31404,.F.);
#44813=ORIENTED_EDGE('',*,*,#31409,.F.);
#44814=ORIENTED_EDGE('',*,*,#31378,.T.);
#44815=ORIENTED_EDGE('',*,*,#31410,.T.);
#44816=ORIENTED_EDGE('',*,*,#31407,.F.);
#44817=ORIENTED_EDGE('',*,*,#31410,.F.);
#44818=ORIENTED_EDGE('',*,*,#31377,.F.);
#44819=ORIENTED_EDGE('',*,*,#31381,.F.);
#44820=ORIENTED_EDGE('',*,*,#31384,.F.);
#44821=ORIENTED_EDGE('',*,*,#31387,.F.);
#44822=ORIENTED_EDGE('',*,*,#31390,.F.);
#44823=ORIENTED_EDGE('',*,*,#31393,.F.);
#44824=ORIENTED_EDGE('',*,*,#31396,.F.);
#44825=ORIENTED_EDGE('',*,*,#31399,.F.);
#44826=ORIENTED_EDGE('',*,*,#31402,.F.);
#44827=ORIENTED_EDGE('',*,*,#31405,.F.);
#44828=ORIENTED_EDGE('',*,*,#31408,.F.);
#44829=ORIENTED_EDGE('',*,*,#31411,.F.);
#44830=ORIENTED_EDGE('',*,*,#31412,.T.);
#44831=ORIENTED_EDGE('',*,*,#31413,.T.);
#44832=ORIENTED_EDGE('',*,*,#31414,.F.);
#44833=ORIENTED_EDGE('',*,*,#31415,.F.);
#44834=ORIENTED_EDGE('',*,*,#31416,.T.);
#44835=ORIENTED_EDGE('',*,*,#31417,.T.);
#44836=ORIENTED_EDGE('',*,*,#31412,.F.);
#44837=ORIENTED_EDGE('',*,*,#31418,.F.);
#44838=ORIENTED_EDGE('',*,*,#31419,.T.);
#44839=ORIENTED_EDGE('',*,*,#31420,.T.);
#44840=ORIENTED_EDGE('',*,*,#31416,.F.);
#44841=ORIENTED_EDGE('',*,*,#31421,.F.);
#44842=ORIENTED_EDGE('',*,*,#31422,.T.);
#44843=ORIENTED_EDGE('',*,*,#31423,.T.);
#44844=ORIENTED_EDGE('',*,*,#31419,.F.);
#44845=ORIENTED_EDGE('',*,*,#31424,.F.);
#44846=ORIENTED_EDGE('',*,*,#31425,.T.);
#44847=ORIENTED_EDGE('',*,*,#31426,.T.);
#44848=ORIENTED_EDGE('',*,*,#31422,.F.);
#44849=ORIENTED_EDGE('',*,*,#31427,.F.);
#44850=ORIENTED_EDGE('',*,*,#31428,.T.);
#44851=ORIENTED_EDGE('',*,*,#31429,.T.);
#44852=ORIENTED_EDGE('',*,*,#31425,.F.);
#44853=ORIENTED_EDGE('',*,*,#31430,.F.);
#44854=ORIENTED_EDGE('',*,*,#31431,.T.);
#44855=ORIENTED_EDGE('',*,*,#31432,.T.);
#44856=ORIENTED_EDGE('',*,*,#31428,.F.);
#44857=ORIENTED_EDGE('',*,*,#31433,.F.);
#44858=ORIENTED_EDGE('',*,*,#31434,.T.);
#44859=ORIENTED_EDGE('',*,*,#31435,.T.);
#44860=ORIENTED_EDGE('',*,*,#31431,.F.);
#44861=ORIENTED_EDGE('',*,*,#31436,.F.);
#44862=ORIENTED_EDGE('',*,*,#31437,.T.);
#44863=ORIENTED_EDGE('',*,*,#31438,.T.);
#44864=ORIENTED_EDGE('',*,*,#31434,.F.);
#44865=ORIENTED_EDGE('',*,*,#31439,.F.);
#44866=ORIENTED_EDGE('',*,*,#31440,.T.);
#44867=ORIENTED_EDGE('',*,*,#31441,.T.);
#44868=ORIENTED_EDGE('',*,*,#31437,.F.);
#44869=ORIENTED_EDGE('',*,*,#31442,.F.);
#44870=ORIENTED_EDGE('',*,*,#31443,.T.);
#44871=ORIENTED_EDGE('',*,*,#31444,.T.);
#44872=ORIENTED_EDGE('',*,*,#31440,.F.);
#44873=ORIENTED_EDGE('',*,*,#31445,.F.);
#44874=ORIENTED_EDGE('',*,*,#31446,.T.);
#44875=ORIENTED_EDGE('',*,*,#31447,.T.);
#44876=ORIENTED_EDGE('',*,*,#31443,.F.);
#44877=ORIENTED_EDGE('',*,*,#31448,.F.);
#44878=ORIENTED_EDGE('',*,*,#31449,.T.);
#44879=ORIENTED_EDGE('',*,*,#31450,.T.);
#44880=ORIENTED_EDGE('',*,*,#31446,.F.);
#44881=ORIENTED_EDGE('',*,*,#31451,.F.);
#44882=ORIENTED_EDGE('',*,*,#31452,.T.);
#44883=ORIENTED_EDGE('',*,*,#31453,.T.);
#44884=ORIENTED_EDGE('',*,*,#31449,.F.);
#44885=ORIENTED_EDGE('',*,*,#31454,.F.);
#44886=ORIENTED_EDGE('',*,*,#31455,.T.);
#44887=ORIENTED_EDGE('',*,*,#31456,.T.);
#44888=ORIENTED_EDGE('',*,*,#31452,.F.);
#44889=ORIENTED_EDGE('',*,*,#31457,.F.);
#44890=ORIENTED_EDGE('',*,*,#31458,.T.);
#44891=ORIENTED_EDGE('',*,*,#31459,.T.);
#44892=ORIENTED_EDGE('',*,*,#31455,.F.);
#44893=ORIENTED_EDGE('',*,*,#31460,.F.);
#44894=ORIENTED_EDGE('',*,*,#31461,.T.);
#44895=ORIENTED_EDGE('',*,*,#31462,.T.);
#44896=ORIENTED_EDGE('',*,*,#31458,.F.);
#44897=ORIENTED_EDGE('',*,*,#31463,.F.);
#44898=ORIENTED_EDGE('',*,*,#31464,.T.);
#44899=ORIENTED_EDGE('',*,*,#31465,.T.);
#44900=ORIENTED_EDGE('',*,*,#31461,.F.);
#44901=ORIENTED_EDGE('',*,*,#31466,.F.);
#44902=ORIENTED_EDGE('',*,*,#31414,.T.);
#44903=ORIENTED_EDGE('',*,*,#31467,.T.);
#44904=ORIENTED_EDGE('',*,*,#31464,.F.);
#44905=ORIENTED_EDGE('',*,*,#31467,.F.);
#44906=ORIENTED_EDGE('',*,*,#31413,.F.);
#44907=ORIENTED_EDGE('',*,*,#31417,.F.);
#44908=ORIENTED_EDGE('',*,*,#31420,.F.);
#44909=ORIENTED_EDGE('',*,*,#31423,.F.);
#44910=ORIENTED_EDGE('',*,*,#31426,.F.);
#44911=ORIENTED_EDGE('',*,*,#31429,.F.);
#44912=ORIENTED_EDGE('',*,*,#31432,.F.);
#44913=ORIENTED_EDGE('',*,*,#31435,.F.);
#44914=ORIENTED_EDGE('',*,*,#31438,.F.);
#44915=ORIENTED_EDGE('',*,*,#31441,.F.);
#44916=ORIENTED_EDGE('',*,*,#31444,.F.);
#44917=ORIENTED_EDGE('',*,*,#31447,.F.);
#44918=ORIENTED_EDGE('',*,*,#31450,.F.);
#44919=ORIENTED_EDGE('',*,*,#31453,.F.);
#44920=ORIENTED_EDGE('',*,*,#31456,.F.);
#44921=ORIENTED_EDGE('',*,*,#31459,.F.);
#44922=ORIENTED_EDGE('',*,*,#31462,.F.);
#44923=ORIENTED_EDGE('',*,*,#31465,.F.);
#44924=ORIENTED_EDGE('',*,*,#31468,.F.);
#44925=ORIENTED_EDGE('',*,*,#31469,.F.);
#44926=ORIENTED_EDGE('',*,*,#31470,.F.);
#44927=ORIENTED_EDGE('',*,*,#31471,.T.);
#44928=ORIENTED_EDGE('',*,*,#31472,.F.);
#44929=ORIENTED_EDGE('',*,*,#31471,.F.);
#44930=ORIENTED_EDGE('',*,*,#31473,.F.);
#44931=ORIENTED_EDGE('',*,*,#31474,.T.);
#44932=ORIENTED_EDGE('',*,*,#31475,.F.);
#44933=ORIENTED_EDGE('',*,*,#31474,.F.);
#44934=ORIENTED_EDGE('',*,*,#31476,.F.);
#44935=ORIENTED_EDGE('',*,*,#31477,.T.);
#44936=ORIENTED_EDGE('',*,*,#31478,.F.);
#44937=ORIENTED_EDGE('',*,*,#31477,.F.);
#44938=ORIENTED_EDGE('',*,*,#31479,.F.);
#44939=ORIENTED_EDGE('',*,*,#31469,.T.);
#44940=ORIENTED_EDGE('',*,*,#31473,.T.);
#44941=ORIENTED_EDGE('',*,*,#31470,.T.);
#44942=ORIENTED_EDGE('',*,*,#31479,.T.);
#44943=ORIENTED_EDGE('',*,*,#31476,.T.);
#44944=ORIENTED_EDGE('',*,*,#31411,.T.);
#44945=ORIENTED_EDGE('',*,*,#31466,.T.);
#44946=ORIENTED_EDGE('',*,*,#31463,.T.);
#44947=ORIENTED_EDGE('',*,*,#31460,.T.);
#44948=ORIENTED_EDGE('',*,*,#31457,.T.);
#44949=ORIENTED_EDGE('',*,*,#31454,.T.);
#44950=ORIENTED_EDGE('',*,*,#31451,.T.);
#44951=ORIENTED_EDGE('',*,*,#31448,.T.);
#44952=ORIENTED_EDGE('',*,*,#31445,.T.);
#44953=ORIENTED_EDGE('',*,*,#31442,.T.);
#44954=ORIENTED_EDGE('',*,*,#31439,.T.);
#44955=ORIENTED_EDGE('',*,*,#31436,.T.);
#44956=ORIENTED_EDGE('',*,*,#31433,.T.);
#44957=ORIENTED_EDGE('',*,*,#31430,.T.);
#44958=ORIENTED_EDGE('',*,*,#31427,.T.);
#44959=ORIENTED_EDGE('',*,*,#31424,.T.);
#44960=ORIENTED_EDGE('',*,*,#31421,.T.);
#44961=ORIENTED_EDGE('',*,*,#31418,.T.);
#44962=ORIENTED_EDGE('',*,*,#31415,.T.);
#44963=ORIENTED_EDGE('',*,*,#31375,.T.);
#44964=ORIENTED_EDGE('',*,*,#31409,.T.);
#44965=ORIENTED_EDGE('',*,*,#31406,.T.);
#44966=ORIENTED_EDGE('',*,*,#31403,.T.);
#44967=ORIENTED_EDGE('',*,*,#31400,.T.);
#44968=ORIENTED_EDGE('',*,*,#31397,.T.);
#44969=ORIENTED_EDGE('',*,*,#31394,.T.);
#44970=ORIENTED_EDGE('',*,*,#31391,.T.);
#44971=ORIENTED_EDGE('',*,*,#31388,.T.);
#44972=ORIENTED_EDGE('',*,*,#31385,.T.);
#44973=ORIENTED_EDGE('',*,*,#31382,.T.);
#44974=ORIENTED_EDGE('',*,*,#31379,.T.);
#44975=ORIENTED_EDGE('',*,*,#31357,.T.);
#44976=ORIENTED_EDGE('',*,*,#31373,.T.);
#44977=ORIENTED_EDGE('',*,*,#31370,.T.);
#44978=ORIENTED_EDGE('',*,*,#31367,.T.);
#44979=ORIENTED_EDGE('',*,*,#31364,.T.);
#44980=ORIENTED_EDGE('',*,*,#31361,.T.);
#44981=ORIENTED_EDGE('',*,*,#31321,.T.);
#44982=ORIENTED_EDGE('',*,*,#31355,.T.);
#44983=ORIENTED_EDGE('',*,*,#31352,.T.);
#44984=ORIENTED_EDGE('',*,*,#31349,.T.);
#44985=ORIENTED_EDGE('',*,*,#31346,.T.);
#44986=ORIENTED_EDGE('',*,*,#31343,.T.);
#44987=ORIENTED_EDGE('',*,*,#31340,.T.);
#44988=ORIENTED_EDGE('',*,*,#31337,.T.);
#44989=ORIENTED_EDGE('',*,*,#31334,.T.);
#44990=ORIENTED_EDGE('',*,*,#31331,.T.);
#44991=ORIENTED_EDGE('',*,*,#31328,.T.);
#44992=ORIENTED_EDGE('',*,*,#31325,.T.);
#44993=ORIENTED_EDGE('',*,*,#31288,.T.);
#44994=ORIENTED_EDGE('',*,*,#31319,.T.);
#44995=ORIENTED_EDGE('',*,*,#31316,.T.);
#44996=ORIENTED_EDGE('',*,*,#31313,.T.);
#44997=ORIENTED_EDGE('',*,*,#31310,.T.);
#44998=ORIENTED_EDGE('',*,*,#31307,.T.);
#44999=ORIENTED_EDGE('',*,*,#31304,.T.);
#45000=ORIENTED_EDGE('',*,*,#31301,.T.);
#45001=ORIENTED_EDGE('',*,*,#31298,.T.);
#45002=ORIENTED_EDGE('',*,*,#31295,.T.);
#45003=ORIENTED_EDGE('',*,*,#31292,.T.);
#45004=ORIENTED_EDGE('',*,*,#31276,.T.);
#45005=ORIENTED_EDGE('',*,*,#31286,.T.);
#45006=ORIENTED_EDGE('',*,*,#31283,.T.);
#45007=ORIENTED_EDGE('',*,*,#31280,.T.);
#45008=ORIENTED_EDGE('',*,*,#31240,.T.);
#45009=ORIENTED_EDGE('',*,*,#31274,.T.);
#45010=ORIENTED_EDGE('',*,*,#31271,.T.);
#45011=ORIENTED_EDGE('',*,*,#31268,.T.);
#45012=ORIENTED_EDGE('',*,*,#31265,.T.);
#45013=ORIENTED_EDGE('',*,*,#31262,.T.);
#45014=ORIENTED_EDGE('',*,*,#31259,.T.);
#45015=ORIENTED_EDGE('',*,*,#31256,.T.);
#45016=ORIENTED_EDGE('',*,*,#31253,.T.);
#45017=ORIENTED_EDGE('',*,*,#31250,.T.);
#45018=ORIENTED_EDGE('',*,*,#31247,.T.);
#45019=ORIENTED_EDGE('',*,*,#31244,.T.);
#45020=ORIENTED_EDGE('',*,*,#31195,.T.);
#45021=ORIENTED_EDGE('',*,*,#31238,.T.);
#45022=ORIENTED_EDGE('',*,*,#31235,.T.);
#45023=ORIENTED_EDGE('',*,*,#31232,.T.);
#45024=ORIENTED_EDGE('',*,*,#31229,.T.);
#45025=ORIENTED_EDGE('',*,*,#31226,.T.);
#45026=ORIENTED_EDGE('',*,*,#31223,.T.);
#45027=ORIENTED_EDGE('',*,*,#31220,.T.);
#45028=ORIENTED_EDGE('',*,*,#31217,.T.);
#45029=ORIENTED_EDGE('',*,*,#31214,.T.);
#45030=ORIENTED_EDGE('',*,*,#31211,.T.);
#45031=ORIENTED_EDGE('',*,*,#31208,.T.);
#45032=ORIENTED_EDGE('',*,*,#31205,.T.);
#45033=ORIENTED_EDGE('',*,*,#31202,.T.);
#45034=ORIENTED_EDGE('',*,*,#31199,.T.);
#45035=ORIENTED_EDGE('',*,*,#31162,.T.);
#45036=ORIENTED_EDGE('',*,*,#31193,.T.);
#45037=ORIENTED_EDGE('',*,*,#31190,.T.);
#45038=ORIENTED_EDGE('',*,*,#31187,.T.);
#45039=ORIENTED_EDGE('',*,*,#31184,.T.);
#45040=ORIENTED_EDGE('',*,*,#31181,.T.);
#45041=ORIENTED_EDGE('',*,*,#31178,.T.);
#45042=ORIENTED_EDGE('',*,*,#31175,.T.);
#45043=ORIENTED_EDGE('',*,*,#31172,.T.);
#45044=ORIENTED_EDGE('',*,*,#31169,.T.);
#45045=ORIENTED_EDGE('',*,*,#31166,.T.);
#45046=ORIENTED_EDGE('',*,*,#31096,.T.);
#45047=ORIENTED_EDGE('',*,*,#31160,.T.);
#45048=ORIENTED_EDGE('',*,*,#31157,.T.);
#45049=ORIENTED_EDGE('',*,*,#31154,.T.);
#45050=ORIENTED_EDGE('',*,*,#31151,.T.);
#45051=ORIENTED_EDGE('',*,*,#31148,.T.);
#45052=ORIENTED_EDGE('',*,*,#31145,.T.);
#45053=ORIENTED_EDGE('',*,*,#31142,.T.);
#45054=ORIENTED_EDGE('',*,*,#31139,.T.);
#45055=ORIENTED_EDGE('',*,*,#31136,.T.);
#45056=ORIENTED_EDGE('',*,*,#31133,.T.);
#45057=ORIENTED_EDGE('',*,*,#31130,.T.);
#45058=ORIENTED_EDGE('',*,*,#31127,.T.);
#45059=ORIENTED_EDGE('',*,*,#31124,.T.);
#45060=ORIENTED_EDGE('',*,*,#31121,.T.);
#45061=ORIENTED_EDGE('',*,*,#31118,.T.);
#45062=ORIENTED_EDGE('',*,*,#31115,.T.);
#45063=ORIENTED_EDGE('',*,*,#31112,.T.);
#45064=ORIENTED_EDGE('',*,*,#31109,.T.);
#45065=ORIENTED_EDGE('',*,*,#31106,.T.);
#45066=ORIENTED_EDGE('',*,*,#31103,.T.);
#45067=ORIENTED_EDGE('',*,*,#31100,.T.);
#45068=ORIENTED_EDGE('',*,*,#31084,.T.);
#45069=ORIENTED_EDGE('',*,*,#31094,.T.);
#45070=ORIENTED_EDGE('',*,*,#31091,.T.);
#45071=ORIENTED_EDGE('',*,*,#31088,.T.);
#45072=ORIENTED_EDGE('',*,*,#31057,.T.);
#45073=ORIENTED_EDGE('',*,*,#31082,.T.);
#45074=ORIENTED_EDGE('',*,*,#31079,.T.);
#45075=ORIENTED_EDGE('',*,*,#31076,.T.);
#45076=ORIENTED_EDGE('',*,*,#31073,.T.);
#45077=ORIENTED_EDGE('',*,*,#31070,.T.);
#45078=ORIENTED_EDGE('',*,*,#31067,.T.);
#45079=ORIENTED_EDGE('',*,*,#31064,.T.);
#45080=ORIENTED_EDGE('',*,*,#31061,.T.);
#45081=ORIENTED_EDGE('',*,*,#31021,.T.);
#45082=ORIENTED_EDGE('',*,*,#31055,.T.);
#45083=ORIENTED_EDGE('',*,*,#31052,.T.);
#45084=ORIENTED_EDGE('',*,*,#31049,.T.);
#45085=ORIENTED_EDGE('',*,*,#31046,.T.);
#45086=ORIENTED_EDGE('',*,*,#31043,.T.);
#45087=ORIENTED_EDGE('',*,*,#31040,.T.);
#45088=ORIENTED_EDGE('',*,*,#31037,.T.);
#45089=ORIENTED_EDGE('',*,*,#31034,.T.);
#45090=ORIENTED_EDGE('',*,*,#31031,.T.);
#45091=ORIENTED_EDGE('',*,*,#31028,.T.);
#45092=ORIENTED_EDGE('',*,*,#31025,.T.);
#45093=ORIENTED_EDGE('',*,*,#30994,.T.);
#45094=ORIENTED_EDGE('',*,*,#31019,.T.);
#45095=ORIENTED_EDGE('',*,*,#31016,.T.);
#45096=ORIENTED_EDGE('',*,*,#31013,.T.);
#45097=ORIENTED_EDGE('',*,*,#31010,.T.);
#45098=ORIENTED_EDGE('',*,*,#31007,.T.);
#45099=ORIENTED_EDGE('',*,*,#31004,.T.);
#45100=ORIENTED_EDGE('',*,*,#31001,.T.);
#45101=ORIENTED_EDGE('',*,*,#30998,.T.);
#45102=ORIENTED_EDGE('',*,*,#30970,.T.);
#45103=ORIENTED_EDGE('',*,*,#30992,.T.);
#45104=ORIENTED_EDGE('',*,*,#30989,.T.);
#45105=ORIENTED_EDGE('',*,*,#30986,.T.);
#45106=ORIENTED_EDGE('',*,*,#30983,.T.);
#45107=ORIENTED_EDGE('',*,*,#30980,.T.);
#45108=ORIENTED_EDGE('',*,*,#30977,.T.);
#45109=ORIENTED_EDGE('',*,*,#30974,.T.);
#45110=ORIENTED_EDGE('',*,*,#30913,.T.);
#45111=ORIENTED_EDGE('',*,*,#30968,.T.);
#45112=ORIENTED_EDGE('',*,*,#30965,.T.);
#45113=ORIENTED_EDGE('',*,*,#30962,.T.);
#45114=ORIENTED_EDGE('',*,*,#30959,.T.);
#45115=ORIENTED_EDGE('',*,*,#30956,.T.);
#45116=ORIENTED_EDGE('',*,*,#30953,.T.);
#45117=ORIENTED_EDGE('',*,*,#30950,.T.);
#45118=ORIENTED_EDGE('',*,*,#30947,.T.);
#45119=ORIENTED_EDGE('',*,*,#30944,.T.);
#45120=ORIENTED_EDGE('',*,*,#30941,.T.);
#45121=ORIENTED_EDGE('',*,*,#30938,.T.);
#45122=ORIENTED_EDGE('',*,*,#30935,.T.);
#45123=ORIENTED_EDGE('',*,*,#30932,.T.);
#45124=ORIENTED_EDGE('',*,*,#30929,.T.);
#45125=ORIENTED_EDGE('',*,*,#30926,.T.);
#45126=ORIENTED_EDGE('',*,*,#30923,.T.);
#45127=ORIENTED_EDGE('',*,*,#30920,.T.);
#45128=ORIENTED_EDGE('',*,*,#30917,.T.);
#45129=ORIENTED_EDGE('',*,*,#30862,.T.);
#45130=ORIENTED_EDGE('',*,*,#30911,.T.);
#45131=ORIENTED_EDGE('',*,*,#30908,.T.);
#45132=ORIENTED_EDGE('',*,*,#30905,.T.);
#45133=ORIENTED_EDGE('',*,*,#30902,.T.);
#45134=ORIENTED_EDGE('',*,*,#30899,.T.);
#45135=ORIENTED_EDGE('',*,*,#30896,.T.);
#45136=ORIENTED_EDGE('',*,*,#30893,.T.);
#45137=ORIENTED_EDGE('',*,*,#30890,.T.);
#45138=ORIENTED_EDGE('',*,*,#30887,.T.);
#45139=ORIENTED_EDGE('',*,*,#30884,.T.);
#45140=ORIENTED_EDGE('',*,*,#30881,.T.);
#45141=ORIENTED_EDGE('',*,*,#30878,.T.);
#45142=ORIENTED_EDGE('',*,*,#30875,.T.);
#45143=ORIENTED_EDGE('',*,*,#30872,.T.);
#45144=ORIENTED_EDGE('',*,*,#30869,.T.);
#45145=ORIENTED_EDGE('',*,*,#30866,.T.);
#45146=ORIENTED_EDGE('',*,*,#30838,.T.);
#45147=ORIENTED_EDGE('',*,*,#30860,.T.);
#45148=ORIENTED_EDGE('',*,*,#30857,.T.);
#45149=ORIENTED_EDGE('',*,*,#30854,.T.);
#45150=ORIENTED_EDGE('',*,*,#30851,.T.);
#45151=ORIENTED_EDGE('',*,*,#30848,.T.);
#45152=ORIENTED_EDGE('',*,*,#30845,.T.);
#45153=ORIENTED_EDGE('',*,*,#30842,.T.);
#45154=ORIENTED_EDGE('',*,*,#30820,.T.);
#45155=ORIENTED_EDGE('',*,*,#30836,.T.);
#45156=ORIENTED_EDGE('',*,*,#30833,.T.);
#45157=ORIENTED_EDGE('',*,*,#30830,.T.);
#45158=ORIENTED_EDGE('',*,*,#30827,.T.);
#45159=ORIENTED_EDGE('',*,*,#30824,.T.);
#45160=ORIENTED_EDGE('',*,*,#30754,.T.);
#45161=ORIENTED_EDGE('',*,*,#30818,.T.);
#45162=ORIENTED_EDGE('',*,*,#30815,.T.);
#45163=ORIENTED_EDGE('',*,*,#30812,.T.);
#45164=ORIENTED_EDGE('',*,*,#30809,.T.);
#45165=ORIENTED_EDGE('',*,*,#30806,.T.);
#45166=ORIENTED_EDGE('',*,*,#30803,.T.);
#45167=ORIENTED_EDGE('',*,*,#30800,.T.);
#45168=ORIENTED_EDGE('',*,*,#30797,.T.);
#45169=ORIENTED_EDGE('',*,*,#30794,.T.);
#45170=ORIENTED_EDGE('',*,*,#30791,.T.);
#45171=ORIENTED_EDGE('',*,*,#30788,.T.);
#45172=ORIENTED_EDGE('',*,*,#30785,.T.);
#45173=ORIENTED_EDGE('',*,*,#30782,.T.);
#45174=ORIENTED_EDGE('',*,*,#30779,.T.);
#45175=ORIENTED_EDGE('',*,*,#30776,.T.);
#45176=ORIENTED_EDGE('',*,*,#30773,.T.);
#45177=ORIENTED_EDGE('',*,*,#30770,.T.);
#45178=ORIENTED_EDGE('',*,*,#30767,.T.);
#45179=ORIENTED_EDGE('',*,*,#30764,.T.);
#45180=ORIENTED_EDGE('',*,*,#30761,.T.);
#45181=ORIENTED_EDGE('',*,*,#30758,.T.);
#45182=ORIENTED_EDGE('',*,*,#30649,.T.);
#45183=ORIENTED_EDGE('',*,*,#30752,.T.);
#45184=ORIENTED_EDGE('',*,*,#30749,.T.);
#45185=ORIENTED_EDGE('',*,*,#30746,.T.);
#45186=ORIENTED_EDGE('',*,*,#30743,.T.);
#45187=ORIENTED_EDGE('',*,*,#30740,.T.);
#45188=ORIENTED_EDGE('',*,*,#30737,.T.);
#45189=ORIENTED_EDGE('',*,*,#30734,.T.);
#45190=ORIENTED_EDGE('',*,*,#30731,.T.);
#45191=ORIENTED_EDGE('',*,*,#30728,.T.);
#45192=ORIENTED_EDGE('',*,*,#30725,.T.);
#45193=ORIENTED_EDGE('',*,*,#30722,.T.);
#45194=ORIENTED_EDGE('',*,*,#30719,.T.);
#45195=ORIENTED_EDGE('',*,*,#30716,.T.);
#45196=ORIENTED_EDGE('',*,*,#30713,.T.);
#45197=ORIENTED_EDGE('',*,*,#30710,.T.);
#45198=ORIENTED_EDGE('',*,*,#30707,.T.);
#45199=ORIENTED_EDGE('',*,*,#30704,.T.);
#45200=ORIENTED_EDGE('',*,*,#30701,.T.);
#45201=ORIENTED_EDGE('',*,*,#30698,.T.);
#45202=ORIENTED_EDGE('',*,*,#30695,.T.);
#45203=ORIENTED_EDGE('',*,*,#30692,.T.);
#45204=ORIENTED_EDGE('',*,*,#30689,.T.);
#45205=ORIENTED_EDGE('',*,*,#30686,.T.);
#45206=ORIENTED_EDGE('',*,*,#30683,.T.);
#45207=ORIENTED_EDGE('',*,*,#30680,.T.);
#45208=ORIENTED_EDGE('',*,*,#30677,.T.);
#45209=ORIENTED_EDGE('',*,*,#30674,.T.);
#45210=ORIENTED_EDGE('',*,*,#30671,.T.);
#45211=ORIENTED_EDGE('',*,*,#30668,.T.);
#45212=ORIENTED_EDGE('',*,*,#30665,.T.);
#45213=ORIENTED_EDGE('',*,*,#30662,.T.);
#45214=ORIENTED_EDGE('',*,*,#30659,.T.);
#45215=ORIENTED_EDGE('',*,*,#30656,.T.);
#45216=ORIENTED_EDGE('',*,*,#30653,.T.);
#45217=ORIENTED_EDGE('',*,*,#30637,.T.);
#45218=ORIENTED_EDGE('',*,*,#30647,.T.);
#45219=ORIENTED_EDGE('',*,*,#30644,.T.);
#45220=ORIENTED_EDGE('',*,*,#30641,.T.);
#45221=ORIENTED_EDGE('',*,*,#30601,.T.);
#45222=ORIENTED_EDGE('',*,*,#30635,.T.);
#45223=ORIENTED_EDGE('',*,*,#30632,.T.);
#45224=ORIENTED_EDGE('',*,*,#30629,.T.);
#45225=ORIENTED_EDGE('',*,*,#30626,.T.);
#45226=ORIENTED_EDGE('',*,*,#30623,.T.);
#45227=ORIENTED_EDGE('',*,*,#30620,.T.);
#45228=ORIENTED_EDGE('',*,*,#30617,.T.);
#45229=ORIENTED_EDGE('',*,*,#30614,.T.);
#45230=ORIENTED_EDGE('',*,*,#30611,.T.);
#45231=ORIENTED_EDGE('',*,*,#30608,.T.);
#45232=ORIENTED_EDGE('',*,*,#30605,.T.);
#45233=ORIENTED_EDGE('',*,*,#31480,.T.);
#45234=ORIENTED_EDGE('',*,*,#31481,.T.);
#45235=ORIENTED_EDGE('',*,*,#31482,.T.);
#45236=ORIENTED_EDGE('',*,*,#31481,.F.);
#45237=ORIENTED_EDGE('',*,*,#31483,.F.);
#45238=ORIENTED_EDGE('',*,*,#31484,.T.);
#45239=ORIENTED_EDGE('',*,*,#31482,.F.);
#45240=ORIENTED_EDGE('',*,*,#31484,.F.);
#45241=ORIENTED_EDGE('',*,*,#31485,.F.);
#45242=ORIENTED_EDGE('',*,*,#31486,.F.);
#45243=ORIENTED_EDGE('',*,*,#31487,.F.);
#45244=ORIENTED_EDGE('',*,*,#31488,.F.);
#45245=ORIENTED_EDGE('',*,*,#31489,.F.);
#45246=ORIENTED_EDGE('',*,*,#31490,.F.);
#45247=ORIENTED_EDGE('',*,*,#31491,.F.);
#45248=ORIENTED_EDGE('',*,*,#31492,.F.);
#45249=ORIENTED_EDGE('',*,*,#31480,.F.);
#45250=ORIENTED_EDGE('',*,*,#31493,.F.);
#45251=ORIENTED_EDGE('',*,*,#31494,.T.);
#45252=ORIENTED_EDGE('',*,*,#31495,.T.);
#45253=ORIENTED_EDGE('',*,*,#31496,.T.);
#45254=ORIENTED_EDGE('',*,*,#31497,.T.);
#45255=ORIENTED_EDGE('',*,*,#31498,.T.);
#45256=ORIENTED_EDGE('',*,*,#31499,.T.);
#45257=ORIENTED_EDGE('',*,*,#31500,.T.);
#45258=ORIENTED_EDGE('',*,*,#31501,.F.);
#45259=ORIENTED_EDGE('',*,*,#31502,.F.);
#45260=ORIENTED_EDGE('',*,*,#31475,.T.);
#45261=ORIENTED_EDGE('',*,*,#31478,.T.);
#45262=ORIENTED_EDGE('',*,*,#31468,.T.);
#45263=ORIENTED_EDGE('',*,*,#31472,.T.);
#45264=ORIENTED_EDGE('',*,*,#31503,.T.);
#45265=ORIENTED_EDGE('',*,*,#31504,.T.);
#45266=ORIENTED_EDGE('',*,*,#31483,.T.);
#45267=ORIENTED_EDGE('',*,*,#31504,.F.);
#45268=ORIENTED_EDGE('',*,*,#31505,.F.);
#45269=ORIENTED_EDGE('',*,*,#31506,.F.);
#45270=ORIENTED_EDGE('',*,*,#31507,.F.);
#45271=ORIENTED_EDGE('',*,*,#31508,.F.);
#45272=ORIENTED_EDGE('',*,*,#31509,.F.);
#45273=ORIENTED_EDGE('',*,*,#31510,.F.);
#45274=ORIENTED_EDGE('',*,*,#31511,.F.);
#45275=ORIENTED_EDGE('',*,*,#31512,.F.);
#45276=ORIENTED_EDGE('',*,*,#31513,.F.);
#45277=ORIENTED_EDGE('',*,*,#31514,.F.);
#45278=ORIENTED_EDGE('',*,*,#31515,.F.);
#45279=ORIENTED_EDGE('',*,*,#31503,.F.);
#45280=ORIENTED_EDGE('',*,*,#31502,.T.);
#45281=ORIENTED_EDGE('',*,*,#31516,.T.);
#45282=ORIENTED_EDGE('',*,*,#31517,.T.);
#45283=ORIENTED_EDGE('',*,*,#31516,.F.);
#45284=ORIENTED_EDGE('',*,*,#31518,.F.);
#45285=ORIENTED_EDGE('',*,*,#31519,.T.);
#45286=ORIENTED_EDGE('',*,*,#31517,.F.);
#45287=ORIENTED_EDGE('',*,*,#31519,.F.);
#45288=ORIENTED_EDGE('',*,*,#31513,.T.);
#45289=ORIENTED_EDGE('',*,*,#31520,.T.);
#45290=ORIENTED_EDGE('',*,*,#31518,.T.);
#45291=ORIENTED_EDGE('',*,*,#31520,.F.);
#45292=ORIENTED_EDGE('',*,*,#31493,.T.);
#45293=ORIENTED_EDGE('',*,*,#31521,.T.);
#45294=ORIENTED_EDGE('',*,*,#31522,.T.);
#45295=ORIENTED_EDGE('',*,*,#31521,.F.);
#45296=ORIENTED_EDGE('',*,*,#31523,.F.);
#45297=ORIENTED_EDGE('',*,*,#31524,.T.);
#45298=ORIENTED_EDGE('',*,*,#31522,.F.);
#45299=ORIENTED_EDGE('',*,*,#31524,.F.);
#45300=ORIENTED_EDGE('',*,*,#31515,.T.);
#45301=ORIENTED_EDGE('',*,*,#31525,.T.);
#45302=ORIENTED_EDGE('',*,*,#31523,.T.);
#45303=ORIENTED_EDGE('',*,*,#31525,.F.);
#45304=ORIENTED_EDGE('',*,*,#31501,.T.);
#45305=ORIENTED_EDGE('',*,*,#31526,.T.);
#45306=ORIENTED_EDGE('',*,*,#31527,.T.);
#45307=ORIENTED_EDGE('',*,*,#31526,.F.);
#45308=ORIENTED_EDGE('',*,*,#31528,.F.);
#45309=ORIENTED_EDGE('',*,*,#31529,.T.);
#45310=ORIENTED_EDGE('',*,*,#31527,.F.);
#45311=ORIENTED_EDGE('',*,*,#31529,.F.);
#45312=ORIENTED_EDGE('',*,*,#31514,.T.);
#45313=ORIENTED_EDGE('',*,*,#31530,.T.);
#45314=ORIENTED_EDGE('',*,*,#31528,.T.);
#45315=ORIENTED_EDGE('',*,*,#31530,.F.);
#45316=ORIENTED_EDGE('',*,*,#31531,.F.);
#45317=ORIENTED_EDGE('',*,*,#31532,.T.);
#45318=ORIENTED_EDGE('',*,*,#31532,.F.);
#45319=ORIENTED_EDGE('',*,*,#31500,.F.);
#45320=ORIENTED_EDGE('',*,*,#31533,.T.);
#45321=ORIENTED_EDGE('',*,*,#31531,.T.);
#45322=ORIENTED_EDGE('',*,*,#31533,.F.);
#45323=ORIENTED_EDGE('',*,*,#31534,.F.);
#45324=ORIENTED_EDGE('',*,*,#31535,.T.);
#45325=ORIENTED_EDGE('',*,*,#31535,.F.);
#45326=ORIENTED_EDGE('',*,*,#31499,.F.);
#45327=ORIENTED_EDGE('',*,*,#31536,.T.);
#45328=ORIENTED_EDGE('',*,*,#31534,.T.);
#45329=ORIENTED_EDGE('',*,*,#31536,.F.);
#45330=ORIENTED_EDGE('',*,*,#31537,.F.);
#45331=ORIENTED_EDGE('',*,*,#31538,.T.);
#45332=ORIENTED_EDGE('',*,*,#31538,.F.);
#45333=ORIENTED_EDGE('',*,*,#31494,.F.);
#45334=ORIENTED_EDGE('',*,*,#31539,.T.);
#45335=ORIENTED_EDGE('',*,*,#31540,.T.);
#45336=ORIENTED_EDGE('',*,*,#31539,.F.);
#45337=ORIENTED_EDGE('',*,*,#31540,.F.);
#45338=ORIENTED_EDGE('',*,*,#31541,.T.);
#45339=ORIENTED_EDGE('',*,*,#31537,.T.);
#45340=ORIENTED_EDGE('',*,*,#31541,.F.);
#45341=ORIENTED_EDGE('',*,*,#31542,.F.);
#45342=ORIENTED_EDGE('',*,*,#31543,.T.);
#45343=ORIENTED_EDGE('',*,*,#31543,.F.);
#45344=ORIENTED_EDGE('',*,*,#31495,.F.);
#45345=ORIENTED_EDGE('',*,*,#31544,.T.);
#45346=ORIENTED_EDGE('',*,*,#31545,.T.);
#45347=ORIENTED_EDGE('',*,*,#31544,.F.);
#45348=ORIENTED_EDGE('',*,*,#31545,.F.);
#45349=ORIENTED_EDGE('',*,*,#31546,.T.);
#45350=ORIENTED_EDGE('',*,*,#31542,.T.);
#45351=ORIENTED_EDGE('',*,*,#31546,.F.);
#45352=ORIENTED_EDGE('',*,*,#31547,.F.);
#45353=ORIENTED_EDGE('',*,*,#31548,.T.);
#45354=ORIENTED_EDGE('',*,*,#31548,.F.);
#45355=ORIENTED_EDGE('',*,*,#31496,.F.);
#45356=ORIENTED_EDGE('',*,*,#31549,.T.);
#45357=ORIENTED_EDGE('',*,*,#31550,.T.);
#45358=ORIENTED_EDGE('',*,*,#31549,.F.);
#45359=ORIENTED_EDGE('',*,*,#31550,.F.);
#45360=ORIENTED_EDGE('',*,*,#31551,.T.);
#45361=ORIENTED_EDGE('',*,*,#31547,.T.);
#45362=ORIENTED_EDGE('',*,*,#31551,.F.);
#45363=ORIENTED_EDGE('',*,*,#31552,.F.);
#45364=ORIENTED_EDGE('',*,*,#31553,.T.);
#45365=ORIENTED_EDGE('',*,*,#31553,.F.);
#45366=ORIENTED_EDGE('',*,*,#31497,.F.);
#45367=ORIENTED_EDGE('',*,*,#31554,.T.);
#45368=ORIENTED_EDGE('',*,*,#31555,.T.);
#45369=ORIENTED_EDGE('',*,*,#31554,.F.);
#45370=ORIENTED_EDGE('',*,*,#31555,.F.);
#45371=ORIENTED_EDGE('',*,*,#31556,.T.);
#45372=ORIENTED_EDGE('',*,*,#31552,.T.);
#45373=ORIENTED_EDGE('',*,*,#31556,.F.);
#45374=ORIENTED_EDGE('',*,*,#31557,.F.);
#45375=ORIENTED_EDGE('',*,*,#31558,.T.);
#45376=ORIENTED_EDGE('',*,*,#31498,.F.);
#45377=ORIENTED_EDGE('',*,*,#31558,.F.);
#45378=ORIENTED_EDGE('',*,*,#31557,.T.);
#45379=ORIENTED_EDGE('',*,*,#31559,.T.);
#45380=ORIENTED_EDGE('',*,*,#31560,.T.);
#45381=ORIENTED_EDGE('',*,*,#31561,.T.);
#45382=ORIENTED_EDGE('',*,*,#31505,.T.);
#45383=ORIENTED_EDGE('',*,*,#31562,.T.);
#45384=ORIENTED_EDGE('',*,*,#31563,.T.);
#45385=ORIENTED_EDGE('',*,*,#31559,.F.);
#45386=ORIENTED_EDGE('',*,*,#31512,.T.);
#45387=ORIENTED_EDGE('',*,*,#31564,.T.);
#45388=ORIENTED_EDGE('',*,*,#31565,.T.);
#45389=ORIENTED_EDGE('',*,*,#31562,.F.);
#45390=ORIENTED_EDGE('',*,*,#31511,.T.);
#45391=ORIENTED_EDGE('',*,*,#31566,.T.);
#45392=ORIENTED_EDGE('',*,*,#31567,.T.);
#45393=ORIENTED_EDGE('',*,*,#31564,.F.);
#45394=ORIENTED_EDGE('',*,*,#31510,.T.);
#45395=ORIENTED_EDGE('',*,*,#31568,.T.);
#45396=ORIENTED_EDGE('',*,*,#31569,.T.);
#45397=ORIENTED_EDGE('',*,*,#31566,.F.);
#45398=ORIENTED_EDGE('',*,*,#31509,.T.);
#45399=ORIENTED_EDGE('',*,*,#31570,.T.);
#45400=ORIENTED_EDGE('',*,*,#31571,.T.);
#45401=ORIENTED_EDGE('',*,*,#31568,.F.);
#45402=ORIENTED_EDGE('',*,*,#31508,.T.);
#45403=ORIENTED_EDGE('',*,*,#31572,.T.);
#45404=ORIENTED_EDGE('',*,*,#31573,.T.);
#45405=ORIENTED_EDGE('',*,*,#31570,.F.);
#45406=ORIENTED_EDGE('',*,*,#31507,.T.);
#45407=ORIENTED_EDGE('',*,*,#31561,.F.);
#45408=ORIENTED_EDGE('',*,*,#31574,.T.);
#45409=ORIENTED_EDGE('',*,*,#31572,.F.);
#45410=ORIENTED_EDGE('',*,*,#31506,.T.);
#45411=ORIENTED_EDGE('',*,*,#31571,.F.);
#45412=ORIENTED_EDGE('',*,*,#31575,.T.);
#45413=ORIENTED_EDGE('',*,*,#31576,.F.);
#45414=ORIENTED_EDGE('',*,*,#31577,.F.);
#45415=ORIENTED_EDGE('',*,*,#31573,.F.);
#45416=ORIENTED_EDGE('',*,*,#31578,.T.);
#45417=ORIENTED_EDGE('',*,*,#31579,.F.);
#45418=ORIENTED_EDGE('',*,*,#31575,.F.);
#45419=ORIENTED_EDGE('',*,*,#31574,.F.);
#45420=ORIENTED_EDGE('',*,*,#31580,.T.);
#45421=ORIENTED_EDGE('',*,*,#31581,.F.);
#45422=ORIENTED_EDGE('',*,*,#31578,.F.);
#45423=ORIENTED_EDGE('',*,*,#31560,.F.);
#45424=ORIENTED_EDGE('',*,*,#31582,.T.);
#45425=ORIENTED_EDGE('',*,*,#31583,.F.);
#45426=ORIENTED_EDGE('',*,*,#31580,.F.);
#45427=ORIENTED_EDGE('',*,*,#31584,.T.);
#45428=ORIENTED_EDGE('',*,*,#31485,.T.);
#45429=ORIENTED_EDGE('',*,*,#31585,.T.);
#45430=ORIENTED_EDGE('',*,*,#31576,.T.);
#45431=ORIENTED_EDGE('',*,*,#31586,.T.);
#45432=ORIENTED_EDGE('',*,*,#31486,.T.);
#45433=ORIENTED_EDGE('',*,*,#31584,.F.);
#45434=ORIENTED_EDGE('',*,*,#31579,.T.);
#45435=ORIENTED_EDGE('',*,*,#31587,.T.);
#45436=ORIENTED_EDGE('',*,*,#31487,.T.);
#45437=ORIENTED_EDGE('',*,*,#31586,.F.);
#45438=ORIENTED_EDGE('',*,*,#31581,.T.);
#45439=ORIENTED_EDGE('',*,*,#31588,.T.);
#45440=ORIENTED_EDGE('',*,*,#31488,.T.);
#45441=ORIENTED_EDGE('',*,*,#31587,.F.);
#45442=ORIENTED_EDGE('',*,*,#31583,.T.);
#45443=ORIENTED_EDGE('',*,*,#31589,.T.);
#45444=ORIENTED_EDGE('',*,*,#31489,.T.);
#45445=ORIENTED_EDGE('',*,*,#31588,.F.);
#45446=ORIENTED_EDGE('',*,*,#31590,.T.);
#45447=ORIENTED_EDGE('',*,*,#31591,.T.);
#45448=ORIENTED_EDGE('',*,*,#31490,.T.);
#45449=ORIENTED_EDGE('',*,*,#31589,.F.);
#45450=ORIENTED_EDGE('',*,*,#31592,.T.);
#45451=ORIENTED_EDGE('',*,*,#31593,.T.);
#45452=ORIENTED_EDGE('',*,*,#31491,.T.);
#45453=ORIENTED_EDGE('',*,*,#31591,.F.);
#45454=ORIENTED_EDGE('',*,*,#31594,.T.);
#45455=ORIENTED_EDGE('',*,*,#31585,.F.);
#45456=ORIENTED_EDGE('',*,*,#31492,.T.);
#45457=ORIENTED_EDGE('',*,*,#31593,.F.);
#45458=ORIENTED_EDGE('',*,*,#31595,.T.);
#45459=ORIENTED_EDGE('',*,*,#31569,.F.);
#45460=ORIENTED_EDGE('',*,*,#31577,.T.);
#45461=ORIENTED_EDGE('',*,*,#31595,.F.);
#45462=ORIENTED_EDGE('',*,*,#31596,.F.);
#45463=ORIENTED_EDGE('',*,*,#31567,.F.);
#45464=ORIENTED_EDGE('',*,*,#31596,.T.);
#45465=ORIENTED_EDGE('',*,*,#31594,.F.);
#45466=ORIENTED_EDGE('',*,*,#31597,.F.);
#45467=ORIENTED_EDGE('',*,*,#31565,.F.);
#45468=ORIENTED_EDGE('',*,*,#31597,.T.);
#45469=ORIENTED_EDGE('',*,*,#31592,.F.);
#45470=ORIENTED_EDGE('',*,*,#31598,.F.);
#45471=ORIENTED_EDGE('',*,*,#31563,.F.);
#45472=ORIENTED_EDGE('',*,*,#31598,.T.);
#45473=ORIENTED_EDGE('',*,*,#31590,.F.);
#45474=ORIENTED_EDGE('',*,*,#31582,.F.);
#48276=CONICAL_SURFACE('',#54368,4.75,0.785398163397446);
#48277=CONICAL_SURFACE('',#54388,4.75,0.785398163397446);
#48278=CONICAL_SURFACE('',#54398,4.75,0.785398163397446);
#48279=CONICAL_SURFACE('',#54402,4.75,0.785398163397446);
#48280=CONICAL_SURFACE('',#54403,4.75,0.785398163397446);
#48281=CONICAL_SURFACE('',#54407,4.75,0.785398163397446);
#48282=CONICAL_SURFACE('',#54408,4.75,0.785398163397446);
#48283=CONICAL_SURFACE('',#54412,4.75,0.785398163397446);
#48284=CONICAL_SURFACE('',#54413,1.5,1.02974425867665);
#48285=CONICAL_SURFACE('',#54416,1.5,1.02974425867665);
#48286=CONICAL_SURFACE('',#54419,1.525,1.02974425867665);
#48287=CONICAL_SURFACE('',#54421,3.175,0.785398163397448);
#48288=CONICAL_SURFACE('',#54424,1.525,1.02974425867665);
#48289=CONICAL_SURFACE('',#54426,3.175,0.785398163397448);
#48290=CONICAL_SURFACE('',#54429,1.525,1.02974425867665);
#48291=CONICAL_SURFACE('',#54431,3.175,0.785398163397448);
#48292=CONICAL_SURFACE('',#54434,1.525,1.02974425867665);
#48293=CONICAL_SURFACE('',#54436,3.175,0.785398163397448);
#48294=CONICAL_SURFACE('',#54442,9.75,0.785398163397447);
#48295=CONICAL_SURFACE('',#54445,9.75,0.785398163397447);
#48296=CONICAL_SURFACE('',#54448,9.75,0.785398163397447);
#48297=CONICAL_SURFACE('',#54451,9.75,0.785398163397447);
#48298=CONICAL_SURFACE('',#54461,9.5,0.785398163397447);
#48299=CONICAL_SURFACE('',#54463,9.5,0.785398163397447);
#48300=CONICAL_SURFACE('',#54465,9.5,0.785398163397447);
#48301=CONICAL_SURFACE('',#54468,9.5,0.785398163397447);
#50120=ADVANCED_FACE('',(#15033),#12735,.F.);
#50121=ADVANCED_FACE('',(#15034),#12736,.F.);
#50122=ADVANCED_FACE('',(#15035),#12737,.F.);
#50123=ADVANCED_FACE('',(#15036),#12738,.F.);
#50124=ADVANCED_FACE('',(#15037),#12739,.F.);
#50125=ADVANCED_FACE('',(#15038),#12740,.F.);
#50126=ADVANCED_FACE('',(#15039),#12741,.F.);
#50127=ADVANCED_FACE('',(#15040),#12742,.F.);
#50128=ADVANCED_FACE('',(#15041),#12743,.F.);
#50129=ADVANCED_FACE('',(#15042),#12744,.F.);
#50130=ADVANCED_FACE('',(#15043),#12745,.F.);
#50131=ADVANCED_FACE('',(#15044),#12746,.F.);
#50132=ADVANCED_FACE('',(#15045),#12747,.F.);
#50133=ADVANCED_FACE('',(#15046),#12748,.F.);
#50134=ADVANCED_FACE('',(#15047),#12749,.F.);
#50135=ADVANCED_FACE('',(#15048),#12750,.F.);
#50136=ADVANCED_FACE('',(#15049),#12751,.F.);
#50137=ADVANCED_FACE('',(#15050),#12752,.F.);
#50138=ADVANCED_FACE('',(#15051),#719,.F.);
#50139=ADVANCED_FACE('',(#15052),#720,.F.);
#50140=ADVANCED_FACE('',(#15053),#721,.F.);
#50141=ADVANCED_FACE('',(#15054),#722,.F.);
#50142=ADVANCED_FACE('',(#15055),#723,.F.);
#50143=ADVANCED_FACE('',(#15056),#724,.F.);
#50144=ADVANCED_FACE('',(#15057),#725,.F.);
#50145=ADVANCED_FACE('',(#15058),#726,.F.);
#50146=ADVANCED_FACE('',(#15059),#727,.F.);
#50147=ADVANCED_FACE('',(#15060),#728,.F.);
#50148=ADVANCED_FACE('',(#15061),#729,.F.);
#50149=ADVANCED_FACE('',(#15062),#730,.F.);
#50150=ADVANCED_FACE('',(#15063),#731,.F.);
#50151=ADVANCED_FACE('',(#15064),#12753,.F.);
#50152=ADVANCED_FACE('',(#15065),#732,.F.);
#50153=ADVANCED_FACE('',(#15066),#733,.F.);
#50154=ADVANCED_FACE('',(#15067),#734,.F.);
#50155=ADVANCED_FACE('',(#15068),#735,.F.);
#50156=ADVANCED_FACE('',(#15069),#736,.F.);
#50157=ADVANCED_FACE('',(#15070),#737,.F.);
#50158=ADVANCED_FACE('',(#15071),#738,.F.);
#50159=ADVANCED_FACE('',(#15072),#739,.F.);
#50160=ADVANCED_FACE('',(#15073),#740,.F.);
#50161=ADVANCED_FACE('',(#15074),#741,.F.);
#50162=ADVANCED_FACE('',(#15075),#742,.F.);
#50163=ADVANCED_FACE('',(#15076),#743,.F.);
#50164=ADVANCED_FACE('',(#15077),#744,.F.);
#50165=ADVANCED_FACE('',(#15078),#745,.F.);
#50166=ADVANCED_FACE('',(#15079),#746,.F.);
#50167=ADVANCED_FACE('',(#15080),#747,.F.);
#50168=ADVANCED_FACE('',(#15081),#748,.F.);
#50169=ADVANCED_FACE('',(#15082),#749,.F.);
#50170=ADVANCED_FACE('',(#15083),#12754,.F.);
#50171=ADVANCED_FACE('',(#15084),#750,.F.);
#50172=ADVANCED_FACE('',(#15085),#751,.F.);
#50173=ADVANCED_FACE('',(#15086),#12755,.T.);
#50174=ADVANCED_FACE('',(#15087),#752,.F.);
#50175=ADVANCED_FACE('',(#15088),#753,.F.);
#50176=ADVANCED_FACE('',(#15089),#754,.F.);
#50177=ADVANCED_FACE('',(#15090),#755,.F.);
#50178=ADVANCED_FACE('',(#15091),#756,.F.);
#50179=ADVANCED_FACE('',(#15092),#757,.F.);
#50180=ADVANCED_FACE('',(#15093),#758,.F.);
#50181=ADVANCED_FACE('',(#15094),#759,.F.);
#50182=ADVANCED_FACE('',(#15095),#12756,.F.);
#50183=ADVANCED_FACE('',(#15096),#760,.F.);
#50184=ADVANCED_FACE('',(#15097),#761,.F.);
#50185=ADVANCED_FACE('',(#15098),#762,.F.);
#50186=ADVANCED_FACE('',(#15099),#763,.F.);
#50187=ADVANCED_FACE('',(#15100),#764,.F.);
#50188=ADVANCED_FACE('',(#15101),#765,.F.);
#50189=ADVANCED_FACE('',(#15102),#766,.F.);
#50190=ADVANCED_FACE('',(#15103),#767,.F.);
#50191=ADVANCED_FACE('',(#15104),#768,.F.);
#50192=ADVANCED_FACE('',(#15105),#769,.F.);
#50193=ADVANCED_FACE('',(#15106),#12757,.F.);
#50194=ADVANCED_FACE('',(#15107),#770,.F.);
#50195=ADVANCED_FACE('',(#15108),#771,.F.);
#50196=ADVANCED_FACE('',(#15109),#12758,.T.);
#50197=ADVANCED_FACE('',(#15110),#12759,.F.);
#50198=ADVANCED_FACE('',(#15111),#12760,.F.);
#50199=ADVANCED_FACE('',(#15112),#12761,.F.);
#50200=ADVANCED_FACE('',(#15113),#12762,.F.);
#50201=ADVANCED_FACE('',(#15114),#12763,.F.);
#50202=ADVANCED_FACE('',(#15115),#12764,.F.);
#50203=ADVANCED_FACE('',(#15116),#12765,.F.);
#50204=ADVANCED_FACE('',(#15117),#12766,.F.);
#50205=ADVANCED_FACE('',(#15118),#12767,.F.);
#50206=ADVANCED_FACE('',(#15119),#12768,.F.);
#50207=ADVANCED_FACE('',(#15120),#12769,.F.);
#50208=ADVANCED_FACE('',(#15121),#12770,.F.);
#50209=ADVANCED_FACE('',(#15122),#12771,.F.);
#50210=ADVANCED_FACE('',(#15123),#12772,.F.);
#50211=ADVANCED_FACE('',(#15124),#12773,.F.);
#50212=ADVANCED_FACE('',(#15125),#12774,.F.);
#50213=ADVANCED_FACE('',(#15126),#772,.F.);
#50214=ADVANCED_FACE('',(#15127),#773,.F.);
#50215=ADVANCED_FACE('',(#15128),#774,.F.);
#50216=ADVANCED_FACE('',(#15129),#775,.F.);
#50217=ADVANCED_FACE('',(#15130),#12775,.F.);
#50218=ADVANCED_FACE('',(#15131),#12776,.F.);
#50219=ADVANCED_FACE('',(#15132),#12777,.F.);
#50220=ADVANCED_FACE('',(#15133),#776,.F.);
#50221=ADVANCED_FACE('',(#15134),#777,.F.);
#50222=ADVANCED_FACE('',(#15135),#778,.F.);
#50223=ADVANCED_FACE('',(#15136),#779,.F.);
#50224=ADVANCED_FACE('',(#15137),#780,.F.);
#50225=ADVANCED_FACE('',(#15138),#781,.F.);
#50226=ADVANCED_FACE('',(#15139),#12778,.F.);
#50227=ADVANCED_FACE('',(#15140),#12779,.F.);
#50228=ADVANCED_FACE('',(#15141),#12780,.F.);
#50229=ADVANCED_FACE('',(#15142),#782,.F.);
#50230=ADVANCED_FACE('',(#15143),#12781,.T.);
#50231=ADVANCED_FACE('',(#15144),#12782,.F.);
#50232=ADVANCED_FACE('',(#15145),#783,.F.);
#50233=ADVANCED_FACE('',(#15146),#784,.F.);
#50234=ADVANCED_FACE('',(#15147),#785,.F.);
#50235=ADVANCED_FACE('',(#15148),#786,.F.);
#50236=ADVANCED_FACE('',(#15149),#12783,.F.);
#50237=ADVANCED_FACE('',(#15150),#12784,.F.);
#50238=ADVANCED_FACE('',(#15151),#12785,.F.);
#50239=ADVANCED_FACE('',(#15152),#787,.F.);
#50240=ADVANCED_FACE('',(#15153),#788,.F.);
#50241=ADVANCED_FACE('',(#15154),#789,.F.);
#50242=ADVANCED_FACE('',(#15155),#790,.F.);
#50243=ADVANCED_FACE('',(#15156),#791,.F.);
#50244=ADVANCED_FACE('',(#15157),#792,.F.);
#50245=ADVANCED_FACE('',(#15158),#793,.F.);
#50246=ADVANCED_FACE('',(#15159),#12786,.F.);
#50247=ADVANCED_FACE('',(#15160),#12787,.F.);
#50248=ADVANCED_FACE('',(#15161),#12788,.F.);
#50249=ADVANCED_FACE('',(#15162),#12789,.F.);
#50250=ADVANCED_FACE('',(#15163),#12790,.T.);
#50251=ADVANCED_FACE('',(#15164),#12791,.F.);
#50252=ADVANCED_FACE('',(#15165),#12792,.F.);
#50253=ADVANCED_FACE('',(#15166),#12793,.F.);
#50254=ADVANCED_FACE('',(#15167),#12794,.F.);
#50255=ADVANCED_FACE('',(#15168),#12795,.F.);
#50256=ADVANCED_FACE('',(#15169),#12796,.F.);
#50257=ADVANCED_FACE('',(#15170),#12797,.F.);
#50258=ADVANCED_FACE('',(#15171),#12798,.F.);
#50259=ADVANCED_FACE('',(#15172),#12799,.F.);
#50260=ADVANCED_FACE('',(#15173),#794,.F.);
#50261=ADVANCED_FACE('',(#15174),#795,.F.);
#50262=ADVANCED_FACE('',(#15175),#12800,.F.);
#50263=ADVANCED_FACE('',(#15176),#796,.F.);
#50264=ADVANCED_FACE('',(#15177),#797,.F.);
#50265=ADVANCED_FACE('',(#15178),#12801,.F.);
#50266=ADVANCED_FACE('',(#15179),#12802,.F.);
#50267=ADVANCED_FACE('',(#15180),#12803,.F.);
#50268=ADVANCED_FACE('',(#15181),#12804,.F.);
#50269=ADVANCED_FACE('',(#15182),#12805,.T.);
#50270=ADVANCED_FACE('',(#15183),#798,.F.);
#50271=ADVANCED_FACE('',(#15184),#799,.F.);
#50272=ADVANCED_FACE('',(#15185),#800,.F.);
#50273=ADVANCED_FACE('',(#15186),#801,.F.);
#50274=ADVANCED_FACE('',(#15187),#802,.F.);
#50275=ADVANCED_FACE('',(#15188),#803,.F.);
#50276=ADVANCED_FACE('',(#15189),#804,.F.);
#50277=ADVANCED_FACE('',(#15190),#805,.F.);
#50278=ADVANCED_FACE('',(#15191),#806,.F.);
#50279=ADVANCED_FACE('',(#15192),#807,.F.);
#50280=ADVANCED_FACE('',(#15193),#808,.F.);
#50281=ADVANCED_FACE('',(#15194),#809,.F.);
#50282=ADVANCED_FACE('',(#15195),#12806,.T.);
#50283=ADVANCED_FACE('',(#15196),#810,.F.);
#50284=ADVANCED_FACE('',(#15197),#811,.F.);
#50285=ADVANCED_FACE('',(#15198),#12807,.F.);
#50286=ADVANCED_FACE('',(#15199),#812,.F.);
#50287=ADVANCED_FACE('',(#15200),#813,.F.);
#50288=ADVANCED_FACE('',(#15201),#12808,.F.);
#50289=ADVANCED_FACE('',(#15202),#12809,.F.);
#50290=ADVANCED_FACE('',(#15203),#12810,.F.);
#50291=ADVANCED_FACE('',(#15204),#12811,.F.);
#50292=ADVANCED_FACE('',(#15205),#12812,.T.);
#50293=ADVANCED_FACE('',(#15206),#12813,.F.);
#50294=ADVANCED_FACE('',(#15207),#12814,.F.);
#50295=ADVANCED_FACE('',(#15208),#12815,.F.);
#50296=ADVANCED_FACE('',(#15209),#12816,.F.);
#50297=ADVANCED_FACE('',(#15210),#12817,.F.);
#50298=ADVANCED_FACE('',(#15211),#814,.F.);
#50299=ADVANCED_FACE('',(#15212),#815,.F.);
#50300=ADVANCED_FACE('',(#15213),#816,.F.);
#50301=ADVANCED_FACE('',(#15214),#817,.F.);
#50302=ADVANCED_FACE('',(#15215),#818,.F.);
#50303=ADVANCED_FACE('',(#15216),#12818,.F.);
#50304=ADVANCED_FACE('',(#15217),#12819,.F.);
#50305=ADVANCED_FACE('',(#15218),#12820,.F.);
#50306=ADVANCED_FACE('',(#15219),#12821,.F.);
#50307=ADVANCED_FACE('',(#15220),#12822,.F.);
#50308=ADVANCED_FACE('',(#15221),#12823,.F.);
#50309=ADVANCED_FACE('',(#15222),#819,.F.);
#50310=ADVANCED_FACE('',(#15223),#820,.F.);
#50311=ADVANCED_FACE('',(#15224),#821,.F.);
#50312=ADVANCED_FACE('',(#15225),#822,.F.);
#50313=ADVANCED_FACE('',(#15226),#823,.F.);
#50314=ADVANCED_FACE('',(#15227),#824,.F.);
#50315=ADVANCED_FACE('',(#15228),#825,.F.);
#50316=ADVANCED_FACE('',(#15229),#826,.F.);
#50317=ADVANCED_FACE('',(#15230),#12824,.F.);
#50318=ADVANCED_FACE('',(#15231),#827,.F.);
#50319=ADVANCED_FACE('',(#15232),#828,.F.);
#50320=ADVANCED_FACE('',(#15233),#12825,.T.);
#50321=ADVANCED_FACE('',(#15234),#829,.F.);
#50322=ADVANCED_FACE('',(#15235),#830,.F.);
#50323=ADVANCED_FACE('',(#15236),#831,.F.);
#50324=ADVANCED_FACE('',(#15237),#832,.F.);
#50325=ADVANCED_FACE('',(#15238),#833,.F.);
#50326=ADVANCED_FACE('',(#15239),#834,.F.);
#50327=ADVANCED_FACE('',(#15240),#835,.F.);
#50328=ADVANCED_FACE('',(#15241),#836,.F.);
#50329=ADVANCED_FACE('',(#15242),#837,.F.);
#50330=ADVANCED_FACE('',(#15243),#838,.F.);
#50331=ADVANCED_FACE('',(#15244),#839,.F.);
#50332=ADVANCED_FACE('',(#15245),#12826,.T.);
#50333=ADVANCED_FACE('',(#15246),#840,.F.);
#50334=ADVANCED_FACE('',(#15247),#841,.F.);
#50335=ADVANCED_FACE('',(#15248),#842,.F.);
#50336=ADVANCED_FACE('',(#15249),#843,.F.);
#50337=ADVANCED_FACE('',(#15250),#844,.F.);
#50338=ADVANCED_FACE('',(#15251),#845,.F.);
#50339=ADVANCED_FACE('',(#15252),#846,.F.);
#50340=ADVANCED_FACE('',(#15253),#847,.F.);
#50341=ADVANCED_FACE('',(#15254),#848,.F.);
#50342=ADVANCED_FACE('',(#15255),#849,.F.);
#50343=ADVANCED_FACE('',(#15256),#850,.F.);
#50344=ADVANCED_FACE('',(#15257),#12827,.F.);
#50345=ADVANCED_FACE('',(#15258),#851,.F.);
#50346=ADVANCED_FACE('',(#15259),#852,.F.);
#50347=ADVANCED_FACE('',(#15260),#853,.F.);
#50348=ADVANCED_FACE('',(#15261),#12828,.T.);
#50349=ADVANCED_FACE('',(#15262),#12829,.F.);
#50350=ADVANCED_FACE('',(#15263),#12830,.F.);
#50351=ADVANCED_FACE('',(#15264),#12831,.F.);
#50352=ADVANCED_FACE('',(#15265),#12832,.F.);
#50353=ADVANCED_FACE('',(#15266),#12833,.F.);
#50354=ADVANCED_FACE('',(#15267),#12834,.F.);
#50355=ADVANCED_FACE('',(#15268),#12835,.F.);
#50356=ADVANCED_FACE('',(#15269),#12836,.F.);
#50357=ADVANCED_FACE('',(#15270),#12837,.F.);
#50358=ADVANCED_FACE('',(#15271),#12838,.F.);
#50359=ADVANCED_FACE('',(#15272),#12839,.F.);
#50360=ADVANCED_FACE('',(#15273),#12840,.F.);
#50361=ADVANCED_FACE('',(#15274),#12841,.F.);
#50362=ADVANCED_FACE('',(#15275),#12842,.F.);
#50363=ADVANCED_FACE('',(#15276),#12843,.F.);
#50364=ADVANCED_FACE('',(#15277),#12844,.F.);
#50365=ADVANCED_FACE('',(#15278),#12845,.F.);
#50366=ADVANCED_FACE('',(#15279),#12846,.F.);
#50367=ADVANCED_FACE('',(#15280),#854,.F.);
#50368=ADVANCED_FACE('',(#15281),#855,.F.);
#50369=ADVANCED_FACE('',(#15282),#856,.F.);
#50370=ADVANCED_FACE('',(#15283),#857,.F.);
#50371=ADVANCED_FACE('',(#15284),#858,.F.);
#50372=ADVANCED_FACE('',(#15285),#859,.F.);
#50373=ADVANCED_FACE('',(#15286),#860,.F.);
#50374=ADVANCED_FACE('',(#15287),#861,.F.);
#50375=ADVANCED_FACE('',(#15288),#862,.F.);
#50376=ADVANCED_FACE('',(#15289),#863,.F.);
#50377=ADVANCED_FACE('',(#15290),#864,.F.);
#50378=ADVANCED_FACE('',(#15291),#12847,.T.);
#50379=ADVANCED_FACE('',(#15292),#12848,.F.);
#50380=ADVANCED_FACE('',(#15293),#12849,.F.);
#50381=ADVANCED_FACE('',(#15294),#12850,.F.);
#50382=ADVANCED_FACE('',(#15295),#12851,.F.);
#50383=ADVANCED_FACE('',(#15296),#12852,.F.);
#50384=ADVANCED_FACE('',(#15297),#12853,.F.);
#50385=ADVANCED_FACE('',(#15298),#12854,.F.);
#50386=ADVANCED_FACE('',(#15299),#12855,.F.);
#50387=ADVANCED_FACE('',(#15300),#12856,.F.);
#50388=ADVANCED_FACE('',(#15301),#12857,.F.);
#50389=ADVANCED_FACE('',(#15302),#12858,.F.);
#50390=ADVANCED_FACE('',(#15303),#12859,.F.);
#50391=ADVANCED_FACE('',(#15304),#12860,.F.);
#50392=ADVANCED_FACE('',(#15305),#12861,.F.);
#50393=ADVANCED_FACE('',(#15306),#12862,.F.);
#50394=ADVANCED_FACE('',(#15307),#12863,.F.);
#50395=ADVANCED_FACE('',(#15308),#12864,.F.);
#50396=ADVANCED_FACE('',(#15309),#12865,.F.);
#50397=ADVANCED_FACE('',(#15310),#12866,.F.);
#50398=ADVANCED_FACE('',(#15311),#12867,.F.);
#50399=ADVANCED_FACE('',(#15312),#865,.F.);
#50400=ADVANCED_FACE('',(#15313),#866,.F.);
#50401=ADVANCED_FACE('',(#15314),#867,.F.);
#50402=ADVANCED_FACE('',(#15315),#868,.F.);
#50403=ADVANCED_FACE('',(#15316),#869,.F.);
#50404=ADVANCED_FACE('',(#15317),#870,.F.);
#50405=ADVANCED_FACE('',(#15318),#871,.F.);
#50406=ADVANCED_FACE('',(#15319),#872,.F.);
#50407=ADVANCED_FACE('',(#15320),#12868,.F.);
#50408=ADVANCED_FACE('',(#15321),#12869,.F.);
#50409=ADVANCED_FACE('',(#15322),#12870,.F.);
#50410=ADVANCED_FACE('',(#15323),#873,.F.);
#50411=ADVANCED_FACE('',(#15324),#12871,.T.);
#50412=ADVANCED_FACE('',(#15325),#12872,.F.);
#50413=ADVANCED_FACE('',(#15326),#874,.F.);
#50414=ADVANCED_FACE('',(#15327),#875,.F.);
#50415=ADVANCED_FACE('',(#15328),#876,.F.);
#50416=ADVANCED_FACE('',(#15329),#877,.F.);
#50417=ADVANCED_FACE('',(#15330),#12873,.F.);
#50418=ADVANCED_FACE('',(#15331),#12874,.F.);
#50419=ADVANCED_FACE('',(#15332),#12875,.F.);
#50420=ADVANCED_FACE('',(#15333),#878,.F.);
#50421=ADVANCED_FACE('',(#15334),#879,.F.);
#50422=ADVANCED_FACE('',(#15335),#880,.F.);
#50423=ADVANCED_FACE('',(#15336),#881,.F.);
#50424=ADVANCED_FACE('',(#15337),#882,.F.);
#50425=ADVANCED_FACE('',(#15338),#883,.F.);
#50426=ADVANCED_FACE('',(#15339),#884,.F.);
#50427=ADVANCED_FACE('',(#15340),#12876,.F.);
#50428=ADVANCED_FACE('',(#15341),#12877,.F.);
#50429=ADVANCED_FACE('',(#15342),#12878,.F.);
#50430=ADVANCED_FACE('',(#15343),#12879,.F.);
#50431=ADVANCED_FACE('',(#15344),#12880,.T.);
#50432=ADVANCED_FACE('',(#15345),#12881,.F.);
#50433=ADVANCED_FACE('',(#15346),#12882,.F.);
#50434=ADVANCED_FACE('',(#15347),#12883,.F.);
#50435=ADVANCED_FACE('',(#15348),#12884,.F.);
#50436=ADVANCED_FACE('',(#15349,#989,#990,#991,#992,#993,#994,#995,#996,
#997,#998,#999,#1000,#1001,#1002,#1003,#1004,#1005,#1006,#1007,#1008,#1009,
#1010,#1011),#12885,.T.);
#50437=ADVANCED_FACE('',(#15350),#48276,.F.);
#50438=ADVANCED_FACE('',(#15351),#1140,.F.);
#50439=ADVANCED_FACE('',(#15352,#1012,#1013,#1014,#1015,#1016,#1017,#1018,
#1019,#1020,#1021,#1022,#1023),#12886,.T.);
#50440=ADVANCED_FACE('',(#15353),#48277,.F.);
#50441=ADVANCED_FACE('',(#15354,#1024,#1025,#1026,#1027),#12887,.F.);
#50442=ADVANCED_FACE('',(#15355),#48278,.F.);
#50443=ADVANCED_FACE('',(#15356),#1141,.F.);
#50444=ADVANCED_FACE('',(#15357),#48279,.F.);
#50445=ADVANCED_FACE('',(#15358),#48280,.F.);
#50446=ADVANCED_FACE('',(#15359),#1142,.F.);
#50447=ADVANCED_FACE('',(#15360),#48281,.F.);
#50448=ADVANCED_FACE('',(#15361),#48282,.F.);
#50449=ADVANCED_FACE('',(#15362),#1143,.F.);
#50450=ADVANCED_FACE('',(#15363),#48283,.F.);
#50451=ADVANCED_FACE('',(#15364),#48284,.F.);
#50452=ADVANCED_FACE('',(#15365),#1144,.F.);
#50453=ADVANCED_FACE('',(#15366),#48285,.F.);
#50454=ADVANCED_FACE('',(#15367),#1145,.F.);
#50455=ADVANCED_FACE('',(#15368),#48286,.F.);
#50456=ADVANCED_FACE('',(#15369),#48287,.F.);
#50457=ADVANCED_FACE('',(#15370),#1146,.F.);
#50458=ADVANCED_FACE('',(#15371),#48288,.F.);
#50459=ADVANCED_FACE('',(#15372),#48289,.F.);
#50460=ADVANCED_FACE('',(#15373),#1147,.F.);
#50461=ADVANCED_FACE('',(#15374),#48290,.F.);
#50462=ADVANCED_FACE('',(#15375),#48291,.F.);
#50463=ADVANCED_FACE('',(#15376),#1148,.F.);
#50464=ADVANCED_FACE('',(#15377),#48292,.F.);
#50465=ADVANCED_FACE('',(#15378),#48293,.F.);
#50466=ADVANCED_FACE('',(#15379),#1149,.F.);
#50467=ADVANCED_FACE('',(#15380),#1150,.F.);
#50468=ADVANCED_FACE('',(#15381),#12888,.T.);
#50469=ADVANCED_FACE('',(#15382),#48294,.T.);
#50470=ADVANCED_FACE('',(#15383),#12889,.T.);
#50471=ADVANCED_FACE('',(#15384),#48295,.T.);
#50472=ADVANCED_FACE('',(#15385),#12890,.T.);
#50473=ADVANCED_FACE('',(#15386),#48296,.T.);
#50474=ADVANCED_FACE('',(#15387),#12891,.T.);
#50475=ADVANCED_FACE('',(#15388),#48297,.T.);
#50476=ADVANCED_FACE('',(#15389),#12892,.T.);
#50477=ADVANCED_FACE('',(#15390),#12893,.T.);
#50478=ADVANCED_FACE('',(#15391),#1151,.T.);
#50479=ADVANCED_FACE('',(#15392),#12894,.T.);
#50480=ADVANCED_FACE('',(#15393),#1152,.T.);
#50481=ADVANCED_FACE('',(#15394),#12895,.T.);
#50482=ADVANCED_FACE('',(#15395),#48298,.T.);
#50483=ADVANCED_FACE('',(#15396),#12896,.T.);
#50484=ADVANCED_FACE('',(#15397),#48299,.T.);
#50485=ADVANCED_FACE('',(#15398),#12897,.T.);
#50486=ADVANCED_FACE('',(#15399),#48300,.T.);
#50487=ADVANCED_FACE('',(#15400),#12898,.T.);
#50488=ADVANCED_FACE('',(#15401),#48301,.T.);
#50489=ADVANCED_FACE('',(#15402),#1153,.T.);
#50490=ADVANCED_FACE('',(#15403),#12899,.T.);
#50491=ADVANCED_FACE('',(#15404),#1154,.T.);
#50492=ADVANCED_FACE('',(#15405),#12900,.T.);
#51021=CLOSED_SHELL('',(#50120,#50121,#50122,#50123,#50124,#50125,#50126,
#50127,#50128,#50129,#50130,#50131,#50132,#50133,#50134,#50135,#50136,#50137,
#50138,#50139,#50140,#50141,#50142,#50143,#50144,#50145,#50146,#50147,#50148,
#50149,#50150,#50151,#50152,#50153,#50154,#50155,#50156,#50157,#50158,#50159,
#50160,#50161,#50162,#50163,#50164,#50165,#50166,#50167,#50168,#50169,#50170,
#50171,#50172,#50173,#50174,#50175,#50176,#50177,#50178,#50179,#50180,#50181,
#50182,#50183,#50184,#50185,#50186,#50187,#50188,#50189,#50190,#50191,#50192,
#50193,#50194,#50195,#50196,#50197,#50198,#50199,#50200,#50201,#50202,#50203,
#50204,#50205,#50206,#50207,#50208,#50209,#50210,#50211,#50212,#50213,#50214,
#50215,#50216,#50217,#50218,#50219,#50220,#50221,#50222,#50223,#50224,#50225,
#50226,#50227,#50228,#50229,#50230,#50231,#50232,#50233,#50234,#50235,#50236,
#50237,#50238,#50239,#50240,#50241,#50242,#50243,#50244,#50245,#50246,#50247,
#50248,#50249,#50250,#50251,#50252,#50253,#50254,#50255,#50256,#50257,#50258,
#50259,#50260,#50261,#50262,#50263,#50264,#50265,#50266,#50267,#50268,#50269,
#50270,#50271,#50272,#50273,#50274,#50275,#50276,#50277,#50278,#50279,#50280,
#50281,#50282,#50283,#50284,#50285,#50286,#50287,#50288,#50289,#50290,#50291,
#50292,#50293,#50294,#50295,#50296,#50297,#50298,#50299,#50300,#50301,#50302,
#50303,#50304,#50305,#50306,#50307,#50308,#50309,#50310,#50311,#50312,#50313,
#50314,#50315,#50316,#50317,#50318,#50319,#50320,#50321,#50322,#50323,#50324,
#50325,#50326,#50327,#50328,#50329,#50330,#50331,#50332,#50333,#50334,#50335,
#50336,#50337,#50338,#50339,#50340,#50341,#50342,#50343,#50344,#50345,#50346,
#50347,#50348,#50349,#50350,#50351,#50352,#50353,#50354,#50355,#50356,#50357,
#50358,#50359,#50360,#50361,#50362,#50363,#50364,#50365,#50366,#50367,#50368,
#50369,#50370,#50371,#50372,#50373,#50374,#50375,#50376,#50377,#50378,#50379,
#50380,#50381,#50382,#50383,#50384,#50385,#50386,#50387,#50388,#50389,#50390,
#50391,#50392,#50393,#50394,#50395,#50396,#50397,#50398,#50399,#50400,#50401,
#50402,#50403,#50404,#50405,#50406,#50407,#50408,#50409,#50410,#50411,#50412,
#50413,#50414,#50415,#50416,#50417,#50418,#50419,#50420,#50421,#50422,#50423,
#50424,#50425,#50426,#50427,#50428,#50429,#50430,#50431,#50432,#50433,#50434,
#50435,#50436,#50437,#50438,#50439,#50440,#50441,#50442,#50443,#50444,#50445,
#50446,#50447,#50448,#50449,#50450,#50451,#50452,#50453,#50454,#50455,#50456,
#50457,#50458,#50459,#50460,#50461,#50462,#50463,#50464,#50465,#50466,#50467,
#50468,#50469,#50470,#50471,#50472,#50473,#50474,#50475,#50476,#50477,#50478,
#50479,#50480,#50481,#50482,#50483,#50484,#50485,#50486,#50487,#50488,#50489,
#50490,#50491,#50492));
#54216=AXIS2_PLACEMENT_3D('',#80526,#64623,#64624);
#54217=AXIS2_PLACEMENT_3D('',#80527,#64625,#64626);
#54218=AXIS2_PLACEMENT_3D('',#80536,#64631,#64632);
#54219=AXIS2_PLACEMENT_3D('',#80542,#64636,#64637);
#54220=AXIS2_PLACEMENT_3D('',#80548,#64641,#64642);
#54221=AXIS2_PLACEMENT_3D('',#80554,#64646,#64647);
#54222=AXIS2_PLACEMENT_3D('',#80560,#64651,#64652);
#54223=AXIS2_PLACEMENT_3D('',#80566,#64656,#64657);
#54224=AXIS2_PLACEMENT_3D('',#80572,#64661,#64662);
#54225=AXIS2_PLACEMENT_3D('',#80578,#64666,#64667);
#54226=AXIS2_PLACEMENT_3D('',#80584,#64671,#64672);
#54227=AXIS2_PLACEMENT_3D('',#80590,#64676,#64677);
#54228=AXIS2_PLACEMENT_3D('',#80596,#64681,#64682);
#54229=AXIS2_PLACEMENT_3D('',#80599,#64685,#64686);
#54230=AXIS2_PLACEMENT_3D('',#80600,#64687,#64688);
#54231=AXIS2_PLACEMENT_3D('',#80609,#64693,#64694);
#54232=AXIS2_PLACEMENT_3D('',#80615,#64698,#64699);
#54233=AXIS2_PLACEMENT_3D('',#80621,#64703,#64704);
#54234=AXIS2_PLACEMENT_3D('',#80624,#64707,#64708);
#54235=AXIS2_PLACEMENT_3D('',#80823,#64723,#64724);
#54236=AXIS2_PLACEMENT_3D('',#81099,#64746,#64747);
#54237=AXIS2_PLACEMENT_3D('',#81132,#64752,#64753);
#54238=AXIS2_PLACEMENT_3D('',#81256,#64763,#64764);
#54239=AXIS2_PLACEMENT_3D('',#81412,#64778,#64779);
#54240=AXIS2_PLACEMENT_3D('',#81445,#64784,#64785);
#54241=AXIS2_PLACEMENT_3D('',#81446,#64786,#64787);
#54242=AXIS2_PLACEMENT_3D('',#81455,#64792,#64793);
#54243=AXIS2_PLACEMENT_3D('',#81461,#64797,#64798);
#54244=AXIS2_PLACEMENT_3D('',#81467,#64802,#64803);
#54245=AXIS2_PLACEMENT_3D('',#81473,#64807,#64808);
#54246=AXIS2_PLACEMENT_3D('',#81479,#64812,#64813);
#54247=AXIS2_PLACEMENT_3D('',#81482,#64816,#64817);
#54248=AXIS2_PLACEMENT_3D('',#81483,#64818,#64819);
#54249=AXIS2_PLACEMENT_3D('',#81492,#64824,#64825);
#54250=AXIS2_PLACEMENT_3D('',#81498,#64829,#64830);
#54251=AXIS2_PLACEMENT_3D('',#81504,#64834,#64835);
#54252=AXIS2_PLACEMENT_3D('',#81510,#64839,#64840);
#54253=AXIS2_PLACEMENT_3D('',#81516,#64844,#64845);
#54254=AXIS2_PLACEMENT_3D('',#81522,#64849,#64850);
#54255=AXIS2_PLACEMENT_3D('',#81528,#64854,#64855);
#54256=AXIS2_PLACEMENT_3D('',#81531,#64858,#64859);
#54257=AXIS2_PLACEMENT_3D('',#81595,#64865,#64866);
#54258=AXIS2_PLACEMENT_3D('',#81601,#64870,#64871);
#54259=AXIS2_PLACEMENT_3D('',#81607,#64875,#64876);
#54260=AXIS2_PLACEMENT_3D('',#81703,#64886,#64887);
#54261=AXIS2_PLACEMENT_3D('',#81709,#64891,#64892);
#54262=AXIS2_PLACEMENT_3D('',#81715,#64896,#64897);
#54263=AXIS2_PLACEMENT_3D('',#81733,#64901,#64902);
#54264=AXIS2_PLACEMENT_3D('',#81734,#64903,#64904);
#54265=AXIS2_PLACEMENT_3D('',#81803,#64913,#64914);
#54266=AXIS2_PLACEMENT_3D('',#81809,#64918,#64919);
#54267=AXIS2_PLACEMENT_3D('',#81815,#64923,#64924);
#54268=AXIS2_PLACEMENT_3D('',#81926,#64935,#64936);
#54269=AXIS2_PLACEMENT_3D('',#81932,#64940,#64941);
#54270=AXIS2_PLACEMENT_3D('',#81938,#64945,#64946);
#54271=AXIS2_PLACEMENT_3D('',#81944,#64950,#64951);
#54272=AXIS2_PLACEMENT_3D('',#81947,#64954,#64955);
#54273=AXIS2_PLACEMENT_3D('',#81948,#64956,#64957);
#54274=AXIS2_PLACEMENT_3D('',#81957,#64962,#64963);
#54275=AXIS2_PLACEMENT_3D('',#81963,#64967,#64968);
#54276=AXIS2_PLACEMENT_3D('',#81969,#64972,#64973);
#54277=AXIS2_PLACEMENT_3D('',#81975,#64977,#64978);
#54278=AXIS2_PLACEMENT_3D('',#81981,#64982,#64983);
#54279=AXIS2_PLACEMENT_3D('',#81987,#64987,#64988);
#54280=AXIS2_PLACEMENT_3D('',#81993,#64992,#64993);
#54281=AXIS2_PLACEMENT_3D('',#81996,#64996,#64997);
#54282=AXIS2_PLACEMENT_3D('',#82030,#65001,#65002);
#54283=AXIS2_PLACEMENT_3D('',#82066,#65008,#65009);
#54284=AXIS2_PLACEMENT_3D('',#82072,#65013,#65014);
#54285=AXIS2_PLACEMENT_3D('',#82078,#65018,#65019);
#54286=AXIS2_PLACEMENT_3D('',#82084,#65023,#65024);
#54287=AXIS2_PLACEMENT_3D('',#82087,#65027,#65028);
#54288=AXIS2_PLACEMENT_3D('',#82268,#65041,#65042);
#54289=AXIS2_PLACEMENT_3D('',#82302,#65046,#65047);
#54290=AXIS2_PLACEMENT_3D('',#82338,#65053,#65054);
#54291=AXIS2_PLACEMENT_3D('',#82344,#65058,#65059);
#54292=AXIS2_PLACEMENT_3D('',#82350,#65063,#65064);
#54293=AXIS2_PLACEMENT_3D('',#82356,#65068,#65069);
#54294=AXIS2_PLACEMENT_3D('',#82359,#65072,#65073);
#54295=AXIS2_PLACEMENT_3D('',#82360,#65074,#65075);
#54296=AXIS2_PLACEMENT_3D('',#82369,#65080,#65081);
#54297=AXIS2_PLACEMENT_3D('',#82375,#65085,#65086);
#54298=AXIS2_PLACEMENT_3D('',#82381,#65090,#65091);
#54299=AXIS2_PLACEMENT_3D('',#82384,#65094,#65095);
#54300=AXIS2_PLACEMENT_3D('',#82463,#65102,#65103);
#54301=AXIS2_PLACEMENT_3D('',#82469,#65107,#65108);
#54302=AXIS2_PLACEMENT_3D('',#82475,#65112,#65113);
#54303=AXIS2_PLACEMENT_3D('',#82481,#65117,#65118);
#54304=AXIS2_PLACEMENT_3D('',#82487,#65122,#65123);
#54305=AXIS2_PLACEMENT_3D('',#82493,#65127,#65128);
#54306=AXIS2_PLACEMENT_3D('',#82619,#65140,#65141);
#54307=AXIS2_PLACEMENT_3D('',#82652,#65146,#65147);
#54308=AXIS2_PLACEMENT_3D('',#82818,#65159,#65160);
#54309=AXIS2_PLACEMENT_3D('',#82987,#65173,#65174);
#54310=AXIS2_PLACEMENT_3D('',#83035,#65180,#65181);
#54311=AXIS2_PLACEMENT_3D('',#83036,#65182,#65183);
#54312=AXIS2_PLACEMENT_3D('',#83045,#65188,#65189);
#54313=AXIS2_PLACEMENT_3D('',#83051,#65193,#65194);
#54314=AXIS2_PLACEMENT_3D('',#83057,#65198,#65199);
#54315=AXIS2_PLACEMENT_3D('',#83063,#65203,#65204);
#54316=AXIS2_PLACEMENT_3D('',#83069,#65208,#65209);
#54317=AXIS2_PLACEMENT_3D('',#83075,#65213,#65214);
#54318=AXIS2_PLACEMENT_3D('',#83081,#65218,#65219);
#54319=AXIS2_PLACEMENT_3D('',#83087,#65223,#65224);
#54320=AXIS2_PLACEMENT_3D('',#83093,#65228,#65229);
#54321=AXIS2_PLACEMENT_3D('',#83099,#65233,#65234);
#54322=AXIS2_PLACEMENT_3D('',#83105,#65238,#65239);
#54323=AXIS2_PLACEMENT_3D('',#83108,#65242,#65243);
#54324=AXIS2_PLACEMENT_3D('',#83109,#65244,#65245);
#54325=AXIS2_PLACEMENT_3D('',#83118,#65250,#65251);
#54326=AXIS2_PLACEMENT_3D('',#83124,#65255,#65256);
#54327=AXIS2_PLACEMENT_3D('',#83130,#65260,#65261);
#54328=AXIS2_PLACEMENT_3D('',#83133,#65264,#65265);
#54329=AXIS2_PLACEMENT_3D('',#83299,#65277,#65278);
#54330=AXIS2_PLACEMENT_3D('',#83300,#65279,#65280);
#54331=AXIS2_PLACEMENT_3D('',#83309,#65285,#65286);
#54332=AXIS2_PLACEMENT_3D('',#83315,#65290,#65291);
#54333=AXIS2_PLACEMENT_3D('',#83321,#65295,#65296);
#54334=AXIS2_PLACEMENT_3D('',#83327,#65300,#65301);
#54335=AXIS2_PLACEMENT_3D('',#83333,#65305,#65306);
#54336=AXIS2_PLACEMENT_3D('',#83339,#65310,#65311);
#54337=AXIS2_PLACEMENT_3D('',#83345,#65315,#65316);
#54338=AXIS2_PLACEMENT_3D('',#83351,#65320,#65321);
#54339=AXIS2_PLACEMENT_3D('',#83357,#65325,#65326);
#54340=AXIS2_PLACEMENT_3D('',#83363,#65330,#65331);
#54341=AXIS2_PLACEMENT_3D('',#83369,#65335,#65336);
#54342=AXIS2_PLACEMENT_3D('',#83372,#65339,#65340);
#54343=AXIS2_PLACEMENT_3D('',#83373,#65341,#65342);
#54344=AXIS2_PLACEMENT_3D('',#83382,#65347,#65348);
#54345=AXIS2_PLACEMENT_3D('',#83388,#65352,#65353);
#54346=AXIS2_PLACEMENT_3D('',#83394,#65357,#65358);
#54347=AXIS2_PLACEMENT_3D('',#83400,#65362,#65363);
#54348=AXIS2_PLACEMENT_3D('',#83406,#65367,#65368);
#54349=AXIS2_PLACEMENT_3D('',#83409,#65371,#65372);
#54350=AXIS2_PLACEMENT_3D('',#83533,#65382,#65383);
#54351=AXIS2_PLACEMENT_3D('',#83539,#65387,#65388);
#54352=AXIS2_PLACEMENT_3D('',#83545,#65392,#65393);
#54353=AXIS2_PLACEMENT_3D('',#83563,#65397,#65398);
#54354=AXIS2_PLACEMENT_3D('',#83564,#65399,#65400);
#54355=AXIS2_PLACEMENT_3D('',#83633,#65409,#65410);
#54356=AXIS2_PLACEMENT_3D('',#83639,#65414,#65415);
#54357=AXIS2_PLACEMENT_3D('',#83645,#65419,#65420);
#54358=AXIS2_PLACEMENT_3D('',#83756,#65431,#65432);
#54359=AXIS2_PLACEMENT_3D('',#83762,#65436,#65437);
#54360=AXIS2_PLACEMENT_3D('',#83768,#65441,#65442);
#54361=AXIS2_PLACEMENT_3D('',#83774,#65446,#65447);
#54362=AXIS2_PLACEMENT_3D('',#83777,#65450,#65451);
#54363=AXIS2_PLACEMENT_3D('',#83778,#65452,#65453);
#54364=AXIS2_PLACEMENT_3D('',#83787,#65458,#65459);
#54365=AXIS2_PLACEMENT_3D('',#83793,#65463,#65464);
#54366=AXIS2_PLACEMENT_3D('',#83799,#65468,#65469);
#54367=AXIS2_PLACEMENT_3D('',#83802,#65472,#65473);
#54368=AXIS2_PLACEMENT_3D('',#83803,#65474,#65475);
#54369=AXIS2_PLACEMENT_3D('',#83805,#65476,#65477);
#54370=AXIS2_PLACEMENT_3D('',#83808,#65479,#65480);
#54371=AXIS2_PLACEMENT_3D('',#83809,#65481,#65482);
#54372=AXIS2_PLACEMENT_3D('',#83811,#65483,#65484);
#54373=AXIS2_PLACEMENT_3D('',#83813,#65486,#65487);
#54374=AXIS2_PLACEMENT_3D('',#83818,#65489,#65490);
#54375=AXIS2_PLACEMENT_3D('',#83822,#65492,#65493);
#54376=AXIS2_PLACEMENT_3D('',#83826,#65495,#65496);
#54377=AXIS2_PLACEMENT_3D('',#83829,#65498,#65499);
#54378=AXIS2_PLACEMENT_3D('',#83831,#65500,#65501);
#54379=AXIS2_PLACEMENT_3D('',#83833,#65502,#65503);
#54380=AXIS2_PLACEMENT_3D('',#83835,#65504,#65505);
#54381=AXIS2_PLACEMENT_3D('',#83837,#65506,#65507);
#54382=AXIS2_PLACEMENT_3D('',#83839,#65508,#65509);
#54383=AXIS2_PLACEMENT_3D('',#83841,#65510,#65511);
#54384=AXIS2_PLACEMENT_3D('',#83843,#65512,#65513);
#54385=AXIS2_PLACEMENT_3D('',#83845,#65514,#65515);
#54386=AXIS2_PLACEMENT_3D('',#83847,#65516,#65517);
#54387=AXIS2_PLACEMENT_3D('',#83849,#65518,#65519);
#54388=AXIS2_PLACEMENT_3D('',#83850,#65520,#65521);
#54389=AXIS2_PLACEMENT_3D('',#83852,#65522,#65523);
#54390=AXIS2_PLACEMENT_3D('',#83854,#65525,#65526);
#54391=AXIS2_PLACEMENT_3D('',#83857,#65527,#65528);
#54392=AXIS2_PLACEMENT_3D('',#83861,#65530,#65531);
#54393=AXIS2_PLACEMENT_3D('',#83865,#65533,#65534);
#54394=AXIS2_PLACEMENT_3D('',#83869,#65536,#65537);
#54395=AXIS2_PLACEMENT_3D('',#83872,#65539,#65540);
#54396=AXIS2_PLACEMENT_3D('',#83874,#65541,#65542);
#54397=AXIS2_PLACEMENT_3D('',#83876,#65543,#65544);
#54398=AXIS2_PLACEMENT_3D('',#83877,#65545,#65546);
#54399=AXIS2_PLACEMENT_3D('',#83880,#65548,#65549);
#54400=AXIS2_PLACEMENT_3D('',#83881,#65550,#65551);
#54401=AXIS2_PLACEMENT_3D('',#83883,#65552,#65553);
#54402=AXIS2_PLACEMENT_3D('',#83885,#65555,#65556);
#54403=AXIS2_PLACEMENT_3D('',#83887,#65558,#65559);
#54404=AXIS2_PLACEMENT_3D('',#83890,#65561,#65562);
#54405=AXIS2_PLACEMENT_3D('',#83891,#65563,#65564);
#54406=AXIS2_PLACEMENT_3D('',#83893,#65565,#65566);
#54407=AXIS2_PLACEMENT_3D('',#83895,#65568,#65569);
#54408=AXIS2_PLACEMENT_3D('',#83897,#65571,#65572);
#54409=AXIS2_PLACEMENT_3D('',#83900,#65574,#65575);
#54410=AXIS2_PLACEMENT_3D('',#83901,#65576,#65577);
#54411=AXIS2_PLACEMENT_3D('',#83903,#65578,#65579);
#54412=AXIS2_PLACEMENT_3D('',#83905,#65581,#65582);
#54413=AXIS2_PLACEMENT_3D('',#83907,#65584,#65585);
#54414=AXIS2_PLACEMENT_3D('',#83909,#65586,#65587);
#54415=AXIS2_PLACEMENT_3D('',#83912,#65589,#65590);
#54416=AXIS2_PLACEMENT_3D('',#83914,#65592,#65593);
#54417=AXIS2_PLACEMENT_3D('',#83916,#65594,#65595);
#54418=AXIS2_PLACEMENT_3D('',#83919,#65597,#65598);
#54419=AXIS2_PLACEMENT_3D('',#83921,#65600,#65601);
#54420=AXIS2_PLACEMENT_3D('',#83923,#65602,#65603);
#54421=AXIS2_PLACEMENT_3D('',#83926,#65605,#65606);
#54422=AXIS2_PLACEMENT_3D('',#83929,#65608,#65609);
#54423=AXIS2_PLACEMENT_3D('',#83930,#65610,#65611);
#54424=AXIS2_PLACEMENT_3D('',#83932,#65613,#65614);
#54425=AXIS2_PLACEMENT_3D('',#83934,#65615,#65616);
#54426=AXIS2_PLACEMENT_3D('',#83937,#65618,#65619);
#54427=AXIS2_PLACEMENT_3D('',#83940,#65621,#65622);
#54428=AXIS2_PLACEMENT_3D('',#83941,#65623,#65624);
#54429=AXIS2_PLACEMENT_3D('',#83943,#65626,#65627);
#54430=AXIS2_PLACEMENT_3D('',#83945,#65628,#65629);
#54431=AXIS2_PLACEMENT_3D('',#83948,#65631,#65632);
#54432=AXIS2_PLACEMENT_3D('',#83951,#65634,#65635);
#54433=AXIS2_PLACEMENT_3D('',#83952,#65636,#65637);
#54434=AXIS2_PLACEMENT_3D('',#83954,#65639,#65640);
#54435=AXIS2_PLACEMENT_3D('',#83956,#65641,#65642);
#54436=AXIS2_PLACEMENT_3D('',#83959,#65644,#65645);
#54437=AXIS2_PLACEMENT_3D('',#83962,#65647,#65648);
#54438=AXIS2_PLACEMENT_3D('',#83963,#65649,#65650);
#54439=AXIS2_PLACEMENT_3D('',#83965,#65652,#65653);
#54440=AXIS2_PLACEMENT_3D('',#83967,#65654,#65655);
#54441=AXIS2_PLACEMENT_3D('',#83969,#65657,#65658);
#54442=AXIS2_PLACEMENT_3D('',#83970,#65659,#65660);
#54443=AXIS2_PLACEMENT_3D('',#83974,#65662,#65663);
#54444=AXIS2_PLACEMENT_3D('',#83976,#65665,#65666);
#54445=AXIS2_PLACEMENT_3D('',#83980,#65669,#65670);
#54446=AXIS2_PLACEMENT_3D('',#83983,#65672,#65673);
#54447=AXIS2_PLACEMENT_3D('',#83984,#65674,#65675);
#54448=AXIS2_PLACEMENT_3D('',#83988,#65678,#65679);
#54449=AXIS2_PLACEMENT_3D('',#83991,#65681,#65682);
#54450=AXIS2_PLACEMENT_3D('',#83992,#65683,#65684);
#54451=AXIS2_PLACEMENT_3D('',#83996,#65687,#65688);
#54452=AXIS2_PLACEMENT_3D('',#83999,#65690,#65691);
#54453=AXIS2_PLACEMENT_3D('',#84000,#65692,#65693);
#54454=AXIS2_PLACEMENT_3D('',#84002,#65695,#65696);
#54455=AXIS2_PLACEMENT_3D('',#84008,#65700,#65701);
#54456=AXIS2_PLACEMENT_3D('',#84011,#65703,#65704);
#54457=AXIS2_PLACEMENT_3D('',#84012,#65705,#65706);
#54458=AXIS2_PLACEMENT_3D('',#84016,#65709,#65710);
#54459=AXIS2_PLACEMENT_3D('',#84019,#65712,#65713);
#54460=AXIS2_PLACEMENT_3D('',#84020,#65714,#65715);
#54461=AXIS2_PLACEMENT_3D('',#84023,#65718,#65719);
#54462=AXIS2_PLACEMENT_3D('',#84025,#65721,#65722);
#54463=AXIS2_PLACEMENT_3D('',#84027,#65724,#65725);
#54464=AXIS2_PLACEMENT_3D('',#84029,#65727,#65728);
#54465=AXIS2_PLACEMENT_3D('',#84033,#65731,#65732);
#54466=AXIS2_PLACEMENT_3D('',#84036,#65734,#65735);
#54467=AXIS2_PLACEMENT_3D('',#84037,#65736,#65737);
#54468=AXIS2_PLACEMENT_3D('',#84041,#65740,#65741);
#54469=AXIS2_PLACEMENT_3D('',#84042,#65742,#65743);
#54470=AXIS2_PLACEMENT_3D('',#84043,#65744,#65745);
#54471=AXIS2_PLACEMENT_3D('',#84045,#65747,#65748);
#54472=AXIS2_PLACEMENT_3D('',#84047,#65750,#65751);
#54473=AXIS2_PLACEMENT_3D('',#84049,#65753,#65754);
#64623=DIRECTION('axis',(0.,0.,1.));
#64624=DIRECTION('refdir',(1.,0.,0.));
#64625=DIRECTION('center_axis',(0.,1.,0.));
#64626=DIRECTION('ref_axis',(1.,0.,0.));
#64627=DIRECTION('',(1.,0.,0.));
#64628=DIRECTION('',(0.,0.,-1.));
#64629=DIRECTION('',(1.,0.,0.));
#64630=DIRECTION('',(0.,0.,-1.));
#64631=DIRECTION('center_axis',(1.,0.,0.));
#64632=DIRECTION('ref_axis',(0.,-1.,0.));
#64633=DIRECTION('',(0.,-1.,0.));
#64634=DIRECTION('',(0.,0.,-1.));
#64635=DIRECTION('',(0.,-1.,0.));
#64636=DIRECTION('center_axis',(0.,-1.,0.));
#64637=DIRECTION('ref_axis',(-1.,0.,0.));
#64638=DIRECTION('',(-1.,0.,0.));
#64639=DIRECTION('',(0.,0.,-1.));
#64640=DIRECTION('',(-1.,0.,0.));
#64641=DIRECTION('center_axis',(1.,0.,0.));
#64642=DIRECTION('ref_axis',(0.,-1.,0.));
#64643=DIRECTION('',(0.,-1.,0.));
#64644=DIRECTION('',(0.,0.,-1.));
#64645=DIRECTION('',(0.,-1.,0.));
#64646=DIRECTION('center_axis',(0.,1.,0.));
#64647=DIRECTION('ref_axis',(1.,0.,0.));
#64648=DIRECTION('',(1.,0.,0.));
#64649=DIRECTION('',(0.,0.,-1.));
#64650=DIRECTION('',(1.,0.,0.));
#64651=DIRECTION('center_axis',(1.,0.,0.));
#64652=DIRECTION('ref_axis',(0.,-1.,0.));
#64653=DIRECTION('',(0.,-1.,0.));
#64654=DIRECTION('',(0.,0.,-1.));
#64655=DIRECTION('',(0.,-1.,0.));
#64656=DIRECTION('center_axis',(0.,-1.,0.));
#64657=DIRECTION('ref_axis',(-1.,0.,0.));
#64658=DIRECTION('',(-1.,0.,0.));
#64659=DIRECTION('',(0.,0.,-1.));
#64660=DIRECTION('',(-1.,0.,0.));
#64661=DIRECTION('center_axis',(1.,0.,0.));
#64662=DIRECTION('ref_axis',(0.,-1.,0.));
#64663=DIRECTION('',(0.,-1.,0.));
#64664=DIRECTION('',(0.,0.,-1.));
#64665=DIRECTION('',(0.,-1.,0.));
#64666=DIRECTION('center_axis',(0.,1.,0.));
#64667=DIRECTION('ref_axis',(1.,0.,0.));
#64668=DIRECTION('',(1.,0.,0.));
#64669=DIRECTION('',(0.,0.,-1.));
#64670=DIRECTION('',(1.,0.,0.));
#64671=DIRECTION('center_axis',(-1.,0.,0.));
#64672=DIRECTION('ref_axis',(0.,1.,0.));
#64673=DIRECTION('',(0.,1.,0.));
#64674=DIRECTION('',(0.,0.,-1.));
#64675=DIRECTION('',(0.,1.,0.));
#64676=DIRECTION('center_axis',(0.,-1.,0.));
#64677=DIRECTION('ref_axis',(-1.,0.,0.));
#64678=DIRECTION('',(-1.,0.,0.));
#64679=DIRECTION('',(0.,0.,-1.));
#64680=DIRECTION('',(-1.,0.,0.));
#64681=DIRECTION('center_axis',(1.,0.,0.));
#64682=DIRECTION('ref_axis',(0.,-1.,0.));
#64683=DIRECTION('',(0.,-1.,0.));
#64684=DIRECTION('',(0.,-1.,0.));
#64685=DIRECTION('center_axis',(0.,0.,-1.));
#64686=DIRECTION('ref_axis',(-1.,0.,0.));
#64687=DIRECTION('center_axis',(0.,1.,0.));
#64688=DIRECTION('ref_axis',(1.,0.,0.));
#64689=DIRECTION('',(1.,0.,0.));
#64690=DIRECTION('',(0.,0.,-1.));
#64691=DIRECTION('',(1.,0.,0.));
#64692=DIRECTION('',(0.,0.,-1.));
#64693=DIRECTION('center_axis',(-1.,0.,0.));
#64694=DIRECTION('ref_axis',(0.,1.,0.));
#64695=DIRECTION('',(0.,1.,0.));
#64696=DIRECTION('',(0.,0.,-1.));
#64697=DIRECTION('',(0.,1.,0.));
#64698=DIRECTION('center_axis',(0.,-1.,0.));
#64699=DIRECTION('ref_axis',(-1.,0.,0.));
#64700=DIRECTION('',(-1.,0.,0.));
#64701=DIRECTION('',(0.,0.,-1.));
#64702=DIRECTION('',(-1.,0.,0.));
#64703=DIRECTION('center_axis',(1.,0.,0.));
#64704=DIRECTION('ref_axis',(0.,-1.,0.));
#64705=DIRECTION('',(0.,-1.,0.));
#64706=DIRECTION('',(0.,-1.,0.));
#64707=DIRECTION('center_axis',(0.,0.,-1.));
#64708=DIRECTION('ref_axis',(-1.,0.,0.));
#64709=DIRECTION('',(0.,0.,-1.));
#64710=DIRECTION('',(0.,0.,-1.));
#64711=DIRECTION('',(0.,0.,-1.));
#64712=DIRECTION('',(0.,0.,-1.));
#64713=DIRECTION('',(0.,0.,-1.));
#64714=DIRECTION('',(0.,0.,-1.));
#64715=DIRECTION('',(0.,0.,-1.));
#64716=DIRECTION('',(0.,0.,-1.));
#64717=DIRECTION('',(0.,0.,-1.));
#64718=DIRECTION('',(0.,0.,-1.));
#64719=DIRECTION('',(0.,0.,-1.));
#64720=DIRECTION('',(0.,0.,-1.));
#64721=DIRECTION('',(0.,0.,-1.));
#64722=DIRECTION('',(0.,0.,-1.));
#64723=DIRECTION('center_axis',(0.0750546489289138,-0.997179422006971,0.));
#64724=DIRECTION('ref_axis',(-0.997179422006971,-0.0750546489289138,0.));
#64725=DIRECTION('',(-0.997179422006971,-0.0750546489289138,0.));
#64726=DIRECTION('',(0.,0.,-1.));
#64727=DIRECTION('',(-0.997179422006971,-0.0750546489289138,0.));
#64728=DIRECTION('',(0.,0.,-1.));
#64729=DIRECTION('',(0.,0.,-1.));
#64730=DIRECTION('',(0.,0.,-1.));
#64731=DIRECTION('',(0.,0.,-1.));
#64732=DIRECTION('',(0.,0.,-1.));
#64733=DIRECTION('',(0.,0.,-1.));
#64734=DIRECTION('',(0.,0.,-1.));
#64735=DIRECTION('',(0.,0.,-1.));
#64736=DIRECTION('',(0.,0.,-1.));
#64737=DIRECTION('',(0.,0.,-1.));
#64738=DIRECTION('',(0.,0.,-1.));
#64739=DIRECTION('',(0.,0.,-1.));
#64740=DIRECTION('',(0.,0.,-1.));
#64741=DIRECTION('',(0.,0.,-1.));
#64742=DIRECTION('',(0.,0.,-1.));
#64743=DIRECTION('',(0.,0.,-1.));
#64744=DIRECTION('',(0.,0.,-1.));
#64745=DIRECTION('',(0.,0.,-1.));
#64746=DIRECTION('center_axis',(-0.0871014161005409,0.996199449564835,0.));
#64747=DIRECTION('ref_axis',(0.996199449564835,0.0871014161005409,0.));
#64748=DIRECTION('',(0.996199449564835,0.0871014161005409,0.));
#64749=DIRECTION('',(0.,0.,-1.));
#64750=DIRECTION('',(0.996199449564835,0.0871014161005409,0.));
#64751=DIRECTION('',(0.,0.,-1.));
#64752=DIRECTION('center_axis',(0.,0.,1.));
#64753=DIRECTION('ref_axis',(1.,0.,0.));
#64754=DIRECTION('',(0.,0.,-1.));
#64755=DIRECTION('',(0.,0.,-1.));
#64756=DIRECTION('',(0.,0.,-1.));
#64757=DIRECTION('',(0.,0.,-1.));
#64758=DIRECTION('',(0.,0.,-1.));
#64759=DIRECTION('',(0.,0.,-1.));
#64760=DIRECTION('',(0.,0.,-1.));
#64761=DIRECTION('',(0.,0.,-1.));
#64762=DIRECTION('',(0.,0.,-1.));
#64763=DIRECTION('center_axis',(0.229319053916465,-0.973351309400084,0.));
#64764=DIRECTION('ref_axis',(-0.973351309400084,-0.229319053916465,0.));
#64765=DIRECTION('',(-0.973351309400084,-0.229319053916465,0.));
#64766=DIRECTION('',(0.,0.,-1.));
#64767=DIRECTION('',(-0.973351309400084,-0.229319053916465,0.));
#64768=DIRECTION('',(0.,0.,-1.));
#64769=DIRECTION('',(0.,0.,-1.));
#64770=DIRECTION('',(0.,0.,-1.));
#64771=DIRECTION('',(0.,0.,-1.));
#64772=DIRECTION('',(0.,0.,-1.));
#64773=DIRECTION('',(0.,0.,-1.));
#64774=DIRECTION('',(0.,0.,-1.));
#64775=DIRECTION('',(0.,0.,-1.));
#64776=DIRECTION('',(0.,0.,-1.));
#64777=DIRECTION('',(0.,0.,-1.));
#64778=DIRECTION('center_axis',(0.244891010635767,0.969550613897899,0.));
#64779=DIRECTION('ref_axis',(0.969550613897899,-0.244891010635767,0.));
#64780=DIRECTION('',(0.969550613897899,-0.244891010635767,0.));
#64781=DIRECTION('',(0.,0.,-1.));
#64782=DIRECTION('',(0.969550613897899,-0.244891010635767,0.));
#64783=DIRECTION('',(0.,0.,-1.));
#64784=DIRECTION('center_axis',(0.,0.,1.));
#64785=DIRECTION('ref_axis',(1.,0.,0.));
#64786=DIRECTION('center_axis',(0.,1.,0.));
#64787=DIRECTION('ref_axis',(1.,0.,0.));
#64788=DIRECTION('',(1.,0.,0.));
#64789=DIRECTION('',(0.,0.,-1.));
#64790=DIRECTION('',(1.,0.,0.));
#64791=DIRECTION('',(0.,0.,-1.));
#64792=DIRECTION('center_axis',(1.,0.,0.));
#64793=DIRECTION('ref_axis',(0.,-1.,0.));
#64794=DIRECTION('',(0.,-1.,0.));
#64795=DIRECTION('',(0.,0.,-1.));
#64796=DIRECTION('',(0.,-1.,0.));
#64797=DIRECTION('center_axis',(0.,1.,0.));
#64798=DIRECTION('ref_axis',(1.,0.,0.));
#64799=DIRECTION('',(1.,0.,0.));
#64800=DIRECTION('',(0.,0.,-1.));
#64801=DIRECTION('',(1.,0.,0.));
#64802=DIRECTION('center_axis',(-1.,0.,0.));
#64803=DIRECTION('ref_axis',(0.,1.,0.));
#64804=DIRECTION('',(0.,1.,0.));
#64805=DIRECTION('',(0.,0.,-1.));
#64806=DIRECTION('',(0.,1.,0.));
#64807=DIRECTION('center_axis',(0.,-1.,0.));
#64808=DIRECTION('ref_axis',(-1.,0.,0.));
#64809=DIRECTION('',(-1.,0.,0.));
#64810=DIRECTION('',(0.,0.,-1.));
#64811=DIRECTION('',(-1.,0.,0.));
#64812=DIRECTION('center_axis',(1.,0.,0.));
#64813=DIRECTION('ref_axis',(0.,-1.,0.));
#64814=DIRECTION('',(0.,-1.,0.));
#64815=DIRECTION('',(0.,-1.,0.));
#64816=DIRECTION('center_axis',(0.,0.,-1.));
#64817=DIRECTION('ref_axis',(-1.,0.,0.));
#64818=DIRECTION('center_axis',(0.,-1.,0.));
#64819=DIRECTION('ref_axis',(-1.,0.,0.));
#64820=DIRECTION('',(-1.,0.,0.));
#64821=DIRECTION('',(0.,0.,-1.));
#64822=DIRECTION('',(-1.,0.,0.));
#64823=DIRECTION('',(0.,0.,-1.));
#64824=DIRECTION('center_axis',(1.,0.,0.));
#64825=DIRECTION('ref_axis',(0.,-1.,0.));
#64826=DIRECTION('',(0.,-1.,0.));
#64827=DIRECTION('',(0.,0.,-1.));
#64828=DIRECTION('',(0.,-1.,0.));
#64829=DIRECTION('center_axis',(0.,1.,0.));
#64830=DIRECTION('ref_axis',(1.,0.,0.));
#64831=DIRECTION('',(1.,0.,0.));
#64832=DIRECTION('',(0.,0.,-1.));
#64833=DIRECTION('',(1.,0.,0.));
#64834=DIRECTION('center_axis',(-1.,0.,0.));
#64835=DIRECTION('ref_axis',(0.,1.,0.));
#64836=DIRECTION('',(0.,1.,0.));
#64837=DIRECTION('',(0.,0.,-1.));
#64838=DIRECTION('',(0.,1.,0.));
#64839=DIRECTION('center_axis',(0.,-1.,0.));
#64840=DIRECTION('ref_axis',(-1.,0.,0.));
#64841=DIRECTION('',(-1.,0.,0.));
#64842=DIRECTION('',(0.,0.,-1.));
#64843=DIRECTION('',(-1.,0.,0.));
#64844=DIRECTION('center_axis',(-1.,0.,0.));
#64845=DIRECTION('ref_axis',(0.,1.,0.));
#64846=DIRECTION('',(0.,1.,0.));
#64847=DIRECTION('',(0.,0.,-1.));
#64848=DIRECTION('',(0.,1.,0.));
#64849=DIRECTION('center_axis',(0.,-1.,0.));
#64850=DIRECTION('ref_axis',(-1.,0.,0.));
#64851=DIRECTION('',(-1.,0.,0.));
#64852=DIRECTION('',(0.,0.,-1.));
#64853=DIRECTION('',(-1.,0.,0.));
#64854=DIRECTION('center_axis',(1.,0.,0.));
#64855=DIRECTION('ref_axis',(0.,-1.,0.));
#64856=DIRECTION('',(0.,-1.,0.));
#64857=DIRECTION('',(0.,-1.,0.));
#64858=DIRECTION('center_axis',(0.,0.,-1.));
#64859=DIRECTION('ref_axis',(-1.,0.,0.));
#64860=DIRECTION('',(0.,0.,-1.));
#64861=DIRECTION('',(0.,0.,-1.));
#64862=DIRECTION('',(0.,0.,-1.));
#64863=DIRECTION('',(0.,0.,-1.));
#64864=DIRECTION('',(0.,0.,-1.));
#64865=DIRECTION('center_axis',(1.,0.,0.));
#64866=DIRECTION('ref_axis',(0.,-1.,0.));
#64867=DIRECTION('',(0.,-1.,0.));
#64868=DIRECTION('',(0.,0.,-1.));
#64869=DIRECTION('',(0.,-1.,0.));
#64870=DIRECTION('center_axis',(0.,1.,0.));
#64871=DIRECTION('ref_axis',(1.,0.,0.));
#64872=DIRECTION('',(1.,0.,0.));
#64873=DIRECTION('',(0.,0.,-1.));
#64874=DIRECTION('',(1.,0.,0.));
#64875=DIRECTION('center_axis',(-1.,0.,0.));
#64876=DIRECTION('ref_axis',(0.,1.,0.));
#64877=DIRECTION('',(0.,1.,0.));
#64878=DIRECTION('',(0.,0.,-1.));
#64879=DIRECTION('',(0.,1.,0.));
#64880=DIRECTION('',(0.,0.,-1.));
#64881=DIRECTION('',(0.,0.,-1.));
#64882=DIRECTION('',(0.,0.,-1.));
#64883=DIRECTION('',(0.,0.,-1.));
#64884=DIRECTION('',(0.,0.,-1.));
#64885=DIRECTION('',(0.,0.,-1.));
#64886=DIRECTION('center_axis',(1.,0.,0.));
#64887=DIRECTION('ref_axis',(0.,-1.,0.));
#64888=DIRECTION('',(0.,-1.,0.));
#64889=DIRECTION('',(0.,0.,-1.));
#64890=DIRECTION('',(0.,-1.,0.));
#64891=DIRECTION('center_axis',(0.,1.,0.));
#64892=DIRECTION('ref_axis',(1.,0.,0.));
#64893=DIRECTION('',(1.,0.,0.));
#64894=DIRECTION('',(0.,0.,-1.));
#64895=DIRECTION('',(1.,0.,0.));
#64896=DIRECTION('center_axis',(-1.,0.,0.));
#64897=DIRECTION('ref_axis',(0.,1.,0.));
#64898=DIRECTION('',(0.,1.,0.));
#64899=DIRECTION('',(0.,0.,-1.));
#64900=DIRECTION('',(0.,1.,0.));
#64901=DIRECTION('center_axis',(0.,0.,1.));
#64902=DIRECTION('ref_axis',(1.,0.,0.));
#64903=DIRECTION('center_axis',(0.,-1.,0.));
#64904=DIRECTION('ref_axis',(-1.,0.,0.));
#64905=DIRECTION('',(-1.,0.,0.));
#64906=DIRECTION('',(0.,0.,-1.));
#64907=DIRECTION('',(-1.,0.,0.));
#64908=DIRECTION('',(0.,0.,-1.));
#64909=DIRECTION('',(0.,0.,-1.));
#64910=DIRECTION('',(0.,0.,-1.));
#64911=DIRECTION('',(0.,0.,-1.));
#64912=DIRECTION('',(0.,0.,-1.));
#64913=DIRECTION('center_axis',(-0.843774210720013,-0.536698314999981,0.));
#64914=DIRECTION('ref_axis',(-0.536698314999981,0.843774210720013,0.));
#64915=DIRECTION('',(-0.536698314999981,0.843774210720013,0.));
#64916=DIRECTION('',(0.,0.,-1.));
#64917=DIRECTION('',(-0.536698314999981,0.843774210720013,0.));
#64918=DIRECTION('center_axis',(0.,-1.,0.));
#64919=DIRECTION('ref_axis',(-1.,0.,0.));
#64920=DIRECTION('',(-1.,0.,0.));
#64921=DIRECTION('',(0.,0.,-1.));
#64922=DIRECTION('',(-1.,0.,0.));
#64923=DIRECTION('center_axis',(0.842616728563894,0.538513740534336,0.));
#64924=DIRECTION('ref_axis',(0.538513740534336,-0.842616728563894,0.));
#64925=DIRECTION('',(0.538513740534336,-0.842616728563894,0.));
#64926=DIRECTION('',(0.,0.,-1.));
#64927=DIRECTION('',(0.538513740534336,-0.842616728563894,0.));
#64928=DIRECTION('',(0.,0.,-1.));
#64929=DIRECTION('',(0.,0.,-1.));
#64930=DIRECTION('',(0.,0.,-1.));
#64931=DIRECTION('',(0.,0.,-1.));
#64932=DIRECTION('',(0.,0.,-1.));
#64933=DIRECTION('',(0.,0.,-1.));
#64934=DIRECTION('',(0.,0.,-1.));
#64935=DIRECTION('center_axis',(0.,1.,0.));
#64936=DIRECTION('ref_axis',(1.,0.,0.));
#64937=DIRECTION('',(1.,0.,0.));
#64938=DIRECTION('',(0.,0.,-1.));
#64939=DIRECTION('',(1.,0.,0.));
#64940=DIRECTION('center_axis',(-1.,0.,0.));
#64941=DIRECTION('ref_axis',(0.,1.,0.));
#64942=DIRECTION('',(0.,1.,0.));
#64943=DIRECTION('',(0.,0.,-1.));
#64944=DIRECTION('',(0.,1.,0.));
#64945=DIRECTION('center_axis',(0.,-1.,0.));
#64946=DIRECTION('ref_axis',(-1.,0.,0.));
#64947=DIRECTION('',(-1.,0.,0.));
#64948=DIRECTION('',(0.,0.,-1.));
#64949=DIRECTION('',(-1.,0.,0.));
#64950=DIRECTION('center_axis',(1.,0.,0.));
#64951=DIRECTION('ref_axis',(0.,-1.,0.));
#64952=DIRECTION('',(0.,-1.,0.));
#64953=DIRECTION('',(0.,-1.,0.));
#64954=DIRECTION('center_axis',(0.,0.,1.));
#64955=DIRECTION('ref_axis',(1.,0.,0.));
#64956=DIRECTION('center_axis',(0.,-1.,0.));
#64957=DIRECTION('ref_axis',(-1.,0.,0.));
#64958=DIRECTION('',(-1.,0.,0.));
#64959=DIRECTION('',(0.,0.,-1.));
#64960=DIRECTION('',(-1.,0.,0.));
#64961=DIRECTION('',(0.,0.,-1.));
#64962=DIRECTION('center_axis',(1.,0.,0.));
#64963=DIRECTION('ref_axis',(0.,-1.,0.));
#64964=DIRECTION('',(0.,-1.,0.));
#64965=DIRECTION('',(0.,0.,-1.));
#64966=DIRECTION('',(0.,-1.,0.));
#64967=DIRECTION('center_axis',(0.,1.,0.));
#64968=DIRECTION('ref_axis',(1.,0.,0.));
#64969=DIRECTION('',(1.,0.,0.));
#64970=DIRECTION('',(0.,0.,-1.));
#64971=DIRECTION('',(1.,0.,0.));
#64972=DIRECTION('center_axis',(-1.,0.,0.));
#64973=DIRECTION('ref_axis',(0.,1.,0.));
#64974=DIRECTION('',(0.,1.,0.));
#64975=DIRECTION('',(0.,0.,-1.));
#64976=DIRECTION('',(0.,1.,0.));
#64977=DIRECTION('center_axis',(0.,-1.,0.));
#64978=DIRECTION('ref_axis',(-1.,0.,0.));
#64979=DIRECTION('',(-1.,0.,0.));
#64980=DIRECTION('',(0.,0.,-1.));
#64981=DIRECTION('',(-1.,0.,0.));
#64982=DIRECTION('center_axis',(-1.,0.,0.));
#64983=DIRECTION('ref_axis',(0.,1.,0.));
#64984=DIRECTION('',(0.,1.,0.));
#64985=DIRECTION('',(0.,0.,-1.));
#64986=DIRECTION('',(0.,1.,0.));
#64987=DIRECTION('center_axis',(0.,-1.,0.));
#64988=DIRECTION('ref_axis',(-1.,0.,0.));
#64989=DIRECTION('',(-1.,0.,0.));
#64990=DIRECTION('',(0.,0.,-1.));
#64991=DIRECTION('',(-1.,0.,0.));
#64992=DIRECTION('center_axis',(1.,0.,0.));
#64993=DIRECTION('ref_axis',(0.,-1.,0.));
#64994=DIRECTION('',(0.,-1.,0.));
#64995=DIRECTION('',(0.,-1.,0.));
#64996=DIRECTION('center_axis',(0.,0.,-1.));
#64997=DIRECTION('ref_axis',(-1.,0.,0.));
#64998=DIRECTION('',(0.,0.,-1.));
#64999=DIRECTION('',(0.,0.,-1.));
#65000=DIRECTION('',(0.,0.,-1.));
#65001=DIRECTION('center_axis',(-1.,1.10046549710191E-14,0.));
#65002=DIRECTION('ref_axis',(1.10046549710191E-14,1.,0.));
#65003=DIRECTION('',(1.10046549710191E-14,1.,0.));
#65004=DIRECTION('',(0.,0.,-1.));
#65005=DIRECTION('',(1.10046549710191E-14,1.,0.));
#65006=DIRECTION('',(0.,0.,-1.));
#65007=DIRECTION('',(0.,0.,-1.));
#65008=DIRECTION('center_axis',(-1.,0.,0.));
#65009=DIRECTION('ref_axis',(0.,1.,0.));
#65010=DIRECTION('',(0.,1.,0.));
#65011=DIRECTION('',(0.,0.,-1.));
#65012=DIRECTION('',(0.,1.,0.));
#65013=DIRECTION('center_axis',(0.,-1.,0.));
#65014=DIRECTION('ref_axis',(-1.,0.,0.));
#65015=DIRECTION('',(-1.,0.,0.));
#65016=DIRECTION('',(0.,0.,-1.));
#65017=DIRECTION('',(-1.,0.,0.));
#65018=DIRECTION('center_axis',(1.,0.,0.));
#65019=DIRECTION('ref_axis',(0.,-1.,0.));
#65020=DIRECTION('',(0.,-1.,0.));
#65021=DIRECTION('',(0.,0.,-1.));
#65022=DIRECTION('',(0.,-1.,0.));
#65023=DIRECTION('center_axis',(0.,1.,0.));
#65024=DIRECTION('ref_axis',(1.,0.,0.));
#65025=DIRECTION('',(1.,0.,0.));
#65026=DIRECTION('',(1.,0.,0.));
#65027=DIRECTION('center_axis',(0.,0.,1.));
#65028=DIRECTION('ref_axis',(1.,0.,0.));
#65029=DIRECTION('',(0.,0.,-1.));
#65030=DIRECTION('',(0.,0.,-1.));
#65031=DIRECTION('',(0.,0.,-1.));
#65032=DIRECTION('',(0.,0.,-1.));
#65033=DIRECTION('',(0.,0.,-1.));
#65034=DIRECTION('',(0.,0.,-1.));
#65035=DIRECTION('',(0.,0.,-1.));
#65036=DIRECTION('',(0.,0.,-1.));
#65037=DIRECTION('',(0.,0.,-1.));
#65038=DIRECTION('',(0.,0.,-1.));
#65039=DIRECTION('',(0.,0.,-1.));
#65040=DIRECTION('',(0.,0.,-1.));
#65041=DIRECTION('center_axis',(0.,0.,1.));
#65042=DIRECTION('ref_axis',(1.,0.,0.));
#65043=DIRECTION('',(0.,0.,-1.));
#65044=DIRECTION('',(0.,0.,-1.));
#65045=DIRECTION('',(0.,0.,-1.));
#65046=DIRECTION('center_axis',(-1.,0.,0.));
#65047=DIRECTION('ref_axis',(0.,1.,0.));
#65048=DIRECTION('',(0.,1.,0.));
#65049=DIRECTION('',(0.,0.,-1.));
#65050=DIRECTION('',(0.,1.,0.));
#65051=DIRECTION('',(0.,0.,-1.));
#65052=DIRECTION('',(0.,0.,-1.));
#65053=DIRECTION('center_axis',(-1.,0.,0.));
#65054=DIRECTION('ref_axis',(0.,1.,0.));
#65055=DIRECTION('',(0.,1.,0.));
#65056=DIRECTION('',(0.,0.,-1.));
#65057=DIRECTION('',(0.,1.,0.));
#65058=DIRECTION('center_axis',(0.,-1.,0.));
#65059=DIRECTION('ref_axis',(-1.,0.,0.));
#65060=DIRECTION('',(-1.,0.,0.));
#65061=DIRECTION('',(0.,0.,-1.));
#65062=DIRECTION('',(-1.,0.,0.));
#65063=DIRECTION('center_axis',(1.,0.,0.));
#65064=DIRECTION('ref_axis',(0.,-1.,0.));
#65065=DIRECTION('',(0.,-1.,0.));
#65066=DIRECTION('',(0.,0.,-1.));
#65067=DIRECTION('',(0.,-1.,0.));
#65068=DIRECTION('center_axis',(0.,1.,0.));
#65069=DIRECTION('ref_axis',(1.,0.,0.));
#65070=DIRECTION('',(1.,0.,0.));
#65071=DIRECTION('',(1.,0.,0.));
#65072=DIRECTION('center_axis',(0.,0.,1.));
#65073=DIRECTION('ref_axis',(1.,0.,0.));
#65074=DIRECTION('center_axis',(0.,1.,0.));
#65075=DIRECTION('ref_axis',(1.,0.,0.));
#65076=DIRECTION('',(1.,0.,0.));
#65077=DIRECTION('',(0.,0.,-1.));
#65078=DIRECTION('',(1.,0.,0.));
#65079=DIRECTION('',(0.,0.,-1.));
#65080=DIRECTION('center_axis',(-1.,0.,0.));
#65081=DIRECTION('ref_axis',(0.,1.,0.));
#65082=DIRECTION('',(0.,1.,0.));
#65083=DIRECTION('',(0.,0.,-1.));
#65084=DIRECTION('',(0.,1.,0.));
#65085=DIRECTION('center_axis',(0.,-1.,0.));
#65086=DIRECTION('ref_axis',(-1.,0.,0.));
#65087=DIRECTION('',(-1.,0.,0.));
#65088=DIRECTION('',(0.,0.,-1.));
#65089=DIRECTION('',(-1.,0.,0.));
#65090=DIRECTION('center_axis',(1.,0.,0.));
#65091=DIRECTION('ref_axis',(0.,-1.,0.));
#65092=DIRECTION('',(0.,-1.,0.));
#65093=DIRECTION('',(0.,-1.,0.));
#65094=DIRECTION('center_axis',(0.,0.,-1.));
#65095=DIRECTION('ref_axis',(-1.,0.,0.));
#65096=DIRECTION('',(0.,0.,-1.));
#65097=DIRECTION('',(0.,0.,-1.));
#65098=DIRECTION('',(0.,0.,-1.));
#65099=DIRECTION('',(0.,0.,-1.));
#65100=DIRECTION('',(0.,0.,-1.));
#65101=DIRECTION('',(0.,0.,-1.));
#65102=DIRECTION('center_axis',(0.980484772608259,-0.196595042367124,0.));
#65103=DIRECTION('ref_axis',(-0.196595042367124,-0.980484772608259,0.));
#65104=DIRECTION('',(-0.196595042367124,-0.980484772608259,0.));
#65105=DIRECTION('',(0.,0.,-1.));
#65106=DIRECTION('',(-0.196595042367124,-0.980484772608259,0.));
#65107=DIRECTION('center_axis',(0.,-1.,0.));
#65108=DIRECTION('ref_axis',(-1.,0.,0.));
#65109=DIRECTION('',(-1.,0.,0.));
#65110=DIRECTION('',(0.,0.,-1.));
#65111=DIRECTION('',(-1.,0.,0.));
#65112=DIRECTION('center_axis',(1.,0.,0.));
#65113=DIRECTION('ref_axis',(0.,-1.,0.));
#65114=DIRECTION('',(0.,-1.,0.));
#65115=DIRECTION('',(0.,0.,-1.));
#65116=DIRECTION('',(0.,-1.,0.));
#65117=DIRECTION('center_axis',(0.,1.,0.));
#65118=DIRECTION('ref_axis',(1.,0.,0.));
#65119=DIRECTION('',(1.,0.,0.));
#65120=DIRECTION('',(0.,0.,-1.));
#65121=DIRECTION('',(1.,0.,0.));
#65122=DIRECTION('center_axis',(-0.982679625842875,0.185312581745834,0.));
#65123=DIRECTION('ref_axis',(0.185312581745834,0.982679625842876,0.));
#65124=DIRECTION('',(0.185312581745834,0.982679625842876,0.));
#65125=DIRECTION('',(0.,0.,-1.));
#65126=DIRECTION('',(0.185312581745834,0.982679625842876,0.));
#65127=DIRECTION('center_axis',(-0.129088850062387,-0.991633031312275,0.));
#65128=DIRECTION('ref_axis',(-0.991633031312275,0.129088850062387,0.));
#65129=DIRECTION('',(-0.991633031312275,0.129088850062387,0.));
#65130=DIRECTION('',(0.,0.,-1.));
#65131=DIRECTION('',(-0.991633031312275,0.129088850062387,0.));
#65132=DIRECTION('',(0.,0.,-1.));
#65133=DIRECTION('',(0.,0.,-1.));
#65134=DIRECTION('',(0.,0.,-1.));
#65135=DIRECTION('',(0.,0.,-1.));
#65136=DIRECTION('',(0.,0.,-1.));
#65137=DIRECTION('',(0.,0.,-1.));
#65138=DIRECTION('',(0.,0.,-1.));
#65139=DIRECTION('',(0.,0.,-1.));
#65140=DIRECTION('center_axis',(-0.0843535578886116,0.99643588718569,0.));
#65141=DIRECTION('ref_axis',(0.99643588718569,0.0843535578886116,0.));
#65142=DIRECTION('',(0.99643588718569,0.0843535578886116,0.));
#65143=DIRECTION('',(0.,0.,-1.));
#65144=DIRECTION('',(0.99643588718569,0.0843535578886116,0.));
#65145=DIRECTION('',(0.,0.,-1.));
#65146=DIRECTION('center_axis',(0.,0.,1.));
#65147=DIRECTION('ref_axis',(1.,0.,0.));
#65148=DIRECTION('',(0.,0.,-1.));
#65149=DIRECTION('',(0.,0.,-1.));
#65150=DIRECTION('',(0.,0.,-1.));
#65151=DIRECTION('',(0.,0.,-1.));
#65152=DIRECTION('',(0.,0.,-1.));
#65153=DIRECTION('',(0.,0.,-1.));
#65154=DIRECTION('',(0.,0.,-1.));
#65155=DIRECTION('',(0.,0.,-1.));
#65156=DIRECTION('',(0.,0.,-1.));
#65157=DIRECTION('',(0.,0.,-1.));
#65158=DIRECTION('',(0.,0.,-1.));
#65159=DIRECTION('center_axis',(0.,0.,1.));
#65160=DIRECTION('ref_axis',(1.,0.,0.));
#65161=DIRECTION('',(0.,0.,-1.));
#65162=DIRECTION('',(0.,0.,-1.));
#65163=DIRECTION('',(0.,0.,-1.));
#65164=DIRECTION('',(0.,0.,-1.));
#65165=DIRECTION('',(0.,0.,-1.));
#65166=DIRECTION('',(0.,0.,-1.));
#65167=DIRECTION('',(0.,0.,-1.));
#65168=DIRECTION('',(0.,0.,-1.));
#65169=DIRECTION('',(0.,0.,-1.));
#65170=DIRECTION('',(0.,0.,-1.));
#65171=DIRECTION('',(0.,0.,-1.));
#65172=DIRECTION('',(0.,0.,-1.));
#65173=DIRECTION('center_axis',(0.921250259693202,-0.388970383210866,0.));
#65174=DIRECTION('ref_axis',(-0.388970383210866,-0.921250259693202,0.));
#65175=DIRECTION('',(-0.388970383210866,-0.921250259693202,0.));
#65176=DIRECTION('',(0.,0.,-1.));
#65177=DIRECTION('',(-0.388970383210866,-0.921250259693202,0.));
#65178=DIRECTION('',(0.,0.,-1.));
#65179=DIRECTION('',(0.,0.,-1.));
#65180=DIRECTION('center_axis',(0.,0.,1.));
#65181=DIRECTION('ref_axis',(1.,0.,0.));
#65182=DIRECTION('center_axis',(0.,1.,0.));
#65183=DIRECTION('ref_axis',(1.,0.,0.));
#65184=DIRECTION('',(1.,0.,0.));
#65185=DIRECTION('',(0.,0.,-1.));
#65186=DIRECTION('',(1.,0.,0.));
#65187=DIRECTION('',(0.,0.,-1.));
#65188=DIRECTION('center_axis',(1.,0.,0.));
#65189=DIRECTION('ref_axis',(0.,-1.,0.));
#65190=DIRECTION('',(0.,-1.,0.));
#65191=DIRECTION('',(0.,0.,-1.));
#65192=DIRECTION('',(0.,-1.,0.));
#65193=DIRECTION('center_axis',(0.,-1.,0.));
#65194=DIRECTION('ref_axis',(-1.,0.,0.));
#65195=DIRECTION('',(-1.,0.,0.));
#65196=DIRECTION('',(0.,0.,-1.));
#65197=DIRECTION('',(-1.,0.,0.));
#65198=DIRECTION('center_axis',(1.,0.,0.));
#65199=DIRECTION('ref_axis',(0.,-1.,0.));
#65200=DIRECTION('',(0.,-1.,0.));
#65201=DIRECTION('',(0.,0.,-1.));
#65202=DIRECTION('',(0.,-1.,0.));
#65203=DIRECTION('center_axis',(0.,1.,0.));
#65204=DIRECTION('ref_axis',(1.,0.,0.));
#65205=DIRECTION('',(1.,0.,0.));
#65206=DIRECTION('',(0.,0.,-1.));
#65207=DIRECTION('',(1.,0.,0.));
#65208=DIRECTION('center_axis',(1.,0.,0.));
#65209=DIRECTION('ref_axis',(0.,-1.,0.));
#65210=DIRECTION('',(0.,-1.,0.));
#65211=DIRECTION('',(0.,0.,-1.));
#65212=DIRECTION('',(0.,-1.,0.));
#65213=DIRECTION('center_axis',(0.,-1.,0.));
#65214=DIRECTION('ref_axis',(-1.,0.,0.));
#65215=DIRECTION('',(-1.,0.,0.));
#65216=DIRECTION('',(0.,0.,-1.));
#65217=DIRECTION('',(-1.,0.,0.));
#65218=DIRECTION('center_axis',(1.,0.,0.));
#65219=DIRECTION('ref_axis',(0.,-1.,0.));
#65220=DIRECTION('',(0.,-1.,0.));
#65221=DIRECTION('',(0.,0.,-1.));
#65222=DIRECTION('',(0.,-1.,0.));
#65223=DIRECTION('center_axis',(0.,1.,0.));
#65224=DIRECTION('ref_axis',(1.,0.,0.));
#65225=DIRECTION('',(1.,0.,0.));
#65226=DIRECTION('',(0.,0.,-1.));
#65227=DIRECTION('',(1.,0.,0.));
#65228=DIRECTION('center_axis',(-1.,0.,0.));
#65229=DIRECTION('ref_axis',(0.,1.,0.));
#65230=DIRECTION('',(0.,1.,0.));
#65231=DIRECTION('',(0.,0.,-1.));
#65232=DIRECTION('',(0.,1.,0.));
#65233=DIRECTION('center_axis',(0.,-1.,0.));
#65234=DIRECTION('ref_axis',(-1.,0.,0.));
#65235=DIRECTION('',(-1.,0.,0.));
#65236=DIRECTION('',(0.,0.,-1.));
#65237=DIRECTION('',(-1.,0.,0.));
#65238=DIRECTION('center_axis',(1.,0.,0.));
#65239=DIRECTION('ref_axis',(0.,-1.,0.));
#65240=DIRECTION('',(0.,-1.,0.));
#65241=DIRECTION('',(0.,-1.,0.));
#65242=DIRECTION('center_axis',(0.,0.,-1.));
#65243=DIRECTION('ref_axis',(-1.,0.,0.));
#65244=DIRECTION('center_axis',(0.,1.,0.));
#65245=DIRECTION('ref_axis',(1.,0.,0.));
#65246=DIRECTION('',(1.,0.,0.));
#65247=DIRECTION('',(0.,0.,-1.));
#65248=DIRECTION('',(1.,0.,0.));
#65249=DIRECTION('',(0.,0.,-1.));
#65250=DIRECTION('center_axis',(-1.,0.,0.));
#65251=DIRECTION('ref_axis',(0.,1.,0.));
#65252=DIRECTION('',(0.,1.,0.));
#65253=DIRECTION('',(0.,0.,-1.));
#65254=DIRECTION('',(0.,1.,0.));
#65255=DIRECTION('center_axis',(0.,-1.,0.));
#65256=DIRECTION('ref_axis',(-1.,0.,0.));
#65257=DIRECTION('',(-1.,0.,0.));
#65258=DIRECTION('',(0.,0.,-1.));
#65259=DIRECTION('',(-1.,0.,0.));
#65260=DIRECTION('center_axis',(1.,0.,0.));
#65261=DIRECTION('ref_axis',(0.,-1.,0.));
#65262=DIRECTION('',(0.,-1.,0.));
#65263=DIRECTION('',(0.,-1.,0.));
#65264=DIRECTION('center_axis',(0.,0.,-1.));
#65265=DIRECTION('ref_axis',(-1.,0.,0.));
#65266=DIRECTION('',(0.,0.,-1.));
#65267=DIRECTION('',(0.,0.,-1.));
#65268=DIRECTION('',(0.,0.,-1.));
#65269=DIRECTION('',(0.,0.,-1.));
#65270=DIRECTION('',(0.,0.,-1.));
#65271=DIRECTION('',(0.,0.,-1.));
#65272=DIRECTION('',(0.,0.,-1.));
#65273=DIRECTION('',(0.,0.,-1.));
#65274=DIRECTION('',(0.,0.,-1.));
#65275=DIRECTION('',(0.,0.,-1.));
#65276=DIRECTION('',(0.,0.,-1.));
#65277=DIRECTION('center_axis',(0.,0.,1.));
#65278=DIRECTION('ref_axis',(1.,0.,0.));
#65279=DIRECTION('center_axis',(0.698096755785859,-0.716003435439565,0.));
#65280=DIRECTION('ref_axis',(-0.716003435439565,-0.698096755785859,0.));
#65281=DIRECTION('',(-0.716003435439565,-0.698096755785859,0.));
#65282=DIRECTION('',(0.,0.,-1.));
#65283=DIRECTION('',(-0.716003435439565,-0.698096755785859,0.));
#65284=DIRECTION('',(0.,0.,-1.));
#65285=DIRECTION('center_axis',(-0.817885251670677,-0.575381364922078,0.));
#65286=DIRECTION('ref_axis',(-0.575381364922078,0.817885251670677,0.));
#65287=DIRECTION('',(-0.575381364922078,0.817885251670677,0.));
#65288=DIRECTION('',(0.,0.,-1.));
#65289=DIRECTION('',(-0.575381364922078,0.817885251670677,0.));
#65290=DIRECTION('center_axis',(0.,-1.,0.));
#65291=DIRECTION('ref_axis',(-1.,0.,0.));
#65292=DIRECTION('',(-1.,0.,0.));
#65293=DIRECTION('',(0.,0.,-1.));
#65294=DIRECTION('',(-1.,0.,0.));
#65295=DIRECTION('center_axis',(0.8052872827866,0.592884805153729,0.));
#65296=DIRECTION('ref_axis',(0.592884805153729,-0.8052872827866,0.));
#65297=DIRECTION('',(0.592884805153729,-0.8052872827866,0.));
#65298=DIRECTION('',(0.,0.,-1.));
#65299=DIRECTION('',(0.592884805153729,-0.8052872827866,0.));
#65300=DIRECTION('center_axis',(0.694718635560915,-0.719281598127173,0.));
#65301=DIRECTION('ref_axis',(-0.719281598127173,-0.694718635560915,0.));
#65302=DIRECTION('',(-0.719281598127173,-0.694718635560915,0.));
#65303=DIRECTION('',(0.,0.,-1.));
#65304=DIRECTION('',(-0.719281598127173,-0.694718635560915,0.));
#65305=DIRECTION('center_axis',(0.,1.,0.));
#65306=DIRECTION('ref_axis',(1.,0.,0.));
#65307=DIRECTION('',(1.,0.,0.));
#65308=DIRECTION('',(0.,0.,-1.));
#65309=DIRECTION('',(1.,0.,0.));
#65310=DIRECTION('center_axis',(-0.706620509307552,0.707592718889854,0.));
#65311=DIRECTION('ref_axis',(0.707592718889854,0.706620509307552,0.));
#65312=DIRECTION('',(0.707592718889854,0.706620509307552,0.));
#65313=DIRECTION('',(0.,0.,-1.));
#65314=DIRECTION('',(0.707592718889854,0.706620509307552,0.));
#65315=DIRECTION('center_axis',(1.,0.,0.));
#65316=DIRECTION('ref_axis',(0.,-1.,0.));
#65317=DIRECTION('',(0.,-1.,0.));
#65318=DIRECTION('',(0.,0.,-1.));
#65319=DIRECTION('',(0.,-1.,0.));
#65320=DIRECTION('center_axis',(0.,1.,0.));
#65321=DIRECTION('ref_axis',(1.,0.,0.));
#65322=DIRECTION('',(1.,0.,0.));
#65323=DIRECTION('',(0.,0.,-1.));
#65324=DIRECTION('',(1.,0.,0.));
#65325=DIRECTION('center_axis',(-1.,0.,0.));
#65326=DIRECTION('ref_axis',(0.,1.,0.));
#65327=DIRECTION('',(0.,1.,0.));
#65328=DIRECTION('',(0.,0.,-1.));
#65329=DIRECTION('',(0.,1.,0.));
#65330=DIRECTION('center_axis',(0.,-1.,0.));
#65331=DIRECTION('ref_axis',(-1.,0.,0.));
#65332=DIRECTION('',(-1.,0.,0.));
#65333=DIRECTION('',(0.,0.,-1.));
#65334=DIRECTION('',(-1.,0.,0.));
#65335=DIRECTION('center_axis',(1.,0.,0.));
#65336=DIRECTION('ref_axis',(0.,-1.,0.));
#65337=DIRECTION('',(0.,-1.,0.));
#65338=DIRECTION('',(0.,-1.,0.));
#65339=DIRECTION('center_axis',(0.,0.,-1.));
#65340=DIRECTION('ref_axis',(-1.,0.,0.));
#65341=DIRECTION('center_axis',(0.,1.,0.));
#65342=DIRECTION('ref_axis',(1.,0.,0.));
#65343=DIRECTION('',(1.,0.,0.));
#65344=DIRECTION('',(0.,0.,-1.));
#65345=DIRECTION('',(1.,0.,0.));
#65346=DIRECTION('',(0.,0.,-1.));
#65347=DIRECTION('center_axis',(1.,0.,0.));
#65348=DIRECTION('ref_axis',(0.,-1.,0.));
#65349=DIRECTION('',(0.,-1.,0.));
#65350=DIRECTION('',(0.,0.,-1.));
#65351=DIRECTION('',(0.,-1.,0.));
#65352=DIRECTION('center_axis',(0.,1.,0.));
#65353=DIRECTION('ref_axis',(1.,0.,0.));
#65354=DIRECTION('',(1.,0.,0.));
#65355=DIRECTION('',(0.,0.,-1.));
#65356=DIRECTION('',(1.,0.,0.));
#65357=DIRECTION('center_axis',(-1.,0.,0.));
#65358=DIRECTION('ref_axis',(0.,1.,0.));
#65359=DIRECTION('',(0.,1.,0.));
#65360=DIRECTION('',(0.,0.,-1.));
#65361=DIRECTION('',(0.,1.,0.));
#65362=DIRECTION('center_axis',(0.,-1.,0.));
#65363=DIRECTION('ref_axis',(-1.,0.,0.));
#65364=DIRECTION('',(-1.,0.,0.));
#65365=DIRECTION('',(0.,0.,-1.));
#65366=DIRECTION('',(-1.,0.,0.));
#65367=DIRECTION('center_axis',(1.,0.,0.));
#65368=DIRECTION('ref_axis',(0.,-1.,0.));
#65369=DIRECTION('',(0.,-1.,0.));
#65370=DIRECTION('',(0.,-1.,0.));
#65371=DIRECTION('center_axis',(0.,0.,-1.));
#65372=DIRECTION('ref_axis',(-1.,0.,0.));
#65373=DIRECTION('',(0.,0.,-1.));
#65374=DIRECTION('',(0.,0.,-1.));
#65375=DIRECTION('',(0.,0.,-1.));
#65376=DIRECTION('',(0.,0.,-1.));
#65377=DIRECTION('',(0.,0.,-1.));
#65378=DIRECTION('',(0.,0.,-1.));
#65379=DIRECTION('',(0.,0.,-1.));
#65380=DIRECTION('',(0.,0.,-1.));
#65381=DIRECTION('',(0.,0.,-1.));
#65382=DIRECTION('center_axis',(0.,1.,0.));
#65383=DIRECTION('ref_axis',(1.,0.,0.));
#65384=DIRECTION('',(1.,0.,0.));
#65385=DIRECTION('',(0.,0.,-1.));
#65386=DIRECTION('',(1.,0.,0.));
#65387=DIRECTION('center_axis',(-1.,0.,0.));
#65388=DIRECTION('ref_axis',(0.,1.,0.));
#65389=DIRECTION('',(0.,1.,0.));
#65390=DIRECTION('',(0.,0.,-1.));
#65391=DIRECTION('',(0.,1.,0.));
#65392=DIRECTION('center_axis',(0.,-1.,0.));
#65393=DIRECTION('ref_axis',(-1.,0.,0.));
#65394=DIRECTION('',(-1.,0.,0.));
#65395=DIRECTION('',(0.,0.,-1.));
#65396=DIRECTION('',(-1.,0.,0.));
#65397=DIRECTION('center_axis',(0.,0.,1.));
#65398=DIRECTION('ref_axis',(1.,0.,0.));
#65399=DIRECTION('center_axis',(0.,-1.,0.));
#65400=DIRECTION('ref_axis',(-1.,0.,0.));
#65401=DIRECTION('',(-1.,0.,0.));
#65402=DIRECTION('',(0.,0.,-1.));
#65403=DIRECTION('',(-1.,0.,0.));
#65404=DIRECTION('',(0.,0.,-1.));
#65405=DIRECTION('',(0.,0.,-1.));
#65406=DIRECTION('',(0.,0.,-1.));
#65407=DIRECTION('',(0.,0.,-1.));
#65408=DIRECTION('',(0.,0.,-1.));
#65409=DIRECTION('center_axis',(-0.843779362263309,-0.536690215877393,0.));
#65410=DIRECTION('ref_axis',(-0.536690215877393,0.843779362263309,0.));
#65411=DIRECTION('',(-0.536690215877393,0.843779362263309,0.));
#65412=DIRECTION('',(0.,0.,-1.));
#65413=DIRECTION('',(-0.536690215877393,0.843779362263309,0.));
#65414=DIRECTION('center_axis',(0.,-1.,0.));
#65415=DIRECTION('ref_axis',(-1.,0.,0.));
#65416=DIRECTION('',(-1.,0.,0.));
#65417=DIRECTION('',(0.,0.,-1.));
#65418=DIRECTION('',(-1.,0.,0.));
#65419=DIRECTION('center_axis',(0.842613773269381,0.538518364679178,0.));
#65420=DIRECTION('ref_axis',(0.538518364679178,-0.842613773269381,0.));
#65421=DIRECTION('',(0.538518364679178,-0.842613773269381,0.));
#65422=DIRECTION('',(0.,0.,-1.));
#65423=DIRECTION('',(0.538518364679178,-0.842613773269381,0.));
#65424=DIRECTION('',(0.,0.,-1.));
#65425=DIRECTION('',(0.,0.,-1.));
#65426=DIRECTION('',(0.,0.,-1.));
#65427=DIRECTION('',(0.,0.,-1.));
#65428=DIRECTION('',(0.,0.,-1.));
#65429=DIRECTION('',(0.,0.,-1.));
#65430=DIRECTION('',(0.,0.,-1.));
#65431=DIRECTION('center_axis',(0.,1.,0.));
#65432=DIRECTION('ref_axis',(1.,0.,0.));
#65433=DIRECTION('',(1.,0.,0.));
#65434=DIRECTION('',(0.,0.,-1.));
#65435=DIRECTION('',(1.,0.,0.));
#65436=DIRECTION('center_axis',(-1.,0.,0.));
#65437=DIRECTION('ref_axis',(0.,1.,0.));
#65438=DIRECTION('',(0.,1.,0.));
#65439=DIRECTION('',(0.,0.,-1.));
#65440=DIRECTION('',(0.,1.,0.));
#65441=DIRECTION('center_axis',(0.,-1.,0.));
#65442=DIRECTION('ref_axis',(-1.,0.,0.));
#65443=DIRECTION('',(-1.,0.,0.));
#65444=DIRECTION('',(0.,0.,-1.));
#65445=DIRECTION('',(-1.,0.,0.));
#65446=DIRECTION('center_axis',(1.,0.,0.));
#65447=DIRECTION('ref_axis',(0.,-1.,0.));
#65448=DIRECTION('',(0.,-1.,0.));
#65449=DIRECTION('',(0.,-1.,0.));
#65450=DIRECTION('center_axis',(0.,0.,1.));
#65451=DIRECTION('ref_axis',(1.,0.,0.));
#65452=DIRECTION('center_axis',(0.,-1.,0.));
#65453=DIRECTION('ref_axis',(1.,0.,0.));
#65454=DIRECTION('',(-1.,0.,0.));
#65455=DIRECTION('',(0.,0.,1.));
#65456=DIRECTION('',(1.,0.,0.));
#65457=DIRECTION('',(0.,0.,1.));
#65458=DIRECTION('center_axis',(-1.,0.,0.));
#65459=DIRECTION('ref_axis',(0.,-1.,0.));
#65460=DIRECTION('',(0.,1.,0.));
#65461=DIRECTION('',(0.,-1.,0.));
#65462=DIRECTION('',(0.,0.,1.));
#65463=DIRECTION('center_axis',(0.,1.,0.));
#65464=DIRECTION('ref_axis',(-1.,0.,0.));
#65465=DIRECTION('',(1.,0.,0.));
#65466=DIRECTION('',(-1.,0.,0.));
#65467=DIRECTION('',(0.,0.,1.));
#65468=DIRECTION('center_axis',(1.,0.,0.));
#65469=DIRECTION('ref_axis',(0.,1.,0.));
#65470=DIRECTION('',(0.,-1.,0.));
#65471=DIRECTION('',(0.,1.,0.));
#65472=DIRECTION('center_axis',(0.,0.,1.));
#65473=DIRECTION('ref_axis',(1.,0.,0.));
#65474=DIRECTION('center_axis',(0.,0.,1.));
#65475=DIRECTION('ref_axis',(1.,0.,0.));
#65476=DIRECTION('center_axis',(0.,0.,1.));
#65477=DIRECTION('ref_axis',(1.,0.,0.));
#65478=DIRECTION('',(0.707106781186546,8.65956056235491E-17,-0.707106781186549));
#65479=DIRECTION('center_axis',(0.,0.,-1.));
#65480=DIRECTION('ref_axis',(1.,0.,0.));
#65481=DIRECTION('center_axis',(0.,0.,1.));
#65482=DIRECTION('ref_axis',(1.,0.,0.));
#65483=DIRECTION('center_axis',(0.,0.,1.));
#65484=DIRECTION('ref_axis',(1.,0.,0.));
#65485=DIRECTION('',(0.,0.,1.));
#65486=DIRECTION('center_axis',(0.,0.,1.));
#65487=DIRECTION('ref_axis',(1.,0.,0.));
#65488=DIRECTION('',(0.,1.,0.));
#65489=DIRECTION('center_axis',(0.,0.,-1.));
#65490=DIRECTION('ref_axis',(-1.,0.,0.));
#65491=DIRECTION('',(-1.,0.,0.));
#65492=DIRECTION('center_axis',(0.,0.,-1.));
#65493=DIRECTION('ref_axis',(0.,-1.,0.));
#65494=DIRECTION('',(0.,-1.,0.));
#65495=DIRECTION('center_axis',(0.,0.,-1.));
#65496=DIRECTION('ref_axis',(1.,0.,0.));
#65497=DIRECTION('',(1.,0.,0.));
#65498=DIRECTION('center_axis',(0.,0.,-1.));
#65499=DIRECTION('ref_axis',(0.,1.,0.));
#65500=DIRECTION('center_axis',(0.,0.,1.));
#65501=DIRECTION('ref_axis',(1.,0.,0.));
#65502=DIRECTION('center_axis',(0.,0.,-1.));
#65503=DIRECTION('ref_axis',(1.,0.,0.));
#65504=DIRECTION('center_axis',(0.,0.,-1.));
#65505=DIRECTION('ref_axis',(1.,0.,0.));
#65506=DIRECTION('center_axis',(0.,0.,-1.));
#65507=DIRECTION('ref_axis',(1.,0.,0.));
#65508=DIRECTION('center_axis',(0.,0.,-1.));
#65509=DIRECTION('ref_axis',(1.,0.,0.));
#65510=DIRECTION('center_axis',(0.,0.,-1.));
#65511=DIRECTION('ref_axis',(1.,0.,0.));
#65512=DIRECTION('center_axis',(0.,0.,-1.));
#65513=DIRECTION('ref_axis',(1.,0.,0.));
#65514=DIRECTION('center_axis',(0.,0.,-1.));
#65515=DIRECTION('ref_axis',(1.,0.,0.));
#65516=DIRECTION('center_axis',(0.,0.,1.));
#65517=DIRECTION('ref_axis',(1.,0.,0.));
#65518=DIRECTION('center_axis',(0.,0.,1.));
#65519=DIRECTION('ref_axis',(1.,0.,0.));
#65520=DIRECTION('center_axis',(0.,0.,-1.));
#65521=DIRECTION('ref_axis',(1.,0.,0.));
#65522=DIRECTION('center_axis',(0.,0.,-1.));
#65523=DIRECTION('ref_axis',(1.,0.,0.));
#65524=DIRECTION('',(0.707106781186546,-8.65956056235491E-17,0.707106781186549));
#65525=DIRECTION('center_axis',(0.,0.,1.));
#65526=DIRECTION('ref_axis',(1.,0.,0.));
#65527=DIRECTION('center_axis',(0.,0.,1.));
#65528=DIRECTION('ref_axis',(0.,-1.,0.));
#65529=DIRECTION('',(1.,0.,0.));
#65530=DIRECTION('center_axis',(0.,0.,1.));
#65531=DIRECTION('ref_axis',(-1.,0.,0.));
#65532=DIRECTION('',(0.,-1.,0.));
#65533=DIRECTION('center_axis',(0.,0.,1.));
#65534=DIRECTION('ref_axis',(0.,1.,0.));
#65535=DIRECTION('',(-1.,0.,0.));
#65536=DIRECTION('center_axis',(0.,0.,1.));
#65537=DIRECTION('ref_axis',(1.,0.,0.));
#65538=DIRECTION('',(0.,1.,0.));
#65539=DIRECTION('center_axis',(0.,0.,-1.));
#65540=DIRECTION('ref_axis',(1.,0.,0.));
#65541=DIRECTION('center_axis',(0.,0.,-1.));
#65542=DIRECTION('ref_axis',(1.,0.,0.));
#65543=DIRECTION('center_axis',(0.,0.,-1.));
#65544=DIRECTION('ref_axis',(1.,0.,0.));
#65545=DIRECTION('center_axis',(0.,0.,1.));
#65546=DIRECTION('ref_axis',(1.,0.,0.));
#65547=DIRECTION('',(0.707106781186546,8.65956056235491E-17,-0.707106781186549));
#65548=DIRECTION('center_axis',(0.,0.,-1.));
#65549=DIRECTION('ref_axis',(1.,0.,0.));
#65550=DIRECTION('center_axis',(0.,0.,1.));
#65551=DIRECTION('ref_axis',(1.,0.,0.));
#65552=DIRECTION('center_axis',(0.,0.,1.));
#65553=DIRECTION('ref_axis',(1.,0.,0.));
#65554=DIRECTION('',(0.,0.,1.));
#65555=DIRECTION('center_axis',(0.,0.,-1.));
#65556=DIRECTION('ref_axis',(1.,0.,0.));
#65557=DIRECTION('',(0.707106781186546,-8.65956056235491E-17,0.707106781186549));
#65558=DIRECTION('center_axis',(0.,0.,1.));
#65559=DIRECTION('ref_axis',(1.,0.,0.));
#65560=DIRECTION('',(0.707106781186546,8.65956056235491E-17,-0.707106781186549));
#65561=DIRECTION('center_axis',(0.,0.,-1.));
#65562=DIRECTION('ref_axis',(1.,0.,0.));
#65563=DIRECTION('center_axis',(0.,0.,1.));
#65564=DIRECTION('ref_axis',(1.,0.,0.));
#65565=DIRECTION('center_axis',(0.,0.,1.));
#65566=DIRECTION('ref_axis',(1.,0.,0.));
#65567=DIRECTION('',(0.,0.,1.));
#65568=DIRECTION('center_axis',(0.,0.,-1.));
#65569=DIRECTION('ref_axis',(1.,0.,0.));
#65570=DIRECTION('',(0.707106781186546,-8.65956056235491E-17,0.707106781186549));
#65571=DIRECTION('center_axis',(0.,0.,1.));
#65572=DIRECTION('ref_axis',(1.,0.,0.));
#65573=DIRECTION('',(0.707106781186546,8.65956056235491E-17,-0.707106781186549));
#65574=DIRECTION('center_axis',(0.,0.,-1.));
#65575=DIRECTION('ref_axis',(1.,0.,0.));
#65576=DIRECTION('center_axis',(0.,0.,1.));
#65577=DIRECTION('ref_axis',(1.,0.,0.));
#65578=DIRECTION('center_axis',(0.,0.,1.));
#65579=DIRECTION('ref_axis',(1.,0.,0.));
#65580=DIRECTION('',(0.,0.,1.));
#65581=DIRECTION('center_axis',(0.,0.,-1.));
#65582=DIRECTION('ref_axis',(1.,0.,0.));
#65583=DIRECTION('',(0.707106781186546,-8.65956056235491E-17,0.707106781186549));
#65584=DIRECTION('center_axis',(0.,0.,1.));
#65585=DIRECTION('ref_axis',(1.,0.,0.));
#65586=DIRECTION('center_axis',(0.,0.,-1.));
#65587=DIRECTION('ref_axis',(1.,0.,0.));
#65588=DIRECTION('',(0.857167300702112,-1.04972719113862E-16,-0.515038074910054));
#65589=DIRECTION('center_axis',(0.,0.,-1.));
#65590=DIRECTION('ref_axis',(1.,0.,0.));
#65591=DIRECTION('',(0.,0.,-1.));
#65592=DIRECTION('center_axis',(0.,0.,1.));
#65593=DIRECTION('ref_axis',(1.,0.,0.));
#65594=DIRECTION('center_axis',(0.,0.,-1.));
#65595=DIRECTION('ref_axis',(1.,0.,0.));
#65596=DIRECTION('',(0.857167300702112,-1.04972719113862E-16,-0.515038074910054));
#65597=DIRECTION('center_axis',(0.,0.,-1.));
#65598=DIRECTION('ref_axis',(1.,0.,0.));
#65599=DIRECTION('',(0.,0.,-1.));
#65600=DIRECTION('center_axis',(0.,0.,1.));
#65601=DIRECTION('ref_axis',(1.,0.,0.));
#65602=DIRECTION('center_axis',(0.,0.,-1.));
#65603=DIRECTION('ref_axis',(1.,0.,0.));
#65604=DIRECTION('',(0.857167300702112,-1.04972719113862E-16,-0.515038074910054));
#65605=DIRECTION('center_axis',(0.,0.,1.));
#65606=DIRECTION('ref_axis',(1.,0.,0.));
#65607=DIRECTION('',(0.707106781186548,-8.65956056235493E-17,-0.707106781186548));
#65608=DIRECTION('center_axis',(0.,0.,-1.));
#65609=DIRECTION('ref_axis',(1.,0.,0.));
#65610=DIRECTION('center_axis',(0.,0.,-1.));
#65611=DIRECTION('ref_axis',(1.,0.,0.));
#65612=DIRECTION('',(0.,0.,-1.));
#65613=DIRECTION('center_axis',(0.,0.,1.));
#65614=DIRECTION('ref_axis',(1.,0.,0.));
#65615=DIRECTION('center_axis',(0.,0.,-1.));
#65616=DIRECTION('ref_axis',(1.,0.,0.));
#65617=DIRECTION('',(0.857167300702112,-1.04972719113862E-16,-0.515038074910054));
#65618=DIRECTION('center_axis',(0.,0.,1.));
#65619=DIRECTION('ref_axis',(1.,0.,0.));
#65620=DIRECTION('',(0.707106781186548,-8.65956056235493E-17,-0.707106781186548));
#65621=DIRECTION('center_axis',(0.,0.,-1.));
#65622=DIRECTION('ref_axis',(1.,0.,0.));
#65623=DIRECTION('center_axis',(0.,0.,-1.));
#65624=DIRECTION('ref_axis',(1.,0.,0.));
#65625=DIRECTION('',(0.,0.,-1.));
#65626=DIRECTION('center_axis',(0.,0.,1.));
#65627=DIRECTION('ref_axis',(1.,0.,0.));
#65628=DIRECTION('center_axis',(0.,0.,-1.));
#65629=DIRECTION('ref_axis',(1.,0.,0.));
#65630=DIRECTION('',(0.857167300702112,-1.04972719113862E-16,-0.515038074910054));
#65631=DIRECTION('center_axis',(0.,0.,1.));
#65632=DIRECTION('ref_axis',(1.,0.,0.));
#65633=DIRECTION('',(0.707106781186548,-8.65956056235493E-17,-0.707106781186548));
#65634=DIRECTION('center_axis',(0.,0.,-1.));
#65635=DIRECTION('ref_axis',(1.,0.,0.));
#65636=DIRECTION('center_axis',(0.,0.,-1.));
#65637=DIRECTION('ref_axis',(1.,0.,0.));
#65638=DIRECTION('',(0.,0.,-1.));
#65639=DIRECTION('center_axis',(0.,0.,1.));
#65640=DIRECTION('ref_axis',(1.,0.,0.));
#65641=DIRECTION('center_axis',(0.,0.,-1.));
#65642=DIRECTION('ref_axis',(1.,0.,0.));
#65643=DIRECTION('',(0.857167300702112,-1.04972719113862E-16,-0.515038074910054));
#65644=DIRECTION('center_axis',(0.,0.,1.));
#65645=DIRECTION('ref_axis',(1.,0.,0.));
#65646=DIRECTION('',(0.707106781186548,-8.65956056235493E-17,-0.707106781186548));
#65647=DIRECTION('center_axis',(0.,0.,-1.));
#65648=DIRECTION('ref_axis',(1.,0.,0.));
#65649=DIRECTION('center_axis',(0.,0.,-1.));
#65650=DIRECTION('ref_axis',(1.,0.,0.));
#65651=DIRECTION('',(0.,0.,-1.));
#65652=DIRECTION('center_axis',(0.,0.,1.));
#65653=DIRECTION('ref_axis',(1.,0.,0.));
#65654=DIRECTION('center_axis',(0.,0.,1.));
#65655=DIRECTION('ref_axis',(1.,0.,0.));
#65656=DIRECTION('',(0.,0.,1.));
#65657=DIRECTION('center_axis',(0.,0.,1.));
#65658=DIRECTION('ref_axis',(1.,0.,0.));
#65659=DIRECTION('center_axis',(0.,0.,1.));
#65660=DIRECTION('ref_axis',(0.,-1.,0.));
#65661=DIRECTION('',(0.707106781186552,0.,0.707106781186543));
#65662=DIRECTION('center_axis',(0.,0.,-1.));
#65663=DIRECTION('ref_axis',(0.,-1.,0.));
#65664=DIRECTION('',(0.,0.707106781186546,-0.707106781186549));
#65665=DIRECTION('center_axis',(0.707106781186543,0.,-0.707106781186552));
#65666=DIRECTION('ref_axis',(-0.707106781186552,0.,-0.707106781186543));
#65667=DIRECTION('',(0.707106781186552,0.,0.707106781186543));
#65668=DIRECTION('',(0.,-1.,0.));
#65669=DIRECTION('center_axis',(0.,0.,1.));
#65670=DIRECTION('ref_axis',(1.,0.,0.));
#65671=DIRECTION('',(0.,0.707106781186546,0.707106781186549));
#65672=DIRECTION('center_axis',(0.,0.,-1.));
#65673=DIRECTION('ref_axis',(1.,0.,0.));
#65674=DIRECTION('center_axis',(0.,0.707106781186549,-0.707106781186546));
#65675=DIRECTION('ref_axis',(-1.,0.,0.));
#65676=DIRECTION('',(0.,0.707106781186546,0.707106781186549));
#65677=DIRECTION('',(1.,0.,0.));
#65678=DIRECTION('center_axis',(0.,0.,1.));
#65679=DIRECTION('ref_axis',(0.,1.,0.));
#65680=DIRECTION('',(-0.707106781186552,0.,0.707106781186543));
#65681=DIRECTION('center_axis',(0.,0.,-1.));
#65682=DIRECTION('ref_axis',(0.,1.,0.));
#65683=DIRECTION('center_axis',(-0.707106781186543,0.,-0.707106781186552));
#65684=DIRECTION('ref_axis',(-0.707106781186552,0.,0.707106781186543));
#65685=DIRECTION('',(-0.707106781186552,0.,0.707106781186543));
#65686=DIRECTION('',(0.,1.,0.));
#65687=DIRECTION('center_axis',(0.,0.,1.));
#65688=DIRECTION('ref_axis',(-1.,0.,0.));
#65689=DIRECTION('',(0.,-0.707106781186546,0.707106781186549));
#65690=DIRECTION('center_axis',(0.,0.,-1.));
#65691=DIRECTION('ref_axis',(-1.,0.,0.));
#65692=DIRECTION('center_axis',(0.,-0.707106781186549,-0.707106781186546));
#65693=DIRECTION('ref_axis',(-1.,0.,0.));
#65694=DIRECTION('',(-1.,0.,0.));
#65695=DIRECTION('center_axis',(-1.,0.,0.));
#65696=DIRECTION('ref_axis',(0.,-1.,0.));
#65697=DIRECTION('',(0.,0.,1.));
#65698=DIRECTION('',(0.,-1.,0.));
#65699=DIRECTION('',(0.,0.,1.));
#65700=DIRECTION('center_axis',(0.,0.,1.));
#65701=DIRECTION('ref_axis',(-1.,0.,0.));
#65702=DIRECTION('',(0.,0.,1.));
#65703=DIRECTION('center_axis',(0.,0.,1.));
#65704=DIRECTION('ref_axis',(-1.,0.,0.));
#65705=DIRECTION('center_axis',(0.,-1.,0.));
#65706=DIRECTION('ref_axis',(1.,0.,0.));
#65707=DIRECTION('',(0.,0.,1.));
#65708=DIRECTION('',(1.,0.,0.));
#65709=DIRECTION('center_axis',(0.,0.,1.));
#65710=DIRECTION('ref_axis',(0.,-1.,0.));
#65711=DIRECTION('',(0.,0.,1.));
#65712=DIRECTION('center_axis',(0.,0.,1.));
#65713=DIRECTION('ref_axis',(0.,-1.,0.));
#65714=DIRECTION('center_axis',(-0.707106781186549,0.,0.707106781186546));
#65715=DIRECTION('ref_axis',(0.707106781186546,0.,0.707106781186549));
#65716=DIRECTION('',(0.707106781186546,0.,0.707106781186549));
#65717=DIRECTION('',(-0.707106781186546,0.,-0.707106781186549));
#65718=DIRECTION('center_axis',(0.,0.,-1.));
#65719=DIRECTION('ref_axis',(-1.,0.,0.));
#65720=DIRECTION('',(0.,0.707106781186546,0.707106781186549));
#65721=DIRECTION('center_axis',(0.,-0.707106781186549,0.707106781186546));
#65722=DIRECTION('ref_axis',(1.,0.,0.));
#65723=DIRECTION('',(0.,0.707106781186546,0.707106781186549));
#65724=DIRECTION('center_axis',(0.,0.,-1.));
#65725=DIRECTION('ref_axis',(0.,-1.,0.));
#65726=DIRECTION('',(-0.707106781186546,0.,0.707106781186549));
#65727=DIRECTION('center_axis',(0.707106781186549,0.,0.707106781186546));
#65728=DIRECTION('ref_axis',(0.707106781186546,0.,-0.707106781186549));
#65729=DIRECTION('',(-0.707106781186546,0.,0.707106781186549));
#65730=DIRECTION('',(0.,1.,0.));
#65731=DIRECTION('center_axis',(0.,0.,-1.));
#65732=DIRECTION('ref_axis',(1.,0.,0.));
#65733=DIRECTION('',(0.,-0.707106781186546,0.707106781186549));
#65734=DIRECTION('center_axis',(0.,0.,1.));
#65735=DIRECTION('ref_axis',(1.,0.,0.));
#65736=DIRECTION('center_axis',(0.,0.707106781186549,0.707106781186546));
#65737=DIRECTION('ref_axis',(1.,0.,0.));
#65738=DIRECTION('',(0.,-0.707106781186546,0.707106781186549));
#65739=DIRECTION('',(-1.,0.,0.));
#65740=DIRECTION('center_axis',(0.,0.,-1.));
#65741=DIRECTION('ref_axis',(0.,1.,0.));
#65742=DIRECTION('center_axis',(0.,0.,1.));
#65743=DIRECTION('ref_axis',(0.,1.,0.));
#65744=DIRECTION('center_axis',(0.,0.,1.));
#65745=DIRECTION('ref_axis',(0.,1.,0.));
#65746=DIRECTION('',(0.,0.,1.));
#65747=DIRECTION('center_axis',(0.,1.,0.));
#65748=DIRECTION('ref_axis',(-1.,0.,0.));
#65749=DIRECTION('',(0.,0.,1.));
#65750=DIRECTION('center_axis',(0.,0.,1.));
#65751=DIRECTION('ref_axis',(1.,0.,0.));
#65752=DIRECTION('',(0.,0.,1.));
#65753=DIRECTION('center_axis',(1.,0.,0.));
#65754=DIRECTION('ref_axis',(0.,1.,0.));
#80526=CARTESIAN_POINT('',(0.,0.,0.));
#80527=CARTESIAN_POINT('Origin',(28.9568224176764,-54.2987720370293,-0.6));
#80528=CARTESIAN_POINT('',(28.9568224176764,-54.2987720370293,-0.6));
#80529=CARTESIAN_POINT('',(31.0441293939948,-54.2987720370293,-0.6));
#80530=CARTESIAN_POINT('',(14.4784112088382,-54.2987720370293,-0.6));
#80531=CARTESIAN_POINT('',(28.9568224176764,-54.2987720370293,-0.9));
#80532=CARTESIAN_POINT('',(28.9568224176764,-54.2987720370293,-0.6));
#80533=CARTESIAN_POINT('',(31.0441293939948,-54.2987720370293,-0.9));
#80534=CARTESIAN_POINT('',(28.9568224176764,-54.2987720370293,-0.9));
#80535=CARTESIAN_POINT('',(31.0441293939948,-54.2987720370293,-0.6));
#80536=CARTESIAN_POINT('Origin',(28.9568224176764,-53.1414733529091,-0.6));
#80537=CARTESIAN_POINT('',(28.9568224176764,-53.1414733529091,-0.6));
#80538=CARTESIAN_POINT('',(28.9568224176764,-53.0707366764545,-0.6));
#80539=CARTESIAN_POINT('',(28.9568224176764,-53.1414733529091,-0.9));
#80540=CARTESIAN_POINT('',(28.9568224176764,-53.1414733529091,-0.6));
#80541=CARTESIAN_POINT('',(28.9568224176764,-53.1414733529091,-0.9));
#80542=CARTESIAN_POINT('Origin',(30.8377161249518,-53.1414733529091,-0.6));
#80543=CARTESIAN_POINT('',(30.8377161249518,-53.1414733529091,-0.6));
#80544=CARTESIAN_POINT('',(15.4188580624759,-53.1414733529091,-0.6));
#80545=CARTESIAN_POINT('',(30.8377161249518,-53.1414733529091,-0.9));
#80546=CARTESIAN_POINT('',(30.8377161249518,-53.1414733529091,-0.6));
#80547=CARTESIAN_POINT('',(30.8377161249518,-53.1414733529091,-0.9));
#80548=CARTESIAN_POINT('Origin',(30.8377161249518,-52.7425650954247,-0.6));
#80549=CARTESIAN_POINT('',(30.8377161249518,-52.7425650954247,-0.6));
#80550=CARTESIAN_POINT('',(30.8377161249518,-52.8712825477123,-0.6));
#80551=CARTESIAN_POINT('',(30.8377161249518,-52.7425650954247,-0.9));
#80552=CARTESIAN_POINT('',(30.8377161249518,-52.7425650954247,-0.6));
#80553=CARTESIAN_POINT('',(30.8377161249518,-52.7425650954247,-0.9));
#80554=CARTESIAN_POINT('Origin',(28.9568224176764,-52.7425650954247,-0.6));
#80555=CARTESIAN_POINT('',(28.9568224176764,-52.7425650954247,-0.6));
#80556=CARTESIAN_POINT('',(14.4784112088382,-52.7425650954247,-0.6));
#80557=CARTESIAN_POINT('',(28.9568224176764,-52.7425650954247,-0.9));
#80558=CARTESIAN_POINT('',(28.9568224176764,-52.7425650954247,-0.6));
#80559=CARTESIAN_POINT('',(28.9568224176764,-52.7425650954247,-0.9));
#80560=CARTESIAN_POINT('Origin',(28.9568224176764,-51.7012278437614,-0.6));
#80561=CARTESIAN_POINT('',(28.9568224176764,-51.7012278437614,-0.6));
#80562=CARTESIAN_POINT('',(28.9568224176764,-52.3506139218807,-0.6));
#80563=CARTESIAN_POINT('',(28.9568224176764,-51.7012278437614,-0.9));
#80564=CARTESIAN_POINT('',(28.9568224176764,-51.7012278437614,-0.6));
#80565=CARTESIAN_POINT('',(28.9568224176764,-51.7012278437614,-0.9));
#80566=CARTESIAN_POINT('Origin',(30.9652796015143,-51.7012278437614,-0.6));
#80567=CARTESIAN_POINT('',(30.9652796015143,-51.7012278437614,-0.6));
#80568=CARTESIAN_POINT('',(15.4826398007572,-51.7012278437614,-0.6));
#80569=CARTESIAN_POINT('',(30.9652796015143,-51.7012278437614,-0.9));
#80570=CARTESIAN_POINT('',(30.9652796015143,-51.7012278437614,-0.6));
#80571=CARTESIAN_POINT('',(30.9652796015143,-51.7012278437614,-0.9));
#80572=CARTESIAN_POINT('Origin',(30.9652796015143,-51.3000003695488,-0.6));
#80573=CARTESIAN_POINT('',(30.9652796015143,-51.3000003695488,-0.6));
#80574=CARTESIAN_POINT('',(30.9652796015143,-52.1500001847744,-0.6));
#80575=CARTESIAN_POINT('',(30.9652796015143,-51.3000003695488,-0.9));
#80576=CARTESIAN_POINT('',(30.9652796015143,-51.3000003695488,-0.6));
#80577=CARTESIAN_POINT('',(30.9652796015143,-51.3000003695488,-0.9));
#80578=CARTESIAN_POINT('Origin',(28.5068884119391,-51.3000003695488,-0.6));
#80579=CARTESIAN_POINT('',(28.5068884119391,-51.3000003695488,-0.6));
#80580=CARTESIAN_POINT('',(14.2534442059696,-51.3000003695488,-0.6));
#80581=CARTESIAN_POINT('',(28.5068884119391,-51.3000003695488,-0.9));
#80582=CARTESIAN_POINT('',(28.5068884119391,-51.3000003695488,-0.6));
#80583=CARTESIAN_POINT('',(28.5068884119391,-51.3000003695488,-0.9));
#80584=CARTESIAN_POINT('Origin',(28.5068884119391,-54.7000001072884,-0.6));
#80585=CARTESIAN_POINT('',(28.5068884119391,-54.7000001072884,-0.6));
#80586=CARTESIAN_POINT('',(28.5068884119391,-53.8500000536442,-0.6));
#80587=CARTESIAN_POINT('',(28.5068884119391,-54.7000001072884,-0.9));
#80588=CARTESIAN_POINT('',(28.5068884119391,-54.7000001072884,-0.6));
#80589=CARTESIAN_POINT('',(28.5068884119391,-54.7000001072884,-0.9));
#80590=CARTESIAN_POINT('Origin',(31.0441293939948,-54.7000001072884,-0.6));
#80591=CARTESIAN_POINT('',(31.0441293939948,-54.7000001072884,-0.6));
#80592=CARTESIAN_POINT('',(15.5220646969974,-54.7000001072884,-0.6));
#80593=CARTESIAN_POINT('',(31.0441293939948,-54.7000001072884,-0.9));
#80594=CARTESIAN_POINT('',(31.0441293939948,-54.7000001072884,-0.6));
#80595=CARTESIAN_POINT('',(31.0441293939948,-54.7000001072884,-0.9));
#80596=CARTESIAN_POINT('Origin',(31.0441293939948,-54.2987720370293,-0.6));
#80597=CARTESIAN_POINT('',(31.0441293939948,-53.6493860185146,-0.6));
#80598=CARTESIAN_POINT('',(31.0441293939948,-54.2987720370293,-0.9));
#80599=CARTESIAN_POINT('Origin',(29.775508902967,-53.0000002384186,-0.9));
#80600=CARTESIAN_POINT('Origin',(23.8243475183845,-51.3000003695488,-0.6));
#80601=CARTESIAN_POINT('',(23.8243475183845,-51.3000003695488,-0.6));
#80602=CARTESIAN_POINT('',(24.2742815241218,-51.3000003695488,-0.6));
#80603=CARTESIAN_POINT('',(11.9121737591922,-51.3000003695488,-0.6));
#80604=CARTESIAN_POINT('',(23.8243475183845,-51.3000003695488,-0.9));
#80605=CARTESIAN_POINT('',(23.8243475183845,-51.3000003695488,-0.6));
#80606=CARTESIAN_POINT('',(24.2742815241218,-51.3000003695488,-0.9));
#80607=CARTESIAN_POINT('',(23.8243475183845,-51.3000003695488,-0.9));
#80608=CARTESIAN_POINT('',(24.2742815241218,-51.3000003695488,-0.6));
#80609=CARTESIAN_POINT('Origin',(23.8243475183845,-54.7000001072884,-0.6));
#80610=CARTESIAN_POINT('',(23.8243475183845,-54.7000001072884,-0.6));
#80611=CARTESIAN_POINT('',(23.8243475183845,-53.8500000536442,-0.6));
#80612=CARTESIAN_POINT('',(23.8243475183845,-54.7000001072884,-0.9));
#80613=CARTESIAN_POINT('',(23.8243475183845,-54.7000001072884,-0.6));
#80614=CARTESIAN_POINT('',(23.8243475183845,-54.7000001072884,-0.9));
#80615=CARTESIAN_POINT('Origin',(24.2742815241218,-54.7000001072884,-0.6));
#80616=CARTESIAN_POINT('',(24.2742815241218,-54.7000001072884,-0.6));
#80617=CARTESIAN_POINT('',(12.1371407620609,-54.7000001072884,-0.6));
#80618=CARTESIAN_POINT('',(24.2742815241218,-54.7000001072884,-0.9));
#80619=CARTESIAN_POINT('',(24.2742815241218,-54.7000001072884,-0.6));
#80620=CARTESIAN_POINT('',(24.2742815241218,-54.7000001072884,-0.9));
#80621=CARTESIAN_POINT('Origin',(24.2742815241218,-51.3000003695488,-0.6));
#80622=CARTESIAN_POINT('',(24.2742815241218,-52.1500001847744,-0.6));
#80623=CARTESIAN_POINT('',(24.2742815241218,-51.3000003695488,-0.9));
#80624=CARTESIAN_POINT('Origin',(24.0493145212531,-53.0000002384186,-0.9));
#80625=CARTESIAN_POINT('Ctrl Pts',(19.2345800623298,-54.7579811215401,-0.6));
#80626=CARTESIAN_POINT('Ctrl Pts',(19.2345800623298,-54.7579811215401,-0.9));
#80627=CARTESIAN_POINT('Ctrl Pts',(18.773049376905,-54.7579811215401,-0.6));
#80628=CARTESIAN_POINT('Ctrl Pts',(18.773049376905,-54.7579811215401,-0.9));
#80629=CARTESIAN_POINT('Ctrl Pts',(18.4611120447516,-54.623465359211,-0.6));
#80630=CARTESIAN_POINT('Ctrl Pts',(18.4611120447516,-54.623465359211,-0.9));
#80631=CARTESIAN_POINT('',(19.2345800623298,-54.7579811215401,-0.6));
#80632=CARTESIAN_POINT('',(18.4611120447516,-54.623465359211,-0.6));
#80633=CARTESIAN_POINT('Ctrl Pts',(19.2345800623298,-54.7579811215401,-0.6));
#80634=CARTESIAN_POINT('Ctrl Pts',(18.773049376905,-54.7579811215401,-0.6));
#80635=CARTESIAN_POINT('Ctrl Pts',(18.4611120447516,-54.623465359211,-0.6));
#80636=CARTESIAN_POINT('',(19.2345800623298,-54.7579811215401,-0.9));
#80637=CARTESIAN_POINT('',(19.2345800623298,-54.7579811215401,-0.6));
#80638=CARTESIAN_POINT('',(18.4611120447516,-54.623465359211,-0.9));
#80639=CARTESIAN_POINT('Ctrl Pts',(19.2345800623298,-54.7579811215401,-0.9));
#80640=CARTESIAN_POINT('Ctrl Pts',(18.773049376905,-54.7579811215401,-0.9));
#80641=CARTESIAN_POINT('Ctrl Pts',(18.4611120447516,-54.623465359211,-0.9));
#80642=CARTESIAN_POINT('',(18.4611120447516,-54.623465359211,-0.6));
#80643=CARTESIAN_POINT('Ctrl Pts',(19.889763854444,-54.6246246695518,-0.6));
#80644=CARTESIAN_POINT('Ctrl Pts',(19.889763854444,-54.6246246695518,-0.9));
#80645=CARTESIAN_POINT('Ctrl Pts',(19.5987024530768,-54.7579811215401,-0.6));
#80646=CARTESIAN_POINT('Ctrl Pts',(19.5987024530768,-54.7579811215401,-0.9));
#80647=CARTESIAN_POINT('Ctrl Pts',(19.2345800623298,-54.7579811215401,-0.6));
#80648=CARTESIAN_POINT('Ctrl Pts',(19.2345800623298,-54.7579811215401,-0.9));
#80649=CARTESIAN_POINT('',(19.889763854444,-54.6246246695518,-0.6));
#80650=CARTESIAN_POINT('Ctrl Pts',(19.889763854444,-54.6246246695518,-0.6));
#80651=CARTESIAN_POINT('Ctrl Pts',(19.5987024530768,-54.7579811215401,-0.6));
#80652=CARTESIAN_POINT('Ctrl Pts',(19.2345800623298,-54.7579811215401,-0.6));
#80653=CARTESIAN_POINT('',(19.889763854444,-54.6246246695518,-0.9));
#80654=CARTESIAN_POINT('',(19.889763854444,-54.6246246695518,-0.6));
#80655=CARTESIAN_POINT('Ctrl Pts',(19.889763854444,-54.6246246695518,-0.9));
#80656=CARTESIAN_POINT('Ctrl Pts',(19.5987024530768,-54.7579811215401,-0.9));
#80657=CARTESIAN_POINT('Ctrl Pts',(19.2345800623298,-54.7579811215401,-0.9));
#80658=CARTESIAN_POINT('Ctrl Pts',(20.3362169489264,-54.2512277960777,-0.6));
#80659=CARTESIAN_POINT('Ctrl Pts',(20.3362169489264,-54.2512277960777,-0.9));
#80660=CARTESIAN_POINT('Ctrl Pts',(20.1808347925544,-54.4912688136101,-0.6));
#80661=CARTESIAN_POINT('Ctrl Pts',(20.1808347925544,-54.4912688136101,-0.9));
#80662=CARTESIAN_POINT('Ctrl Pts',(19.889763854444,-54.6246246695518,-0.6));
#80663=CARTESIAN_POINT('Ctrl Pts',(19.889763854444,-54.6246246695518,-0.9));
#80664=CARTESIAN_POINT('',(20.3362169489264,-54.2512277960777,-0.6));
#80665=CARTESIAN_POINT('Ctrl Pts',(20.3362169489264,-54.2512277960777,-0.6));
#80666=CARTESIAN_POINT('Ctrl Pts',(20.1808347925544,-54.4912688136101,-0.6));
#80667=CARTESIAN_POINT('Ctrl Pts',(19.889763854444,-54.6246246695518,-0.6));
#80668=CARTESIAN_POINT('',(20.3362169489264,-54.2512277960777,-0.9));
#80669=CARTESIAN_POINT('',(20.3362169489264,-54.2512277960777,-0.6));
#80670=CARTESIAN_POINT('Ctrl Pts',(20.3362169489264,-54.2512277960777,-0.9));
#80671=CARTESIAN_POINT('Ctrl Pts',(20.1808347925544,-54.4912688136101,-0.9));
#80672=CARTESIAN_POINT('Ctrl Pts',(19.889763854444,-54.6246246695518,-0.9));
#80673=CARTESIAN_POINT('Ctrl Pts',(20.4916086420417,-53.7398366332054,-0.6));
#80674=CARTESIAN_POINT('Ctrl Pts',(20.4916086420417,-53.7398366332054,-0.9));
#80675=CARTESIAN_POINT('Ctrl Pts',(20.4916086420417,-54.0111867785454,-0.6));
#80676=CARTESIAN_POINT('Ctrl Pts',(20.4916086420417,-54.0111867785454,-0.9));
#80677=CARTESIAN_POINT('Ctrl Pts',(20.3362169489264,-54.2512277960777,-0.6));
#80678=CARTESIAN_POINT('Ctrl Pts',(20.3362169489264,-54.2512277960777,-0.9));
#80679=CARTESIAN_POINT('',(20.4916086420417,-53.7398366332054,-0.6));
#80680=CARTESIAN_POINT('Ctrl Pts',(20.4916086420417,-53.7398366332054,-0.6));
#80681=CARTESIAN_POINT('Ctrl Pts',(20.4916086420417,-54.0111867785454,-0.6));
#80682=CARTESIAN_POINT('Ctrl Pts',(20.3362169489264,-54.2512277960777,-0.6));
#80683=CARTESIAN_POINT('',(20.4916086420417,-53.7398366332054,-0.9));
#80684=CARTESIAN_POINT('',(20.4916086420417,-53.7398366332054,-0.6));
#80685=CARTESIAN_POINT('Ctrl Pts',(20.4916086420417,-53.7398366332054,-0.9));
#80686=CARTESIAN_POINT('Ctrl Pts',(20.4916086420417,-54.0111867785454,-0.9));
#80687=CARTESIAN_POINT('Ctrl Pts',(20.3362169489264,-54.2512277960777,-0.9));
#80688=CARTESIAN_POINT('Ctrl Pts',(20.3501310572028,-53.2562760710716,-0.6));
#80689=CARTESIAN_POINT('Ctrl Pts',(20.3501310572028,-53.2562760710716,-0.9));
#80690=CARTESIAN_POINT('Ctrl Pts',(20.4916086420417,-53.4661666750908,-0.6));
#80691=CARTESIAN_POINT('Ctrl Pts',(20.4916086420417,-53.4661666750908,-0.9));
#80692=CARTESIAN_POINT('Ctrl Pts',(20.4916086420417,-53.7398366332054,-0.6));
#80693=CARTESIAN_POINT('Ctrl Pts',(20.4916086420417,-53.7398366332054,-0.9));
#80694=CARTESIAN_POINT('',(20.3501310572028,-53.2562760710716,-0.6));
#80695=CARTESIAN_POINT('Ctrl Pts',(20.3501310572028,-53.2562760710716,-0.6));
#80696=CARTESIAN_POINT('Ctrl Pts',(20.4916086420417,-53.4661666750908,-0.6));
#80697=CARTESIAN_POINT('Ctrl Pts',(20.4916086420417,-53.7398366332054,-0.6));
#80698=CARTESIAN_POINT('',(20.3501310572028,-53.2562760710716,-0.9));
#80699=CARTESIAN_POINT('',(20.3501310572028,-53.2562760710716,-0.6));
#80700=CARTESIAN_POINT('Ctrl Pts',(20.3501310572028,-53.2562760710716,-0.9));
#80701=CARTESIAN_POINT('Ctrl Pts',(20.4916086420417,-53.4661666750908,-0.9));
#80702=CARTESIAN_POINT('Ctrl Pts',(20.4916086420417,-53.7398366332054,-0.9));
#80703=CARTESIAN_POINT('Ctrl Pts',(19.9118032678962,-52.9095498919487,-0.6));
#80704=CARTESIAN_POINT('Ctrl Pts',(19.9118032678962,-52.9095498919487,-0.9));
#80705=CARTESIAN_POINT('Ctrl Pts',(20.2086630091071,-53.046384871006,-0.6));
#80706=CARTESIAN_POINT('Ctrl Pts',(20.2086630091071,-53.046384871006,-0.9));
#80707=CARTESIAN_POINT('Ctrl Pts',(20.3501310572028,-53.2562760710716,-0.6));
#80708=CARTESIAN_POINT('Ctrl Pts',(20.3501310572028,-53.2562760710716,-0.9));
#80709=CARTESIAN_POINT('',(19.9118032678962,-52.9095498919487,-0.6));
#80710=CARTESIAN_POINT('Ctrl Pts',(19.9118032678962,-52.9095498919487,-0.6));
#80711=CARTESIAN_POINT('Ctrl Pts',(20.2086630091071,-53.046384871006,-0.6));
#80712=CARTESIAN_POINT('Ctrl Pts',(20.3501310572028,-53.2562760710716,-0.6));
#80713=CARTESIAN_POINT('',(19.9118032678962,-52.9095498919487,-0.9));
#80714=CARTESIAN_POINT('',(19.9118032678962,-52.9095498919487,-0.6));
#80715=CARTESIAN_POINT('Ctrl Pts',(19.9118032678962,-52.9095498919487,-0.9));
#80716=CARTESIAN_POINT('Ctrl Pts',(20.2086630091071,-53.046384871006,-0.9));
#80717=CARTESIAN_POINT('Ctrl Pts',(20.3501310572028,-53.2562760710716,-0.9));
#80718=CARTESIAN_POINT('Ctrl Pts',(19.1592111811042,-52.6927010416985,-0.6));
#80719=CARTESIAN_POINT('Ctrl Pts',(19.1592111811042,-52.6927010416985,-0.9));
#80720=CARTESIAN_POINT('Ctrl Pts',(19.7077074274421,-52.8167806267738,-0.6));
#80721=CARTESIAN_POINT('Ctrl Pts',(19.7077074274421,-52.8167806267738,-0.9));
#80722=CARTESIAN_POINT('Ctrl Pts',(19.9118032678962,-52.9095498919487,-0.6));
#80723=CARTESIAN_POINT('Ctrl Pts',(19.9118032678962,-52.9095498919487,-0.9));
#80724=CARTESIAN_POINT('',(19.1592111811042,-52.6927010416985,-0.6));
#80725=CARTESIAN_POINT('Ctrl Pts',(19.1592111811042,-52.6927010416985,-0.6));
#80726=CARTESIAN_POINT('Ctrl Pts',(19.7077074274421,-52.8167806267738,-0.6));
#80727=CARTESIAN_POINT('Ctrl Pts',(19.9118032678962,-52.9095498919487,-0.6));
#80728=CARTESIAN_POINT('',(19.1592111811042,-52.6927010416985,-0.9));
#80729=CARTESIAN_POINT('',(19.1592111811042,-52.6927010416985,-0.6));
#80730=CARTESIAN_POINT('Ctrl Pts',(19.1592111811042,-52.6927010416985,-0.9));
#80731=CARTESIAN_POINT('Ctrl Pts',(19.7077074274421,-52.8167806267738,-0.9));
#80732=CARTESIAN_POINT('Ctrl Pts',(19.9118032678962,-52.9095498919487,-0.9));
#80733=CARTESIAN_POINT('Ctrl Pts',(18.4808340296149,-52.4503414034843,-0.6));
#80734=CARTESIAN_POINT('Ctrl Pts',(18.4808340296149,-52.4503414034843,-0.9));
#80735=CARTESIAN_POINT('Ctrl Pts',(18.6107053980231,-52.5686220526695,-0.6));
#80736=CARTESIAN_POINT('Ctrl Pts',(18.6107053980231,-52.5686220526695,-0.9));
#80737=CARTESIAN_POINT('Ctrl Pts',(19.1592111811042,-52.6927010416985,-0.6));
#80738=CARTESIAN_POINT('Ctrl Pts',(19.1592111811042,-52.6927010416985,-0.9));
#80739=CARTESIAN_POINT('',(18.4808340296149,-52.4503414034843,-0.6));
#80740=CARTESIAN_POINT('Ctrl Pts',(18.4808340296149,-52.4503414034843,-0.6));
#80741=CARTESIAN_POINT('Ctrl Pts',(18.6107053980231,-52.5686220526695,-0.6));
#80742=CARTESIAN_POINT('Ctrl Pts',(19.1592111811042,-52.6927010416985,-0.6));
#80743=CARTESIAN_POINT('',(18.4808340296149,-52.4503414034843,-0.9));
#80744=CARTESIAN_POINT('',(18.4808340296149,-52.4503414034843,-0.6));
#80745=CARTESIAN_POINT('Ctrl Pts',(18.4808340296149,-52.4503414034843,-0.9));
#80746=CARTESIAN_POINT('Ctrl Pts',(18.6107053980231,-52.5686220526695,-0.9));
#80747=CARTESIAN_POINT('Ctrl Pts',(19.1592111811042,-52.6927010416985,-0.9));
#80748=CARTESIAN_POINT('Ctrl Pts',(18.3486356958747,-52.1488408446312,-0.6));
#80749=CARTESIAN_POINT('Ctrl Pts',(18.3486356958747,-52.1488408446312,-0.9));
#80750=CARTESIAN_POINT('Ctrl Pts',(18.3486356958747,-52.3320601582527,-0.6));
#80751=CARTESIAN_POINT('Ctrl Pts',(18.3486356958747,-52.3320601582527,-0.9));
#80752=CARTESIAN_POINT('Ctrl Pts',(18.4808340296149,-52.4503414034843,-0.6));
#80753=CARTESIAN_POINT('Ctrl Pts',(18.4808340296149,-52.4503414034843,-0.9));
#80754=CARTESIAN_POINT('',(18.3486356958747,-52.1488408446312,-0.6));
#80755=CARTESIAN_POINT('Ctrl Pts',(18.3486356958747,-52.1488408446312,-0.6));
#80756=CARTESIAN_POINT('Ctrl Pts',(18.3486356958747,-52.3320601582527,-0.6));
#80757=CARTESIAN_POINT('Ctrl Pts',(18.4808340296149,-52.4503414034843,-0.6));
#80758=CARTESIAN_POINT('',(18.3486356958747,-52.1488408446312,-0.9));
#80759=CARTESIAN_POINT('',(18.3486356958747,-52.1488408446312,-0.6));
#80760=CARTESIAN_POINT('Ctrl Pts',(18.3486356958747,-52.1488408446312,-0.9));
#80761=CARTESIAN_POINT('Ctrl Pts',(18.3486356958747,-52.3320601582527,-0.9));
#80762=CARTESIAN_POINT('Ctrl Pts',(18.4808340296149,-52.4503414034843,-0.9));
#80763=CARTESIAN_POINT('Ctrl Pts',(18.5353365167975,-51.788199365139,-0.6));
#80764=CARTESIAN_POINT('Ctrl Pts',(18.5353365167975,-51.788199365139,-0.9));
#80765=CARTESIAN_POINT('Ctrl Pts',(18.3486356958747,-51.9377903342247,-0.6));
#80766=CARTESIAN_POINT('Ctrl Pts',(18.3486356958747,-51.9377903342247,-0.9));
#80767=CARTESIAN_POINT('Ctrl Pts',(18.3486356958747,-52.1488408446312,-0.6));
#80768=CARTESIAN_POINT('Ctrl Pts',(18.3486356958747,-52.1488408446312,-0.9));
#80769=CARTESIAN_POINT('',(18.5353365167975,-51.788199365139,-0.6));
#80770=CARTESIAN_POINT('Ctrl Pts',(18.5353365167975,-51.788199365139,-0.6));
#80771=CARTESIAN_POINT('Ctrl Pts',(18.3486356958747,-51.9377903342247,-0.6));
#80772=CARTESIAN_POINT('Ctrl Pts',(18.3486356958747,-52.1488408446312,-0.6));
#80773=CARTESIAN_POINT('',(18.5353365167975,-51.788199365139,-0.9));
#80774=CARTESIAN_POINT('',(18.5353365167975,-51.788199365139,-0.6));
#80775=CARTESIAN_POINT('Ctrl Pts',(18.5353365167975,-51.788199365139,-0.9));
#80776=CARTESIAN_POINT('Ctrl Pts',(18.3486356958747,-51.9377903342247,-0.9));
#80777=CARTESIAN_POINT('Ctrl Pts',(18.3486356958747,-52.1488408446312,-0.9));
#80778=CARTESIAN_POINT('Ctrl Pts',(19.1302194818854,-51.6386083960533,-0.6));
#80779=CARTESIAN_POINT('Ctrl Pts',(19.1302194818854,-51.6386083960533,-0.9));
#80780=CARTESIAN_POINT('Ctrl Pts',(18.7220278009772,-51.6386083960533,-0.6));
#80781=CARTESIAN_POINT('Ctrl Pts',(18.7220278009772,-51.6386083960533,-0.9));
#80782=CARTESIAN_POINT('Ctrl Pts',(18.5353365167975,-51.788199365139,-0.6));
#80783=CARTESIAN_POINT('Ctrl Pts',(18.5353365167975,-51.788199365139,-0.9));
#80784=CARTESIAN_POINT('',(19.1302194818854,-51.6386083960533,-0.6));
#80785=CARTESIAN_POINT('Ctrl Pts',(19.1302194818854,-51.6386083960533,-0.6));
#80786=CARTESIAN_POINT('Ctrl Pts',(18.7220278009772,-51.6386083960533,-0.6));
#80787=CARTESIAN_POINT('Ctrl Pts',(18.5353365167975,-51.788199365139,-0.6));
#80788=CARTESIAN_POINT('',(19.1302194818854,-51.6386083960533,-0.9));
#80789=CARTESIAN_POINT('',(19.1302194818854,-51.6386083960533,-0.6));
#80790=CARTESIAN_POINT('Ctrl Pts',(19.1302194818854,-51.6386083960533,-0.9));
#80791=CARTESIAN_POINT('Ctrl Pts',(18.7220278009772,-51.6386083960533,-0.9));
#80792=CARTESIAN_POINT('Ctrl Pts',(18.5353365167975,-51.788199365139,-0.9));
#80793=CARTESIAN_POINT('Ctrl Pts',(19.7227850183845,-51.8032745718956,-0.6));
#80794=CARTESIAN_POINT('Ctrl Pts',(19.7227850183845,-51.8032745718956,-0.9));
#80795=CARTESIAN_POINT('Ctrl Pts',(19.5221700891852,-51.6386083960533,-0.6));
#80796=CARTESIAN_POINT('Ctrl Pts',(19.5221700891852,-51.6386083960533,-0.9));
#80797=CARTESIAN_POINT('Ctrl Pts',(19.1302194818854,-51.6386083960533,-0.6));
#80798=CARTESIAN_POINT('Ctrl Pts',(19.1302194818854,-51.6386083960533,-0.9));
#80799=CARTESIAN_POINT('',(19.7227850183845,-51.8032745718956,-0.6));
#80800=CARTESIAN_POINT('Ctrl Pts',(19.7227850183845,-51.8032745718956,-0.6));
#80801=CARTESIAN_POINT('Ctrl Pts',(19.5221700891852,-51.6386083960533,-0.6));
#80802=CARTESIAN_POINT('Ctrl Pts',(19.1302194818854,-51.6386083960533,-0.6));
#80803=CARTESIAN_POINT('',(19.7227850183845,-51.8032745718956,-0.9));
#80804=CARTESIAN_POINT('',(19.7227850183845,-51.8032745718956,-0.6));
#80805=CARTESIAN_POINT('Ctrl Pts',(19.7227850183845,-51.8032745718956,-0.9));
#80806=CARTESIAN_POINT('Ctrl Pts',(19.5221700891852,-51.6386083960533,-0.9));
#80807=CARTESIAN_POINT('Ctrl Pts',(19.1302194818854,-51.6386083960533,-0.9));
#80808=CARTESIAN_POINT('Ctrl Pts',(19.958180449903,-52.2903136610985,-0.6));
#80809=CARTESIAN_POINT('Ctrl Pts',(19.958180449903,-52.2903136610985,-0.9));
#80810=CARTESIAN_POINT('Ctrl Pts',(19.9233904108405,-51.9679401516914,-0.6));
#80811=CARTESIAN_POINT('Ctrl Pts',(19.9233904108405,-51.9679401516914,-0.9));
#80812=CARTESIAN_POINT('Ctrl Pts',(19.7227850183845,-51.8032745718956,-0.6));
#80813=CARTESIAN_POINT('Ctrl Pts',(19.7227850183845,-51.8032745718956,-0.9));
#80814=CARTESIAN_POINT('',(19.958180449903,-52.2903136610985,-0.6));
#80815=CARTESIAN_POINT('Ctrl Pts',(19.958180449903,-52.2903136610985,-0.6));
#80816=CARTESIAN_POINT('Ctrl Pts',(19.9233904108405,-51.9679401516914,-0.6));
#80817=CARTESIAN_POINT('Ctrl Pts',(19.7227850183845,-51.8032745718956,-0.6));
#80818=CARTESIAN_POINT('',(19.958180449903,-52.2903136610985,-0.9));
#80819=CARTESIAN_POINT('',(19.958180449903,-52.2903136610985,-0.6));
#80820=CARTESIAN_POINT('Ctrl Pts',(19.958180449903,-52.2903136610985,-0.9));
#80821=CARTESIAN_POINT('Ctrl Pts',(19.9233904108405,-51.9679401516914,-0.9));
#80822=CARTESIAN_POINT('Ctrl Pts',(19.7227850183845,-51.8032745718956,-0.9));
#80823=CARTESIAN_POINT('Origin',(20.3895654901862,-52.2578446269035,-0.6));
#80824=CARTESIAN_POINT('',(20.3895654901862,-52.2578446269035,-0.6));
#80825=CARTESIAN_POINT('',(10.2244394493007,-53.022942611759,-0.6));
#80826=CARTESIAN_POINT('',(20.3895654901862,-52.2578446269035,-0.9));
#80827=CARTESIAN_POINT('',(20.3895654901862,-52.2578446269035,-0.6));
#80828=CARTESIAN_POINT('',(20.3895654901862,-52.2578446269035,-0.9));
#80829=CARTESIAN_POINT('Ctrl Pts',(20.2225771173835,-51.7221013903618,-0.6));
#80830=CARTESIAN_POINT('Ctrl Pts',(20.2225771173835,-51.7221013903618,-0.9));
#80831=CARTESIAN_POINT('Ctrl Pts',(20.3779688104987,-51.9586632847786,-0.6));
#80832=CARTESIAN_POINT('Ctrl Pts',(20.3779688104987,-51.9586632847786,-0.9));
#80833=CARTESIAN_POINT('Ctrl Pts',(20.3895654901862,-52.2578446269035,-0.6));
#80834=CARTESIAN_POINT('Ctrl Pts',(20.3895654901862,-52.2578446269035,-0.9));
#80835=CARTESIAN_POINT('',(20.2225771173835,-51.7221013903618,-0.6));
#80836=CARTESIAN_POINT('Ctrl Pts',(20.2225771173835,-51.7221013903618,-0.6));
#80837=CARTESIAN_POINT('Ctrl Pts',(20.3779688104987,-51.9586632847786,-0.6));
#80838=CARTESIAN_POINT('Ctrl Pts',(20.3895654901862,-52.2578446269035,-0.6));
#80839=CARTESIAN_POINT('',(20.2225771173835,-51.7221013903618,-0.9));
#80840=CARTESIAN_POINT('',(20.2225771173835,-51.7221013903618,-0.6));
#80841=CARTESIAN_POINT('Ctrl Pts',(20.2225771173835,-51.7221013903618,-0.9));
#80842=CARTESIAN_POINT('Ctrl Pts',(20.3779688104987,-51.9586632847786,-0.9));
#80843=CARTESIAN_POINT('Ctrl Pts',(20.3895654901862,-52.2578446269035,-0.9));
#80844=CARTESIAN_POINT('Ctrl Pts',(19.7784414514899,-51.3637797236443,-0.6));
#80845=CARTESIAN_POINT('Ctrl Pts',(19.7784414514899,-51.3637797236443,-0.9));
#80846=CARTESIAN_POINT('Ctrl Pts',(20.0671854242682,-51.4855388998985,-0.6));
#80847=CARTESIAN_POINT('Ctrl Pts',(20.0671854242682,-51.4855388998985,-0.9));
#80848=CARTESIAN_POINT('Ctrl Pts',(20.2225771173835,-51.7221013903618,-0.6));
#80849=CARTESIAN_POINT('Ctrl Pts',(20.2225771173835,-51.7221013903618,-0.9));
#80850=CARTESIAN_POINT('',(19.7784414514899,-51.3637797236443,-0.6));
#80851=CARTESIAN_POINT('Ctrl Pts',(19.7784414514899,-51.3637797236443,-0.6));
#80852=CARTESIAN_POINT('Ctrl Pts',(20.0671854242682,-51.4855388998985,-0.6));
#80853=CARTESIAN_POINT('Ctrl Pts',(20.2225771173835,-51.7221013903618,-0.6));
#80854=CARTESIAN_POINT('',(19.7784414514899,-51.3637797236443,-0.9));
#80855=CARTESIAN_POINT('',(19.7784414514899,-51.3637797236443,-0.6));
#80856=CARTESIAN_POINT('Ctrl Pts',(19.7784414514899,-51.3637797236443,-0.9));
#80857=CARTESIAN_POINT('Ctrl Pts',(20.0671854242682,-51.4855388998985,-0.9));
#80858=CARTESIAN_POINT('Ctrl Pts',(20.2225771173835,-51.7221013903618,-0.9));
#80859=CARTESIAN_POINT('Ctrl Pts',(19.1116609796882,-51.2420193552971,-0.6));
#80860=CARTESIAN_POINT('Ctrl Pts',(19.1116609796882,-51.2420193552971,-0.9));
#80861=CARTESIAN_POINT('Ctrl Pts',(19.4896974787116,-51.2420193552971,-0.6));
#80862=CARTESIAN_POINT('Ctrl Pts',(19.4896974787116,-51.2420193552971,-0.9));
#80863=CARTESIAN_POINT('Ctrl Pts',(19.7784414514899,-51.3637797236443,-0.6));
#80864=CARTESIAN_POINT('Ctrl Pts',(19.7784414514899,-51.3637797236443,-0.9));
#80865=CARTESIAN_POINT('',(19.1116609796882,-51.2420193552971,-0.6));
#80866=CARTESIAN_POINT('Ctrl Pts',(19.1116609796882,-51.2420193552971,-0.6));
#80867=CARTESIAN_POINT('Ctrl Pts',(19.4896974787116,-51.2420193552971,-0.6));
#80868=CARTESIAN_POINT('Ctrl Pts',(19.7784414514899,-51.3637797236443,-0.6));
#80869=CARTESIAN_POINT('',(19.1116609796882,-51.2420193552971,-0.9));
#80870=CARTESIAN_POINT('',(19.1116609796882,-51.2420193552971,-0.6));
#80871=CARTESIAN_POINT('Ctrl Pts',(19.1116609796882,-51.2420193552971,-0.9));
#80872=CARTESIAN_POINT('Ctrl Pts',(19.4896974787116,-51.2420193552971,-0.9));
#80873=CARTESIAN_POINT('Ctrl Pts',(19.7784414514899,-51.3637797236443,-0.9));
#80874=CARTESIAN_POINT('Ctrl Pts',(18.4877863153815,-51.3579813838005,-0.6));
#80875=CARTESIAN_POINT('Ctrl Pts',(18.4877863153815,-51.3579813838005,-0.9));
#80876=CARTESIAN_POINT('Ctrl Pts',(18.7684145197272,-51.2420193552971,-0.6));
#80877=CARTESIAN_POINT('Ctrl Pts',(18.7684145197272,-51.2420193552971,-0.9));
#80878=CARTESIAN_POINT('Ctrl Pts',(19.1116609796882,-51.2420193552971,-0.6));
#80879=CARTESIAN_POINT('Ctrl Pts',(19.1116609796882,-51.2420193552971,-0.9));
#80880=CARTESIAN_POINT('',(18.4877863153815,-51.3579813838005,-0.6));
#80881=CARTESIAN_POINT('Ctrl Pts',(18.4877863153815,-51.3579813838005,-0.6));
#80882=CARTESIAN_POINT('Ctrl Pts',(18.7684145197272,-51.2420193552971,-0.6));
#80883=CARTESIAN_POINT('Ctrl Pts',(19.1116609796882,-51.2420193552971,-0.6));
#80884=CARTESIAN_POINT('',(18.4877863153815,-51.3579813838005,-0.9));
#80885=CARTESIAN_POINT('',(18.4877863153815,-51.3579813838005,-0.6));
#80886=CARTESIAN_POINT('Ctrl Pts',(18.4877863153815,-51.3579813838005,-0.9));
#80887=CARTESIAN_POINT('Ctrl Pts',(18.7684145197272,-51.2420193552971,-0.9));
#80888=CARTESIAN_POINT('Ctrl Pts',(19.1116609796882,-51.2420193552971,-0.9));
#80889=CARTESIAN_POINT('Ctrl Pts',(18.0610456690192,-51.6977493166924,-0.6));
#80890=CARTESIAN_POINT('Ctrl Pts',(18.0610456690192,-51.6977493166924,-0.9));
#80891=CARTESIAN_POINT('Ctrl Pts',(18.2071581110358,-51.4739434123039,-0.6));
#80892=CARTESIAN_POINT('Ctrl Pts',(18.2071581110358,-51.4739434123039,-0.9));
#80893=CARTESIAN_POINT('Ctrl Pts',(18.4877863153815,-51.3579813838005,-0.6));
#80894=CARTESIAN_POINT('Ctrl Pts',(18.4877863153815,-51.3579813838005,-0.9));
#80895=CARTESIAN_POINT('',(18.0610456690192,-51.6977493166924,-0.6));
#80896=CARTESIAN_POINT('Ctrl Pts',(18.0610456690192,-51.6977493166924,-0.6));
#80897=CARTESIAN_POINT('Ctrl Pts',(18.2071581110358,-51.4739434123039,-0.6));
#80898=CARTESIAN_POINT('Ctrl Pts',(18.4877863153815,-51.3579813838005,-0.6));
#80899=CARTESIAN_POINT('',(18.0610456690192,-51.6977493166924,-0.9));
#80900=CARTESIAN_POINT('',(18.0610456690192,-51.6977493166924,-0.6));
#80901=CARTESIAN_POINT('Ctrl Pts',(18.0610456690192,-51.6977493166924,-0.9));
#80902=CARTESIAN_POINT('Ctrl Pts',(18.2071581110358,-51.4739434123039,-0.9));
#80903=CARTESIAN_POINT('Ctrl Pts',(18.4877863153815,-51.3579813838005,-0.9));
#80904=CARTESIAN_POINT('Ctrl Pts',(17.9149332270026,-52.1789906620979,-0.6));
#80905=CARTESIAN_POINT('Ctrl Pts',(17.9149332270026,-52.1789906620979,-0.9));
#80906=CARTESIAN_POINT('Ctrl Pts',(17.9149332270026,-51.9215552210808,-0.6));
#80907=CARTESIAN_POINT('Ctrl Pts',(17.9149332270026,-51.9215552210808,-0.9));
#80908=CARTESIAN_POINT('Ctrl Pts',(18.0610456690192,-51.6977493166924,-0.6));
#80909=CARTESIAN_POINT('Ctrl Pts',(18.0610456690192,-51.6977493166924,-0.9));
#80910=CARTESIAN_POINT('',(17.9149332270026,-52.1789906620979,-0.6));
#80911=CARTESIAN_POINT('Ctrl Pts',(17.9149332270026,-52.1789906620979,-0.6));
#80912=CARTESIAN_POINT('Ctrl Pts',(17.9149332270026,-51.9215552210808,-0.6));
#80913=CARTESIAN_POINT('Ctrl Pts',(18.0610456690192,-51.6977493166924,-0.6));
#80914=CARTESIAN_POINT('',(17.9149332270026,-52.1789906620979,-0.9));
#80915=CARTESIAN_POINT('',(17.9149332270026,-52.1789906620979,-0.6));
#80916=CARTESIAN_POINT('Ctrl Pts',(17.9149332270026,-52.1789906620979,-0.9));
#80917=CARTESIAN_POINT('Ctrl Pts',(17.9149332270026,-51.9215552210808,-0.9));
#80918=CARTESIAN_POINT('Ctrl Pts',(18.0610456690192,-51.6977493166924,-0.9));
#80919=CARTESIAN_POINT('Ctrl Pts',(18.0343809351325,-52.6022509932518,-0.6));
#80920=CARTESIAN_POINT('Ctrl Pts',(18.0343809351325,-52.6022509932518,-0.9));
#80921=CARTESIAN_POINT('Ctrl Pts',(17.9149332270026,-52.4132333397865,-0.6));
#80922=CARTESIAN_POINT('Ctrl Pts',(17.9149332270026,-52.4132333397865,-0.9));
#80923=CARTESIAN_POINT('Ctrl Pts',(17.9149332270026,-52.1789906620979,-0.6));
#80924=CARTESIAN_POINT('Ctrl Pts',(17.9149332270026,-52.1789906620979,-0.9));
#80925=CARTESIAN_POINT('',(18.0343809351325,-52.6022509932518,-0.6));
#80926=CARTESIAN_POINT('Ctrl Pts',(18.0343809351325,-52.6022509932518,-0.6));
#80927=CARTESIAN_POINT('Ctrl Pts',(17.9149332270026,-52.4132333397865,-0.6));
#80928=CARTESIAN_POINT('Ctrl Pts',(17.9149332270026,-52.1789906620979,-0.6));
#80929=CARTESIAN_POINT('',(18.0343809351325,-52.6022509932518,-0.9));
#80930=CARTESIAN_POINT('',(18.0343809351325,-52.6022509932518,-0.6));
#80931=CARTESIAN_POINT('Ctrl Pts',(18.0343809351325,-52.6022509932518,-0.9));
#80932=CARTESIAN_POINT('Ctrl Pts',(17.9149332270026,-52.4132333397865,-0.9));
#80933=CARTESIAN_POINT('Ctrl Pts',(17.9149332270026,-52.1789906620979,-0.9));
#80934=CARTESIAN_POINT('Ctrl Pts',(18.3973398432136,-52.9188267588615,-0.6));
#80935=CARTESIAN_POINT('Ctrl Pts',(18.3973398432136,-52.9188267588615,-0.9));
#80936=CARTESIAN_POINT('Ctrl Pts',(18.1538191065192,-52.7912692427635,-0.6));
#80937=CARTESIAN_POINT('Ctrl Pts',(18.1538191065192,-52.7912692427635,-0.9));
#80938=CARTESIAN_POINT('Ctrl Pts',(18.0343809351325,-52.6022509932518,-0.6));
#80939=CARTESIAN_POINT('Ctrl Pts',(18.0343809351325,-52.6022509932518,-0.9));
#80940=CARTESIAN_POINT('',(18.3973398432136,-52.9188267588615,-0.6));
#80941=CARTESIAN_POINT('Ctrl Pts',(18.3973398432136,-52.9188267588615,-0.6));
#80942=CARTESIAN_POINT('Ctrl Pts',(18.1538191065192,-52.7912692427635,-0.6));
#80943=CARTESIAN_POINT('Ctrl Pts',(18.0343809351325,-52.6022509932518,-0.6));
#80944=CARTESIAN_POINT('',(18.3973398432136,-52.9188267588615,-0.9));
#80945=CARTESIAN_POINT('',(18.3973398432136,-52.9188267588615,-0.6));
#80946=CARTESIAN_POINT('Ctrl Pts',(18.3973398432136,-52.9188267588615,-0.9));
#80947=CARTESIAN_POINT('Ctrl Pts',(18.1538191065192,-52.7912692427635,-0.9));
#80948=CARTESIAN_POINT('Ctrl Pts',(18.0343809351325,-52.6022509932518,-0.9));
#80949=CARTESIAN_POINT('Ctrl Pts',(19.0536775812507,-53.1310371756554,-0.6));
#80950=CARTESIAN_POINT('Ctrl Pts',(19.0536775812507,-53.1310371756554,-0.9));
#80951=CARTESIAN_POINT('Ctrl Pts',(18.5851946100593,-53.018553674221,-0.6));
#80952=CARTESIAN_POINT('Ctrl Pts',(18.5851946100593,-53.018553674221,-0.9));
#80953=CARTESIAN_POINT('Ctrl Pts',(18.3973398432136,-52.9188267588615,-0.6));
#80954=CARTESIAN_POINT('Ctrl Pts',(18.3973398432136,-52.9188267588615,-0.9));
#80955=CARTESIAN_POINT('',(19.0536775812507,-53.1310371756554,-0.6));
#80956=CARTESIAN_POINT('Ctrl Pts',(19.0536775812507,-53.1310371756554,-0.6));
#80957=CARTESIAN_POINT('Ctrl Pts',(18.5851946100593,-53.018553674221,-0.6));
#80958=CARTESIAN_POINT('Ctrl Pts',(18.3973398432136,-52.9188267588615,-0.6));
#80959=CARTESIAN_POINT('',(19.0536775812507,-53.1310371756554,-0.9));
#80960=CARTESIAN_POINT('',(19.0536775812507,-53.1310371756554,-0.6));
#80961=CARTESIAN_POINT('Ctrl Pts',(19.0536775812507,-53.1310371756554,-0.9));
#80962=CARTESIAN_POINT('Ctrl Pts',(18.5851946100593,-53.018553674221,-0.9));
#80963=CARTESIAN_POINT('Ctrl Pts',(18.3973398432136,-52.9188267588615,-0.9));
#80964=CARTESIAN_POINT('Ctrl Pts',(19.6590032801032,-53.2968620657921,-0.6));
#80965=CARTESIAN_POINT('Ctrl Pts',(19.6590032801032,-53.2968620657921,-0.9));
#80966=CARTESIAN_POINT('Ctrl Pts',(19.5221700891852,-53.2435200810432,-0.6));
#80967=CARTESIAN_POINT('Ctrl Pts',(19.5221700891852,-53.2435200810432,-0.9));
#80968=CARTESIAN_POINT('Ctrl Pts',(19.0536775812507,-53.1310371756554,-0.6));
#80969=CARTESIAN_POINT('Ctrl Pts',(19.0536775812507,-53.1310371756554,-0.9));
#80970=CARTESIAN_POINT('',(19.6590032801032,-53.2968620657921,-0.6));
#80971=CARTESIAN_POINT('Ctrl Pts',(19.6590032801032,-53.2968620657921,-0.6));
#80972=CARTESIAN_POINT('Ctrl Pts',(19.5221700891852,-53.2435200810432,-0.6));
#80973=CARTESIAN_POINT('Ctrl Pts',(19.0536775812507,-53.1310371756554,-0.6));
#80974=CARTESIAN_POINT('',(19.6590032801032,-53.2968620657921,-0.9));
#80975=CARTESIAN_POINT('',(19.6590032801032,-53.2968620657921,-0.6));
#80976=CARTESIAN_POINT('Ctrl Pts',(19.6590032801032,-53.2968620657921,-0.9));
#80977=CARTESIAN_POINT('Ctrl Pts',(19.5221700891852,-53.2435200810432,-0.9));
#80978=CARTESIAN_POINT('Ctrl Pts',(19.0536775812507,-53.1310371756554,-0.9));
#80979=CARTESIAN_POINT('Ctrl Pts',(19.9651422724128,-53.4974763989449,-0.6));
#80980=CARTESIAN_POINT('Ctrl Pts',(19.9651422724128,-53.4974763989449,-0.9));
#80981=CARTESIAN_POINT('Ctrl Pts',(19.8723688349128,-53.3780352473259,-0.6));
#80982=CARTESIAN_POINT('Ctrl Pts',(19.8723688349128,-53.3780352473259,-0.9));
#80983=CARTESIAN_POINT('Ctrl Pts',(19.6590032801032,-53.2968620657921,-0.6));
#80984=CARTESIAN_POINT('Ctrl Pts',(19.6590032801032,-53.2968620657921,-0.9));
#80985=CARTESIAN_POINT('',(19.9651422724128,-53.4974763989449,-0.6));
#80986=CARTESIAN_POINT('Ctrl Pts',(19.9651422724128,-53.4974763989449,-0.6));
#80987=CARTESIAN_POINT('Ctrl Pts',(19.8723688349128,-53.3780352473259,-0.6));
#80988=CARTESIAN_POINT('Ctrl Pts',(19.6590032801032,-53.2968620657921,-0.6));
#80989=CARTESIAN_POINT('',(19.9651422724128,-53.4974763989449,-0.9));
#80990=CARTESIAN_POINT('',(19.9651422724128,-53.4974763989449,-0.6));
#80991=CARTESIAN_POINT('Ctrl Pts',(19.9651422724128,-53.4974763989449,-0.9));
#80992=CARTESIAN_POINT('Ctrl Pts',(19.8723688349128,-53.3780352473259,-0.9));
#80993=CARTESIAN_POINT('Ctrl Pts',(19.6590032801032,-53.2968620657921,-0.9));
#80994=CARTESIAN_POINT('Ctrl Pts',(20.0579061731696,-53.7769441008568,-0.6));
#80995=CARTESIAN_POINT('Ctrl Pts',(20.0579061731696,-53.7769441008568,-0.9));
#80996=CARTESIAN_POINT('Ctrl Pts',(20.0579061731696,-53.6169169545174,-0.6));
#80997=CARTESIAN_POINT('Ctrl Pts',(20.0579061731696,-53.6169169545174,-0.9));
#80998=CARTESIAN_POINT('Ctrl Pts',(19.9651422724128,-53.4974763989449,-0.6));
#80999=CARTESIAN_POINT('Ctrl Pts',(19.9651422724128,-53.4974763989449,-0.9));
#81000=CARTESIAN_POINT('',(20.0579061731696,-53.7769441008568,-0.6));
#81001=CARTESIAN_POINT('Ctrl Pts',(20.0579061731696,-53.7769441008568,-0.6));
#81002=CARTESIAN_POINT('Ctrl Pts',(20.0579061731696,-53.6169169545174,-0.6));
#81003=CARTESIAN_POINT('Ctrl Pts',(19.9651422724128,-53.4974763989449,-0.6));
#81004=CARTESIAN_POINT('',(20.0579061731696,-53.7769441008568,-0.9));
#81005=CARTESIAN_POINT('',(20.0579061731696,-53.7769441008568,-0.6));
#81006=CARTESIAN_POINT('Ctrl Pts',(20.0579061731696,-53.7769441008568,-0.9));
#81007=CARTESIAN_POINT('Ctrl Pts',(20.0579061731696,-53.6169169545174,-0.9));
#81008=CARTESIAN_POINT('Ctrl Pts',(19.9651422724128,-53.4974763989449,-0.9));
#81009=CARTESIAN_POINT('Ctrl Pts',(19.9616613611579,-54.0680084824562,-0.6));
#81010=CARTESIAN_POINT('Ctrl Pts',(19.9616613611579,-54.0680084824562,-0.9));
#81011=CARTESIAN_POINT('Ctrl Pts',(20.0579061731696,-53.934652030468,-0.6));
#81012=CARTESIAN_POINT('Ctrl Pts',(20.0579061731696,-53.934652030468,-0.9));
#81013=CARTESIAN_POINT('Ctrl Pts',(20.0579061731696,-53.7769441008568,-0.6));
#81014=CARTESIAN_POINT('Ctrl Pts',(20.0579061731696,-53.7769441008568,-0.9));
#81015=CARTESIAN_POINT('',(19.9616613611579,-54.0680084824562,-0.6));
#81016=CARTESIAN_POINT('Ctrl Pts',(19.9616613611579,-54.0680084824562,-0.6));
#81017=CARTESIAN_POINT('Ctrl Pts',(20.0579061731696,-53.934652030468,-0.6));
#81018=CARTESIAN_POINT('Ctrl Pts',(20.0579061731696,-53.7769441008568,-0.6));
#81019=CARTESIAN_POINT('',(19.9616613611579,-54.0680084824562,-0.9));
#81020=CARTESIAN_POINT('',(19.9616613611579,-54.0680084824562,-0.6));
#81021=CARTESIAN_POINT('Ctrl Pts',(19.9616613611579,-54.0680084824562,-0.9));
#81022=CARTESIAN_POINT('Ctrl Pts',(20.0579061731696,-53.934652030468,-0.9));
#81023=CARTESIAN_POINT('Ctrl Pts',(20.0579061731696,-53.7769441008568,-0.9));
#81024=CARTESIAN_POINT('Ctrl Pts',(19.6682825312018,-54.2778990864754,-0.6));
#81025=CARTESIAN_POINT('Ctrl Pts',(19.6682825312018,-54.2778990864754,-0.9));
#81026=CARTESIAN_POINT('Ctrl Pts',(19.8654165491462,-54.201364338398,-0.6));
#81027=CARTESIAN_POINT('Ctrl Pts',(19.8654165491462,-54.201364338398,-0.9));
#81028=CARTESIAN_POINT('Ctrl Pts',(19.9616613611579,-54.0680084824562,-0.6));
#81029=CARTESIAN_POINT('Ctrl Pts',(19.9616613611579,-54.0680084824562,-0.9));
#81030=CARTESIAN_POINT('',(19.6682825312018,-54.2778990864754,-0.6));
#81031=CARTESIAN_POINT('Ctrl Pts',(19.6682825312018,-54.2778990864754,-0.6));
#81032=CARTESIAN_POINT('Ctrl Pts',(19.8654165491462,-54.201364338398,-0.6));
#81033=CARTESIAN_POINT('Ctrl Pts',(19.9616613611579,-54.0680084824562,-0.6));
#81034=CARTESIAN_POINT('',(19.6682825312018,-54.2778990864754,-0.9));
#81035=CARTESIAN_POINT('',(19.6682825312018,-54.2778990864754,-0.6));
#81036=CARTESIAN_POINT('Ctrl Pts',(19.6682825312018,-54.2778990864754,-0.9));
#81037=CARTESIAN_POINT('Ctrl Pts',(19.8654165491462,-54.201364338398,-0.9));
#81038=CARTESIAN_POINT('Ctrl Pts',(19.9616613611579,-54.0680084824562,-0.9));
#81039=CARTESIAN_POINT('Ctrl Pts',(19.2137041315436,-54.3544338345528,-0.6));
#81040=CARTESIAN_POINT('Ctrl Pts',(19.2137041315436,-54.3544338345528,-0.9));
#81041=CARTESIAN_POINT('Ctrl Pts',(19.4711485132575,-54.3544338345528,-0.6));
#81042=CARTESIAN_POINT('Ctrl Pts',(19.4711485132575,-54.3544338345528,-0.9));
#81043=CARTESIAN_POINT('Ctrl Pts',(19.6682825312018,-54.2778990864754,-0.6));
#81044=CARTESIAN_POINT('Ctrl Pts',(19.6682825312018,-54.2778990864754,-0.9));
#81045=CARTESIAN_POINT('',(19.2137041315436,-54.3544338345528,-0.6));
#81046=CARTESIAN_POINT('Ctrl Pts',(19.2137041315436,-54.3544338345528,-0.6));
#81047=CARTESIAN_POINT('Ctrl Pts',(19.4711485132575,-54.3544338345528,-0.6));
#81048=CARTESIAN_POINT('Ctrl Pts',(19.6682825312018,-54.2778990864754,-0.6));
#81049=CARTESIAN_POINT('',(19.2137041315436,-54.3544338345528,-0.9));
#81050=CARTESIAN_POINT('',(19.2137041315436,-54.3544338345528,-0.6));
#81051=CARTESIAN_POINT('Ctrl Pts',(19.2137041315436,-54.3544338345528,-0.9));
#81052=CARTESIAN_POINT('Ctrl Pts',(19.4711485132575,-54.3544338345528,-0.9));
#81053=CARTESIAN_POINT('Ctrl Pts',(19.6682825312018,-54.2778990864754,-0.9));
#81054=CARTESIAN_POINT('Ctrl Pts',(18.6918821558356,-54.2535470128059,-0.6));
#81055=CARTESIAN_POINT('Ctrl Pts',(18.6918821558356,-54.2535470128059,-0.9));
#81056=CARTESIAN_POINT('Ctrl Pts',(18.9238062128425,-54.3544338345528,-0.6));
#81057=CARTESIAN_POINT('Ctrl Pts',(18.9238062128425,-54.3544338345528,-0.9));
#81058=CARTESIAN_POINT('Ctrl Pts',(19.2137041315436,-54.3544338345528,-0.6));
#81059=CARTESIAN_POINT('Ctrl Pts',(19.2137041315436,-54.3544338345528,-0.9));
#81060=CARTESIAN_POINT('',(18.6918821558356,-54.2535470128059,-0.6));
#81061=CARTESIAN_POINT('Ctrl Pts',(18.6918821558356,-54.2535470128059,-0.6));
#81062=CARTESIAN_POINT('Ctrl Pts',(18.9238062128425,-54.3544338345528,-0.6));
#81063=CARTESIAN_POINT('Ctrl Pts',(19.2137041315436,-54.3544338345528,-0.6));
#81064=CARTESIAN_POINT('',(18.6918821558356,-54.2535470128059,-0.9));
#81065=CARTESIAN_POINT('',(18.6918821558356,-54.2535470128059,-0.6));
#81066=CARTESIAN_POINT('Ctrl Pts',(18.6918821558356,-54.2535470128059,-0.9));
#81067=CARTESIAN_POINT('Ctrl Pts',(18.9238062128425,-54.3544338345528,-0.9));
#81068=CARTESIAN_POINT('Ctrl Pts',(19.2137041315436,-54.3544338345528,-0.9));
#81069=CARTESIAN_POINT('Ctrl Pts',(18.3497896417975,-53.9891545176506,-0.6));
#81070=CARTESIAN_POINT('Ctrl Pts',(18.3497896417975,-53.9891545176506,-0.9));
#81071=CARTESIAN_POINT('Ctrl Pts',(18.4599580988288,-54.1526601910591,-0.6));
#81072=CARTESIAN_POINT('Ctrl Pts',(18.4599580988288,-54.1526601910591,-0.9));
#81073=CARTESIAN_POINT('Ctrl Pts',(18.6918821558356,-54.2535470128059,-0.6));
#81074=CARTESIAN_POINT('Ctrl Pts',(18.6918821558356,-54.2535470128059,-0.9));
#81075=CARTESIAN_POINT('',(18.3497896417975,-53.9891545176506,-0.6));
#81076=CARTESIAN_POINT('Ctrl Pts',(18.3497896417975,-53.9891545176506,-0.6));
#81077=CARTESIAN_POINT('Ctrl Pts',(18.4599580988288,-54.1526601910591,-0.6));
#81078=CARTESIAN_POINT('Ctrl Pts',(18.6918821558356,-54.2535470128059,-0.6));
#81079=CARTESIAN_POINT('',(18.3497896417975,-53.9891545176506,-0.9));
#81080=CARTESIAN_POINT('',(18.3497896417975,-53.9891545176506,-0.6));
#81081=CARTESIAN_POINT('Ctrl Pts',(18.3497896417975,-53.9891545176506,-0.9));
#81082=CARTESIAN_POINT('Ctrl Pts',(18.4599580988288,-54.1526601910591,-0.9));
#81083=CARTESIAN_POINT('Ctrl Pts',(18.6918821558356,-54.2535470128059,-0.9));
#81084=CARTESIAN_POINT('Ctrl Pts',(18.2094755396247,-53.5705320239067,-0.6));
#81085=CARTESIAN_POINT('Ctrl Pts',(18.2094755396247,-53.5705320239067,-0.9));
#81086=CARTESIAN_POINT('Ctrl Pts',(18.2396307215095,-53.8256482481956,-0.6));
#81087=CARTESIAN_POINT('Ctrl Pts',(18.2396307215095,-53.8256482481956,-0.9));
#81088=CARTESIAN_POINT('Ctrl Pts',(18.3497896417975,-53.9891545176506,-0.6));
#81089=CARTESIAN_POINT('Ctrl Pts',(18.3497896417975,-53.9891545176506,-0.9));
#81090=CARTESIAN_POINT('',(18.2094755396247,-53.5705320239067,-0.6));
#81091=CARTESIAN_POINT('Ctrl Pts',(18.2094755396247,-53.5705320239067,-0.6));
#81092=CARTESIAN_POINT('Ctrl Pts',(18.2396307215095,-53.8256482481956,-0.6));
#81093=CARTESIAN_POINT('Ctrl Pts',(18.3497896417975,-53.9891545176506,-0.6));
#81094=CARTESIAN_POINT('',(18.2094755396247,-53.5705320239067,-0.9));
#81095=CARTESIAN_POINT('',(18.2094755396247,-53.5705320239067,-0.6));
#81096=CARTESIAN_POINT('Ctrl Pts',(18.2094755396247,-53.5705320239067,-0.9));
#81097=CARTESIAN_POINT('Ctrl Pts',(18.2396307215095,-53.8256482481956,-0.9));
#81098=CARTESIAN_POINT('Ctrl Pts',(18.3497896417975,-53.9891545176506,-0.9));
#81099=CARTESIAN_POINT('Origin',(17.7850618585944,-53.6076400876045,-0.6));
#81100=CARTESIAN_POINT('',(17.7850618585944,-53.6076400876045,-0.6));
#81101=CARTESIAN_POINT('',(8.98635809002947,-54.3769434218173,-0.6));
#81102=CARTESIAN_POINT('',(17.7850618585944,-53.6076400876045,-0.9));
#81103=CARTESIAN_POINT('',(17.7850618585944,-53.6076400876045,-0.6));
#81104=CARTESIAN_POINT('',(17.7850618585944,-53.6076400876045,-0.9));
#81105=CARTESIAN_POINT('Ctrl Pts',(17.9717626795173,-54.2187587618828,-0.6));
#81106=CARTESIAN_POINT('Ctrl Pts',(17.9717626795173,-54.2187587618828,-0.9));
#81107=CARTESIAN_POINT('Ctrl Pts',(17.7943411096931,-53.9485673308372,-0.6));
#81108=CARTESIAN_POINT('Ctrl Pts',(17.7943411096931,-53.9485673308372,-0.9));
#81109=CARTESIAN_POINT('Ctrl Pts',(17.7850618585944,-53.6076400876045,-0.6));
#81110=CARTESIAN_POINT('Ctrl Pts',(17.7850618585944,-53.6076400876045,-0.9));
#81111=CARTESIAN_POINT('',(17.9717626795173,-54.2187587618828,-0.6));
#81112=CARTESIAN_POINT('Ctrl Pts',(17.9717626795173,-54.2187587618828,-0.6));
#81113=CARTESIAN_POINT('Ctrl Pts',(17.7943411096931,-53.9485673308372,-0.6));
#81114=CARTESIAN_POINT('Ctrl Pts',(17.7850618585944,-53.6076400876045,-0.6));
#81115=CARTESIAN_POINT('',(17.9717626795173,-54.2187587618828,-0.9));
#81116=CARTESIAN_POINT('',(17.9717626795173,-54.2187587618828,-0.6));
#81117=CARTESIAN_POINT('Ctrl Pts',(17.9717626795173,-54.2187587618828,-0.9));
#81118=CARTESIAN_POINT('Ctrl Pts',(17.7943411096931,-53.9485673308372,-0.9));
#81119=CARTESIAN_POINT('Ctrl Pts',(17.7850618585944,-53.6076400876045,-0.9));
#81120=CARTESIAN_POINT('Ctrl Pts',(18.4611120447516,-54.623465359211,-0.6));
#81121=CARTESIAN_POINT('Ctrl Pts',(18.4611120447516,-54.623465359211,-0.9));
#81122=CARTESIAN_POINT('Ctrl Pts',(18.1491842493415,-54.4889495968819,-0.6));
#81123=CARTESIAN_POINT('Ctrl Pts',(18.1491842493415,-54.4889495968819,-0.9));
#81124=CARTESIAN_POINT('Ctrl Pts',(17.9717626795173,-54.2187587618828,-0.6));
#81125=CARTESIAN_POINT('Ctrl Pts',(17.9717626795173,-54.2187587618828,-0.9));
#81126=CARTESIAN_POINT('Ctrl Pts',(18.4611120447516,-54.623465359211,-0.6));
#81127=CARTESIAN_POINT('Ctrl Pts',(18.1491842493415,-54.4889495968819,-0.6));
#81128=CARTESIAN_POINT('Ctrl Pts',(17.9717626795173,-54.2187587618828,-0.6));
#81129=CARTESIAN_POINT('Ctrl Pts',(18.4611120447516,-54.623465359211,-0.9));
#81130=CARTESIAN_POINT('Ctrl Pts',(18.1491842493415,-54.4889495968819,-0.9));
#81131=CARTESIAN_POINT('Ctrl Pts',(17.9717626795173,-54.2187587618828,-0.9));
#81132=CARTESIAN_POINT('Origin',(19.1383352503181,-53.0000002384186,-0.9));
#81133=CARTESIAN_POINT('Ctrl Pts',(10.8737364038825,-54.212960422039,-0.6));
#81134=CARTESIAN_POINT('Ctrl Pts',(10.8737364038825,-54.212960422039,-0.9));
#81135=CARTESIAN_POINT('Ctrl Pts',(11.1404504999518,-54.3729875683784,-0.6));
#81136=CARTESIAN_POINT('Ctrl Pts',(11.1404504999518,-54.3729875683784,-0.9));
#81137=CARTESIAN_POINT('Ctrl Pts',(11.4512243494391,-54.3729875683784,-0.6));
#81138=CARTESIAN_POINT('Ctrl Pts',(11.4512243494391,-54.3729875683784,-0.9));
#81139=CARTESIAN_POINT('',(10.8737364038825,-54.212960422039,-0.6));
#81140=CARTESIAN_POINT('',(11.4512243494391,-54.3729875683784,-0.6));
#81141=CARTESIAN_POINT('Ctrl Pts',(10.8737364038825,-54.212960422039,-0.6));
#81142=CARTESIAN_POINT('Ctrl Pts',(11.1404504999518,-54.3729875683784,-0.6));
#81143=CARTESIAN_POINT('Ctrl Pts',(11.4512243494391,-54.3729875683784,-0.6));
#81144=CARTESIAN_POINT('',(10.8737364038825,-54.212960422039,-0.9));
#81145=CARTESIAN_POINT('',(10.8737364038825,-54.212960422039,-0.6));
#81146=CARTESIAN_POINT('',(11.4512243494391,-54.3729875683784,-0.9));
#81147=CARTESIAN_POINT('Ctrl Pts',(10.8737364038825,-54.212960422039,-0.9));
#81148=CARTESIAN_POINT('Ctrl Pts',(11.1404504999518,-54.3729875683784,-0.9));
#81149=CARTESIAN_POINT('Ctrl Pts',(11.4512243494391,-54.3729875683784,-0.9));
#81150=CARTESIAN_POINT('',(11.4512243494391,-54.3729875683784,-0.6));
#81151=CARTESIAN_POINT('Ctrl Pts',(10.4806223139167,-53.7293998599052,-0.6));
#81152=CARTESIAN_POINT('Ctrl Pts',(10.4806223139167,-53.7293998599052,-0.9));
#81153=CARTESIAN_POINT('Ctrl Pts',(10.6070223078132,-54.0529332756996,-0.6));
#81154=CARTESIAN_POINT('Ctrl Pts',(10.6070223078132,-54.0529332756996,-0.9));
#81155=CARTESIAN_POINT('Ctrl Pts',(10.8737364038825,-54.212960422039,-0.6));
#81156=CARTESIAN_POINT('Ctrl Pts',(10.8737364038825,-54.212960422039,-0.9));
#81157=CARTESIAN_POINT('',(10.4806223139167,-53.7293998599052,-0.6));
#81158=CARTESIAN_POINT('Ctrl Pts',(10.4806223139167,-53.7293998599052,-0.6));
#81159=CARTESIAN_POINT('Ctrl Pts',(10.6070223078132,-54.0529332756996,-0.6));
#81160=CARTESIAN_POINT('Ctrl Pts',(10.8737364038825,-54.212960422039,-0.6));
#81161=CARTESIAN_POINT('',(10.4806223139167,-53.7293998599052,-0.9));
#81162=CARTESIAN_POINT('',(10.4806223139167,-53.7293998599052,-0.6));
#81163=CARTESIAN_POINT('Ctrl Pts',(10.4806223139167,-53.7293998599052,-0.9));
#81164=CARTESIAN_POINT('Ctrl Pts',(10.6070223078132,-54.0529332756996,-0.9));
#81165=CARTESIAN_POINT('Ctrl Pts',(10.8737364038825,-54.212960422039,-0.9));
#81166=CARTESIAN_POINT('Ctrl Pts',(10.3542318567634,-52.9721693396568,-0.6));
#81167=CARTESIAN_POINT('Ctrl Pts',(10.3542318567634,-52.9721693396568,-0.9));
#81168=CARTESIAN_POINT('Ctrl Pts',(10.3542318567634,-53.4058664441109,-0.6));
#81169=CARTESIAN_POINT('Ctrl Pts',(10.3542318567634,-53.4058664441109,-0.9));
#81170=CARTESIAN_POINT('Ctrl Pts',(10.4806223139167,-53.7293998599052,-0.6));
#81171=CARTESIAN_POINT('Ctrl Pts',(10.4806223139167,-53.7293998599052,-0.9));
#81172=CARTESIAN_POINT('',(10.3542318567634,-52.9721693396568,-0.6));
#81173=CARTESIAN_POINT('Ctrl Pts',(10.3542318567634,-52.9721693396568,-0.6));
#81174=CARTESIAN_POINT('Ctrl Pts',(10.3542318567634,-53.4058664441109,-0.6));
#81175=CARTESIAN_POINT('Ctrl Pts',(10.4806223139167,-53.7293998599052,-0.6));
#81176=CARTESIAN_POINT('',(10.3542318567634,-52.9721693396568,-0.9));
#81177=CARTESIAN_POINT('',(10.3542318567634,-52.9721693396568,-0.6));
#81178=CARTESIAN_POINT('Ctrl Pts',(10.3542318567634,-52.9721693396568,-0.9));
#81179=CARTESIAN_POINT('Ctrl Pts',(10.3542318567634,-53.4058664441109,-0.9));
#81180=CARTESIAN_POINT('Ctrl Pts',(10.4806223139167,-53.7293998599052,-0.9));
#81181=CARTESIAN_POINT('Ctrl Pts',(10.4609098657966,-52.3193041682243,-0.6));
#81182=CARTESIAN_POINT('Ctrl Pts',(10.4609098657966,-52.3193041682243,-0.9));
#81183=CARTESIAN_POINT('Ctrl Pts',(10.3542318567634,-52.6358799338341,-0.6));
#81184=CARTESIAN_POINT('Ctrl Pts',(10.3542318567634,-52.6358799338341,-0.9));
#81185=CARTESIAN_POINT('Ctrl Pts',(10.3542318567634,-52.9721693396568,-0.6));
#81186=CARTESIAN_POINT('Ctrl Pts',(10.3542318567634,-52.9721693396568,-0.9));
#81187=CARTESIAN_POINT('',(10.4609098657966,-52.3193041682243,-0.6));
#81188=CARTESIAN_POINT('Ctrl Pts',(10.4609098657966,-52.3193041682243,-0.6));
#81189=CARTESIAN_POINT('Ctrl Pts',(10.3542318567634,-52.6358799338341,-0.6));
#81190=CARTESIAN_POINT('Ctrl Pts',(10.3542318567634,-52.9721693396568,-0.6));
#81191=CARTESIAN_POINT('',(10.4609098657966,-52.3193041682243,-0.9));
#81192=CARTESIAN_POINT('',(10.4609098657966,-52.3193041682243,-0.6));
#81193=CARTESIAN_POINT('Ctrl Pts',(10.4609098657966,-52.3193041682243,-0.9));
#81194=CARTESIAN_POINT('Ctrl Pts',(10.3542318567634,-52.6358799338341,-0.9));
#81195=CARTESIAN_POINT('Ctrl Pts',(10.3542318567634,-52.9721693396568,-0.9));
#81196=CARTESIAN_POINT('Ctrl Pts',(10.8308305963874,-51.8148706555367,-0.6));
#81197=CARTESIAN_POINT('Ctrl Pts',(10.8308305963874,-51.8148706555367,-0.9));
#81198=CARTESIAN_POINT('Ctrl Pts',(10.5675974115729,-52.0027284026146,-0.6));
#81199=CARTESIAN_POINT('Ctrl Pts',(10.5675974115729,-52.0027284026146,-0.9));
#81200=CARTESIAN_POINT('Ctrl Pts',(10.4609098657966,-52.3193041682243,-0.6));
#81201=CARTESIAN_POINT('Ctrl Pts',(10.4609098657966,-52.3193041682243,-0.9));
#81202=CARTESIAN_POINT('',(10.8308305963874,-51.8148706555367,-0.6));
#81203=CARTESIAN_POINT('Ctrl Pts',(10.8308305963874,-51.8148706555367,-0.6));
#81204=CARTESIAN_POINT('Ctrl Pts',(10.5675974115729,-52.0027284026146,-0.6));
#81205=CARTESIAN_POINT('Ctrl Pts',(10.4609098657966,-52.3193041682243,-0.6));
#81206=CARTESIAN_POINT('',(10.8308305963874,-51.8148706555367,-0.9));
#81207=CARTESIAN_POINT('',(10.8308305963874,-51.8148706555367,-0.6));
#81208=CARTESIAN_POINT('Ctrl Pts',(10.8308305963874,-51.8148706555367,-0.9));
#81209=CARTESIAN_POINT('Ctrl Pts',(10.5675974115729,-52.0027284026146,-0.9));
#81210=CARTESIAN_POINT('Ctrl Pts',(10.4609098657966,-52.3193041682243,-0.9));
#81211=CARTESIAN_POINT('Ctrl Pts',(11.4860143885016,-51.6270129084587,-0.6));
#81212=CARTESIAN_POINT('Ctrl Pts',(11.4860143885016,-51.6270129084587,-0.9));
#81213=CARTESIAN_POINT('Ctrl Pts',(11.0940637812018,-51.6270129084587,-0.6));
#81214=CARTESIAN_POINT('Ctrl Pts',(11.0940637812018,-51.6270129084587,-0.9));
#81215=CARTESIAN_POINT('Ctrl Pts',(10.8308305963874,-51.8148706555367,-0.6));
#81216=CARTESIAN_POINT('Ctrl Pts',(10.8308305963874,-51.8148706555367,-0.9));
#81217=CARTESIAN_POINT('',(11.4860143885016,-51.6270129084587,-0.6));
#81218=CARTESIAN_POINT('Ctrl Pts',(11.4860143885016,-51.6270129084587,-0.6));
#81219=CARTESIAN_POINT('Ctrl Pts',(11.0940637812018,-51.6270129084587,-0.6));
#81220=CARTESIAN_POINT('Ctrl Pts',(10.8308305963874,-51.8148706555367,-0.6));
#81221=CARTESIAN_POINT('',(11.4860143885016,-51.6270129084587,-0.9));
#81222=CARTESIAN_POINT('',(11.4860143885016,-51.6270129084587,-0.6));
#81223=CARTESIAN_POINT('Ctrl Pts',(11.4860143885016,-51.6270129084587,-0.9));
#81224=CARTESIAN_POINT('Ctrl Pts',(11.0940637812018,-51.6270129084587,-0.9));
#81225=CARTESIAN_POINT('Ctrl Pts',(10.8308305963874,-51.8148706555367,-0.9));
#81226=CARTESIAN_POINT('Ctrl Pts',(12.0519056543708,-51.796316921711,-0.6));
#81227=CARTESIAN_POINT('Ctrl Pts',(12.0519056543708,-51.796316921711,-0.9));
#81228=CARTESIAN_POINT('Ctrl Pts',(11.8269434198737,-51.6270129084587,-0.6));
#81229=CARTESIAN_POINT('Ctrl Pts',(11.8269434198737,-51.6270129084587,-0.9));
#81230=CARTESIAN_POINT('Ctrl Pts',(11.4860143885016,-51.6270129084587,-0.6));
#81231=CARTESIAN_POINT('Ctrl Pts',(11.4860143885016,-51.6270129084587,-0.9));
#81232=CARTESIAN_POINT('',(12.0519056543708,-51.796316921711,-0.6));
#81233=CARTESIAN_POINT('Ctrl Pts',(12.0519056543708,-51.796316921711,-0.6));
#81234=CARTESIAN_POINT('Ctrl Pts',(11.8269434198737,-51.6270129084587,-0.6));
#81235=CARTESIAN_POINT('Ctrl Pts',(11.4860143885016,-51.6270129084587,-0.6));
#81236=CARTESIAN_POINT('',(12.0519056543708,-51.796316921711,-0.9));
#81237=CARTESIAN_POINT('',(12.0519056543708,-51.796316921711,-0.6));
#81238=CARTESIAN_POINT('Ctrl Pts',(12.0519056543708,-51.796316921711,-0.9));
#81239=CARTESIAN_POINT('Ctrl Pts',(11.8269434198737,-51.6270129084587,-0.9));
#81240=CARTESIAN_POINT('Ctrl Pts',(11.4860143885016,-51.6270129084587,-0.9));
#81241=CARTESIAN_POINT('Ctrl Pts',(12.3951521143317,-52.3366985917091,-0.6));
#81242=CARTESIAN_POINT('Ctrl Pts',(12.3951521143317,-52.3366985917091,-0.9));
#81243=CARTESIAN_POINT('Ctrl Pts',(12.276877425611,-51.9656209349632,-0.6));
#81244=CARTESIAN_POINT('Ctrl Pts',(12.276877425611,-51.9656209349632,-0.9));
#81245=CARTESIAN_POINT('Ctrl Pts',(12.0519056543708,-51.796316921711,-0.6));
#81246=CARTESIAN_POINT('Ctrl Pts',(12.0519056543708,-51.796316921711,-0.9));
#81247=CARTESIAN_POINT('',(12.3951521143317,-52.3366985917091,-0.6));
#81248=CARTESIAN_POINT('Ctrl Pts',(12.3951521143317,-52.3366985917091,-0.6));
#81249=CARTESIAN_POINT('Ctrl Pts',(12.276877425611,-51.9656209349632,-0.6));
#81250=CARTESIAN_POINT('Ctrl Pts',(12.0519056543708,-51.796316921711,-0.6));
#81251=CARTESIAN_POINT('',(12.3951521143317,-52.3366985917091,-0.9));
#81252=CARTESIAN_POINT('',(12.3951521143317,-52.3366985917091,-0.6));
#81253=CARTESIAN_POINT('Ctrl Pts',(12.3951521143317,-52.3366985917091,-0.9));
#81254=CARTESIAN_POINT('Ctrl Pts',(12.276877425611,-51.9656209349632,-0.9));
#81255=CARTESIAN_POINT('Ctrl Pts',(12.0519056543708,-51.796316921711,-0.9));
#81256=CARTESIAN_POINT('Origin',(12.8381338343024,-52.2323332428932,-0.6));
#81257=CARTESIAN_POINT('',(12.8381338343024,-52.2323332428932,-0.6));
#81258=CARTESIAN_POINT('',(6.67095317451304,-53.685305073903,-0.6));
#81259=CARTESIAN_POINT('',(12.8381338343024,-52.2323332428932,-0.9));
#81260=CARTESIAN_POINT('',(12.8381338343024,-52.2323332428932,-0.6));
#81261=CARTESIAN_POINT('',(12.8381338343024,-52.2323332428932,-0.9));
#81262=CARTESIAN_POINT('Ctrl Pts',(12.3534097895026,-51.5017740130424,-0.6));
#81263=CARTESIAN_POINT('Ctrl Pts',(12.3534097895026,-51.5017740130424,-0.9));
#81264=CARTESIAN_POINT('Ctrl Pts',(12.7012911066413,-51.7615286707878,-0.6));
#81265=CARTESIAN_POINT('Ctrl Pts',(12.7012911066413,-51.7615286707878,-0.9));
#81266=CARTESIAN_POINT('Ctrl Pts',(12.8381338343024,-52.2323332428932,-0.6));
#81267=CARTESIAN_POINT('Ctrl Pts',(12.8381338343024,-52.2323332428932,-0.9));
#81268=CARTESIAN_POINT('',(12.3534097895026,-51.5017740130424,-0.6));
#81269=CARTESIAN_POINT('Ctrl Pts',(12.3534097895026,-51.5017740130424,-0.6));
#81270=CARTESIAN_POINT('Ctrl Pts',(12.7012911066413,-51.7615286707878,-0.6));
#81271=CARTESIAN_POINT('Ctrl Pts',(12.8381338343024,-52.2323332428932,-0.6));
#81272=CARTESIAN_POINT('',(12.3534097895026,-51.5017740130424,-0.9));
#81273=CARTESIAN_POINT('',(12.3534097895026,-51.5017740130424,-0.6));
#81274=CARTESIAN_POINT('Ctrl Pts',(12.3534097895026,-51.5017740130424,-0.9));
#81275=CARTESIAN_POINT('Ctrl Pts',(12.7012911066413,-51.7615286707878,-0.9));
#81276=CARTESIAN_POINT('Ctrl Pts',(12.8381338343024,-52.2323332428932,-0.9));
#81277=CARTESIAN_POINT('Ctrl Pts',(11.4952936396003,-51.2420193552971,-0.6));
#81278=CARTESIAN_POINT('Ctrl Pts',(11.4952936396003,-51.2420193552971,-0.9));
#81279=CARTESIAN_POINT('Ctrl Pts',(12.0055284723639,-51.2420193552971,-0.6));
#81280=CARTESIAN_POINT('Ctrl Pts',(12.0055284723639,-51.2420193552971,-0.9));
#81281=CARTESIAN_POINT('Ctrl Pts',(12.3534097895026,-51.5017740130424,-0.6));
#81282=CARTESIAN_POINT('Ctrl Pts',(12.3534097895026,-51.5017740130424,-0.9));
#81283=CARTESIAN_POINT('',(11.4952936396003,-51.2420193552971,-0.6));
#81284=CARTESIAN_POINT('Ctrl Pts',(11.4952936396003,-51.2420193552971,-0.6));
#81285=CARTESIAN_POINT('Ctrl Pts',(12.0055284723639,-51.2420193552971,-0.6));
#81286=CARTESIAN_POINT('Ctrl Pts',(12.3534097895026,-51.5017740130424,-0.6));
#81287=CARTESIAN_POINT('',(11.4952936396003,-51.2420193552971,-0.9));
#81288=CARTESIAN_POINT('',(11.4952936396003,-51.2420193552971,-0.6));
#81289=CARTESIAN_POINT('Ctrl Pts',(11.4952936396003,-51.2420193552971,-0.9));
#81290=CARTESIAN_POINT('Ctrl Pts',(12.0055284723639,-51.2420193552971,-0.9));
#81291=CARTESIAN_POINT('Ctrl Pts',(12.3534097895026,-51.5017740130424,-0.9));
#81292=CARTESIAN_POINT('Ctrl Pts',(10.6708040460944,-51.4472715258598,-0.6));
#81293=CARTESIAN_POINT('Ctrl Pts',(10.6708040460944,-51.4472715258598,-0.9));
#81294=CARTESIAN_POINT('Ctrl Pts',(11.045359633863,-51.2420193552971,-0.6));
#81295=CARTESIAN_POINT('Ctrl Pts',(11.045359633863,-51.2420193552971,-0.9));
#81296=CARTESIAN_POINT('Ctrl Pts',(11.4952936396003,-51.2420193552971,-0.6));
#81297=CARTESIAN_POINT('Ctrl Pts',(11.4952936396003,-51.2420193552971,-0.9));
#81298=CARTESIAN_POINT('',(10.6708040460944,-51.4472715258598,-0.6));
#81299=CARTESIAN_POINT('Ctrl Pts',(10.6708040460944,-51.4472715258598,-0.6));
#81300=CARTESIAN_POINT('Ctrl Pts',(11.045359633863,-51.2420193552971,-0.6));
#81301=CARTESIAN_POINT('Ctrl Pts',(11.4952936396003,-51.2420193552971,-0.6));
#81302=CARTESIAN_POINT('',(10.6708040460944,-51.4472715258598,-0.9));
#81303=CARTESIAN_POINT('',(10.6708040460944,-51.4472715258598,-0.6));
#81304=CARTESIAN_POINT('Ctrl Pts',(10.6708040460944,-51.4472715258598,-0.9));
#81305=CARTESIAN_POINT('Ctrl Pts',(11.045359633863,-51.2420193552971,-0.9));
#81306=CARTESIAN_POINT('Ctrl Pts',(11.4952936396003,-51.2420193552971,-0.9));
#81307=CARTESIAN_POINT('Ctrl Pts',(10.0933161005378,-52.0479540228844,-0.6));
#81308=CARTESIAN_POINT('Ctrl Pts',(10.0933161005378,-52.0479540228844,-0.9));
#81309=CARTESIAN_POINT('Ctrl Pts',(10.2962484583259,-51.652524292469,-0.6));
#81310=CARTESIAN_POINT('Ctrl Pts',(10.2962484583259,-51.652524292469,-0.9));
#81311=CARTESIAN_POINT('Ctrl Pts',(10.6708040460944,-51.4472715258598,-0.6));
#81312=CARTESIAN_POINT('Ctrl Pts',(10.6708040460944,-51.4472715258598,-0.9));
#81313=CARTESIAN_POINT('',(10.0933161005378,-52.0479540228844,-0.6));
#81314=CARTESIAN_POINT('Ctrl Pts',(10.0933161005378,-52.0479540228844,-0.6));
#81315=CARTESIAN_POINT('Ctrl Pts',(10.2962484583259,-51.652524292469,-0.6));
#81316=CARTESIAN_POINT('Ctrl Pts',(10.6708040460944,-51.4472715258598,-0.6));
#81317=CARTESIAN_POINT('',(10.0933161005378,-52.0479540228844,-0.9));
#81318=CARTESIAN_POINT('',(10.0933161005378,-52.0479540228844,-0.6));
#81319=CARTESIAN_POINT('Ctrl Pts',(10.0933161005378,-52.0479540228844,-0.9));
#81320=CARTESIAN_POINT('Ctrl Pts',(10.2962484583259,-51.652524292469,-0.9));
#81321=CARTESIAN_POINT('Ctrl Pts',(10.6708040460944,-51.4472715258598,-0.9));
#81322=CARTESIAN_POINT('Ctrl Pts',(9.89038374274969,-52.974488556385,-0.6));
#81323=CARTESIAN_POINT('Ctrl Pts',(9.89038374274969,-52.974488556385,-0.9));
#81324=CARTESIAN_POINT('Ctrl Pts',(9.89038374274969,-52.4433831572533,-0.6));
#81325=CARTESIAN_POINT('Ctrl Pts',(9.89038374274969,-52.4433831572533,-0.9));
#81326=CARTESIAN_POINT('Ctrl Pts',(10.0933161005378,-52.0479540228844,-0.6));
#81327=CARTESIAN_POINT('Ctrl Pts',(10.0933161005378,-52.0479540228844,-0.9));
#81328=CARTESIAN_POINT('',(9.89038374274969,-52.974488556385,-0.6));
#81329=CARTESIAN_POINT('Ctrl Pts',(9.89038374274969,-52.974488556385,-0.6));
#81330=CARTESIAN_POINT('Ctrl Pts',(9.89038374274969,-52.4433831572533,-0.6));
#81331=CARTESIAN_POINT('Ctrl Pts',(10.0933161005378,-52.0479540228844,-0.6));
#81332=CARTESIAN_POINT('',(9.89038374274969,-52.974488556385,-0.9));
#81333=CARTESIAN_POINT('',(9.89038374274969,-52.974488556385,-0.6));
#81334=CARTESIAN_POINT('Ctrl Pts',(9.89038374274969,-52.974488556385,-0.9));
#81335=CARTESIAN_POINT('Ctrl Pts',(9.89038374274969,-52.4433831572533,-0.9));
#81336=CARTESIAN_POINT('Ctrl Pts',(10.0933161005378,-52.0479540228844,-0.9));
#81337=CARTESIAN_POINT('Ctrl Pts',(10.0701227411628,-53.8859484791756,-0.6));
#81338=CARTESIAN_POINT('Ctrl Pts',(10.0701227411628,-53.8859484791756,-0.9));
#81339=CARTESIAN_POINT('Ctrl Pts',(9.89038374274969,-53.4615282416344,-0.6));
#81340=CARTESIAN_POINT('Ctrl Pts',(9.89038374274969,-53.4615282416344,-0.9));
#81341=CARTESIAN_POINT('Ctrl Pts',(9.89038374274969,-52.974488556385,-0.6));
#81342=CARTESIAN_POINT('Ctrl Pts',(9.89038374274969,-52.974488556385,-0.9));
#81343=CARTESIAN_POINT('',(10.0701227411628,-53.8859484791756,-0.6));
#81344=CARTESIAN_POINT('Ctrl Pts',(10.0701227411628,-53.8859484791756,-0.6));
#81345=CARTESIAN_POINT('Ctrl Pts',(9.89038374274969,-53.4615282416344,-0.6));
#81346=CARTESIAN_POINT('Ctrl Pts',(9.89038374274969,-52.974488556385,-0.6));
#81347=CARTESIAN_POINT('',(10.0701227411628,-53.8859484791756,-0.9));
#81348=CARTESIAN_POINT('',(10.0701227411628,-53.8859484791756,-0.6));
#81349=CARTESIAN_POINT('Ctrl Pts',(10.0701227411628,-53.8859484791756,-0.9));
#81350=CARTESIAN_POINT('Ctrl Pts',(9.89038374274969,-53.4615282416344,-0.9));
#81351=CARTESIAN_POINT('Ctrl Pts',(9.89038374274969,-52.974488556385,-0.9));
#81352=CARTESIAN_POINT('Ctrl Pts',(10.5942716822028,-54.5341746211052,-0.6));
#81353=CARTESIAN_POINT('Ctrl Pts',(10.5942716822028,-54.5341746211052,-0.9));
#81354=CARTESIAN_POINT('Ctrl Pts',(10.2498617395759,-54.3103687167168,-0.6));
#81355=CARTESIAN_POINT('Ctrl Pts',(10.2498617395759,-54.3103687167168,-0.9));
#81356=CARTESIAN_POINT('Ctrl Pts',(10.0701227411628,-53.8859484791756,-0.6));
#81357=CARTESIAN_POINT('Ctrl Pts',(10.0701227411628,-53.8859484791756,-0.9));
#81358=CARTESIAN_POINT('',(10.5942716822028,-54.5341746211052,-0.6));
#81359=CARTESIAN_POINT('Ctrl Pts',(10.5942716822028,-54.5341746211052,-0.6));
#81360=CARTESIAN_POINT('Ctrl Pts',(10.2498617395759,-54.3103687167168,-0.6));
#81361=CARTESIAN_POINT('Ctrl Pts',(10.0701227411628,-53.8859484791756,-0.6));
#81362=CARTESIAN_POINT('',(10.5942716822028,-54.5341746211052,-0.9));
#81363=CARTESIAN_POINT('',(10.5942716822028,-54.5341746211052,-0.6));
#81364=CARTESIAN_POINT('Ctrl Pts',(10.5942716822028,-54.5341746211052,-0.9));
#81365=CARTESIAN_POINT('Ctrl Pts',(10.2498617395759,-54.3103687167168,-0.9));
#81366=CARTESIAN_POINT('Ctrl Pts',(10.0701227411628,-53.8859484791756,-0.9));
#81367=CARTESIAN_POINT('Ctrl Pts',(11.4883318170905,-54.7579811215401,-0.6));
#81368=CARTESIAN_POINT('Ctrl Pts',(11.4883318170905,-54.7579811215401,-0.9));
#81369=CARTESIAN_POINT('Ctrl Pts',(10.9386720880866,-54.7579811215401,-0.6));
#81370=CARTESIAN_POINT('Ctrl Pts',(10.9386720880866,-54.7579811215401,-0.9));
#81371=CARTESIAN_POINT('Ctrl Pts',(10.5942716822028,-54.5341746211052,-0.6));
#81372=CARTESIAN_POINT('Ctrl Pts',(10.5942716822028,-54.5341746211052,-0.9));
#81373=CARTESIAN_POINT('',(11.4883318170905,-54.7579811215401,-0.6));
#81374=CARTESIAN_POINT('Ctrl Pts',(11.4883318170905,-54.7579811215401,-0.6));
#81375=CARTESIAN_POINT('Ctrl Pts',(10.9386720880866,-54.7579811215401,-0.6));
#81376=CARTESIAN_POINT('Ctrl Pts',(10.5942716822028,-54.5341746211052,-0.6));
#81377=CARTESIAN_POINT('',(11.4883318170905,-54.7579811215401,-0.9));
#81378=CARTESIAN_POINT('',(11.4883318170905,-54.7579811215401,-0.6));
#81379=CARTESIAN_POINT('Ctrl Pts',(11.4883318170905,-54.7579811215401,-0.9));
#81380=CARTESIAN_POINT('Ctrl Pts',(10.9386720880866,-54.7579811215401,-0.9));
#81381=CARTESIAN_POINT('Ctrl Pts',(10.5942716822028,-54.5341746211052,-0.9));
#81382=CARTESIAN_POINT('Ctrl Pts',(12.3870363458991,-54.4669167399406,-0.6));
#81383=CARTESIAN_POINT('Ctrl Pts',(12.3870363458991,-54.4669167399406,-0.9));
#81384=CARTESIAN_POINT('Ctrl Pts',(12.0194425806403,-54.7579811215401,-0.6));
#81385=CARTESIAN_POINT('Ctrl Pts',(12.0194425806403,-54.7579811215401,-0.9));
#81386=CARTESIAN_POINT('Ctrl Pts',(11.4883318170905,-54.7579811215401,-0.6));
#81387=CARTESIAN_POINT('Ctrl Pts',(11.4883318170905,-54.7579811215401,-0.9));
#81388=CARTESIAN_POINT('',(12.3870363458991,-54.4669167399406,-0.6));
#81389=CARTESIAN_POINT('Ctrl Pts',(12.3870363458991,-54.4669167399406,-0.6));
#81390=CARTESIAN_POINT('Ctrl Pts',(12.0194425806403,-54.7579811215401,-0.6));
#81391=CARTESIAN_POINT('Ctrl Pts',(11.4883318170905,-54.7579811215401,-0.6));
#81392=CARTESIAN_POINT('',(12.3870363458991,-54.4669167399406,-0.9));
#81393=CARTESIAN_POINT('',(12.3870363458991,-54.4669167399406,-0.6));
#81394=CARTESIAN_POINT('Ctrl Pts',(12.3870363458991,-54.4669167399406,-0.9));
#81395=CARTESIAN_POINT('Ctrl Pts',(12.0194425806403,-54.7579811215401,-0.9));
#81396=CARTESIAN_POINT('Ctrl Pts',(11.4883318170905,-54.7579811215401,-0.9));
#81397=CARTESIAN_POINT('Ctrl Pts',(12.8961076959968,-53.6215553879738,-0.6));
#81398=CARTESIAN_POINT('Ctrl Pts',(12.8961076959968,-53.6215553879738,-0.9));
#81399=CARTESIAN_POINT('Ctrl Pts',(12.7546396479011,-54.1758529543877,-0.6));
#81400=CARTESIAN_POINT('Ctrl Pts',(12.7546396479011,-54.1758529543877,-0.9));
#81401=CARTESIAN_POINT('Ctrl Pts',(12.3870363458991,-54.4669167399406,-0.6));
#81402=CARTESIAN_POINT('Ctrl Pts',(12.3870363458991,-54.4669167399406,-0.9));
#81403=CARTESIAN_POINT('',(12.8961076959968,-53.6215553879738,-0.6));
#81404=CARTESIAN_POINT('Ctrl Pts',(12.8961076959968,-53.6215553879738,-0.6));
#81405=CARTESIAN_POINT('Ctrl Pts',(12.7546396479011,-54.1758529543877,-0.6));
#81406=CARTESIAN_POINT('Ctrl Pts',(12.3870363458991,-54.4669167399406,-0.6));
#81407=CARTESIAN_POINT('',(12.8961076959968,-53.6215553879738,-0.9));
#81408=CARTESIAN_POINT('',(12.8961076959968,-53.6215553879738,-0.6));
#81409=CARTESIAN_POINT('Ctrl Pts',(12.8961076959968,-53.6215553879738,-0.9));
#81410=CARTESIAN_POINT('Ctrl Pts',(12.7546396479011,-54.1758529543877,-0.9));
#81411=CARTESIAN_POINT('Ctrl Pts',(12.3870363458991,-54.4669167399406,-0.9));
#81412=CARTESIAN_POINT('Origin',(12.4461832270026,-53.5079125761986,-0.6));
#81413=CARTESIAN_POINT('',(12.4461832270026,-53.5079125761986,-0.6));
#81414=CARTESIAN_POINT('',(6.53600250299025,-52.0151074458665,-0.6));
#81415=CARTESIAN_POINT('',(12.4461832270026,-53.5079125761986,-0.9));
#81416=CARTESIAN_POINT('',(12.4461832270026,-53.5079125761986,-0.6));
#81417=CARTESIAN_POINT('',(12.4461832270026,-53.5079125761986,-0.9));
#81418=CARTESIAN_POINT('Ctrl Pts',(12.0913400873542,-54.1549794077873,-0.6));
#81419=CARTESIAN_POINT('Ctrl Pts',(12.0913400873542,-54.1549794077873,-0.9));
#81420=CARTESIAN_POINT('Ctrl Pts',(12.3534097895026,-53.9369718432426,-0.6));
#81421=CARTESIAN_POINT('Ctrl Pts',(12.3534097895026,-53.9369718432426,-0.9));
#81422=CARTESIAN_POINT('Ctrl Pts',(12.4461832270026,-53.5079125761986,-0.6));
#81423=CARTESIAN_POINT('Ctrl Pts',(12.4461832270026,-53.5079125761986,-0.9));
#81424=CARTESIAN_POINT('',(12.0913400873542,-54.1549794077873,-0.6));
#81425=CARTESIAN_POINT('Ctrl Pts',(12.0913400873542,-54.1549794077873,-0.6));
#81426=CARTESIAN_POINT('Ctrl Pts',(12.3534097895026,-53.9369718432426,-0.6));
#81427=CARTESIAN_POINT('Ctrl Pts',(12.4461832270026,-53.5079125761986,-0.6));
#81428=CARTESIAN_POINT('',(12.0913400873542,-54.1549794077873,-0.9));
#81429=CARTESIAN_POINT('',(12.0913400873542,-54.1549794077873,-0.6));
#81430=CARTESIAN_POINT('Ctrl Pts',(12.0913400873542,-54.1549794077873,-0.9));
#81431=CARTESIAN_POINT('Ctrl Pts',(12.3534097895026,-53.9369718432426,-0.9));
#81432=CARTESIAN_POINT('Ctrl Pts',(12.4461832270026,-53.5079125761986,-0.9));
#81433=CARTESIAN_POINT('Ctrl Pts',(11.4512243494391,-54.3729875683784,-0.6));
#81434=CARTESIAN_POINT('Ctrl Pts',(11.4512243494391,-54.3729875683784,-0.9));
#81435=CARTESIAN_POINT('Ctrl Pts',(11.8292608484626,-54.3729875683784,-0.6));
#81436=CARTESIAN_POINT('Ctrl Pts',(11.8292608484626,-54.3729875683784,-0.9));
#81437=CARTESIAN_POINT('Ctrl Pts',(12.0913400873542,-54.1549794077873,-0.6));
#81438=CARTESIAN_POINT('Ctrl Pts',(12.0913400873542,-54.1549794077873,-0.9));
#81439=CARTESIAN_POINT('Ctrl Pts',(11.4512243494391,-54.3729875683784,-0.6));
#81440=CARTESIAN_POINT('Ctrl Pts',(11.8292608484626,-54.3729875683784,-0.6));
#81441=CARTESIAN_POINT('Ctrl Pts',(12.0913400873542,-54.1549794077873,-0.6));
#81442=CARTESIAN_POINT('Ctrl Pts',(11.4512243494391,-54.3729875683784,-0.9));
#81443=CARTESIAN_POINT('Ctrl Pts',(11.8292608484626,-54.3729875683784,-0.9));
#81444=CARTESIAN_POINT('Ctrl Pts',(12.0913400873542,-54.1549794077873,-0.9));
#81445=CARTESIAN_POINT('Origin',(11.3932457193732,-53.0000002384186,-0.9));
#81446=CARTESIAN_POINT('Origin',(4.11548521369696,-54.2987720370293,-0.6));
#81447=CARTESIAN_POINT('',(4.11548521369696,-54.2987720370293,-0.6));
#81448=CARTESIAN_POINT('',(5.78997518867254,-54.2987720370293,-0.6));
#81449=CARTESIAN_POINT('',(2.05774260684848,-54.2987720370293,-0.6));
#81450=CARTESIAN_POINT('',(4.11548521369696,-54.2987720370293,-0.9));
#81451=CARTESIAN_POINT('',(4.11548521369696,-54.2987720370293,-0.6));
#81452=CARTESIAN_POINT('',(5.78997518867254,-54.2987720370293,-0.9));
#81453=CARTESIAN_POINT('',(4.11548521369696,-54.2987720370293,-0.9));
#81454=CARTESIAN_POINT('',(5.78997518867254,-54.2987720370293,-0.6));
#81455=CARTESIAN_POINT('Origin',(4.11548521369696,-51.3000003695488,-0.6));
#81456=CARTESIAN_POINT('',(4.11548521369696,-51.3000003695488,-0.6));
#81457=CARTESIAN_POINT('',(4.11548521369696,-52.1500001847744,-0.6));
#81458=CARTESIAN_POINT('',(4.11548521369696,-51.3000003695488,-0.9));
#81459=CARTESIAN_POINT('',(4.11548521369696,-51.3000003695488,-0.6));
#81460=CARTESIAN_POINT('',(4.11548521369696,-51.3000003695488,-0.9));
#81461=CARTESIAN_POINT('Origin',(3.66555359214544,-51.3000003695488,-0.6));
#81462=CARTESIAN_POINT('',(3.66555359214544,-51.3000003695488,-0.6));
#81463=CARTESIAN_POINT('',(1.83277679607272,-51.3000003695488,-0.6));
#81464=CARTESIAN_POINT('',(3.66555359214544,-51.3000003695488,-0.9));
#81465=CARTESIAN_POINT('',(3.66555359214544,-51.3000003695488,-0.6));
#81466=CARTESIAN_POINT('',(3.66555359214544,-51.3000003695488,-0.9));
#81467=CARTESIAN_POINT('Origin',(3.66555359214544,-54.7000001072884,-0.6));
#81468=CARTESIAN_POINT('',(3.66555359214544,-54.7000001072884,-0.6));
#81469=CARTESIAN_POINT('',(3.66555359214544,-53.8500000536442,-0.6));
#81470=CARTESIAN_POINT('',(3.66555359214544,-54.7000001072884,-0.9));
#81471=CARTESIAN_POINT('',(3.66555359214544,-54.7000001072884,-0.6));
#81472=CARTESIAN_POINT('',(3.66555359214544,-54.7000001072884,-0.9));
#81473=CARTESIAN_POINT('Origin',(5.78997518867254,-54.7000001072884,-0.6));
#81474=CARTESIAN_POINT('',(5.78997518867254,-54.7000001072884,-0.6));
#81475=CARTESIAN_POINT('',(2.89498759433627,-54.7000001072884,-0.6));
#81476=CARTESIAN_POINT('',(5.78997518867254,-54.7000001072884,-0.9));
#81477=CARTESIAN_POINT('',(5.78997518867254,-54.7000001072884,-0.6));
#81478=CARTESIAN_POINT('',(5.78997518867254,-54.7000001072884,-0.9));
#81479=CARTESIAN_POINT('Origin',(5.78997518867254,-54.2987720370293,-0.6));
#81480=CARTESIAN_POINT('',(5.78997518867254,-53.6493860185146,-0.6));
#81481=CARTESIAN_POINT('',(5.78997518867254,-54.2987720370293,-0.9));
#81482=CARTESIAN_POINT('Origin',(4.72776439040899,-53.0000002384186,-0.9));
#81483=CARTESIAN_POINT('Origin',(-31.9741490855813,-51.7012278437614,-0.6));
#81484=CARTESIAN_POINT('',(-31.9741490855813,-51.7012278437614,-0.6));
#81485=CARTESIAN_POINT('',(-33.0989785864949,-51.7012278437614,-0.6));
#81486=CARTESIAN_POINT('',(-15.9870745427907,-51.7012278437614,-0.6));
#81487=CARTESIAN_POINT('',(-31.9741490855813,-51.7012278437614,-0.9));
#81488=CARTESIAN_POINT('',(-31.9741490855813,-51.7012278437614,-0.6));
#81489=CARTESIAN_POINT('',(-33.0989785864949,-51.7012278437614,-0.9));
#81490=CARTESIAN_POINT('',(-31.9741490855813,-51.7012278437614,-0.9));
#81491=CARTESIAN_POINT('',(-33.0989785864949,-51.7012278437614,-0.6));
#81492=CARTESIAN_POINT('Origin',(-31.9741490855813,-51.3000003695488,-0.6));
#81493=CARTESIAN_POINT('',(-31.9741490855813,-51.3000003695488,-0.6));
#81494=CARTESIAN_POINT('',(-31.9741490855813,-52.1500001847744,-0.6));
#81495=CARTESIAN_POINT('',(-31.9741490855813,-51.3000003695488,-0.9));
#81496=CARTESIAN_POINT('',(-31.9741490855813,-51.3000003695488,-0.6));
#81497=CARTESIAN_POINT('',(-31.9741490855813,-51.3000003695488,-0.9));
#81498=CARTESIAN_POINT('Origin',(-34.6691012382507,-51.3000003695488,-0.6));
#81499=CARTESIAN_POINT('',(-34.6691012382507,-51.3000003695488,-0.6));
#81500=CARTESIAN_POINT('',(-17.3345506191254,-51.3000003695488,-0.6));
#81501=CARTESIAN_POINT('',(-34.6691012382507,-51.3000003695488,-0.9));
#81502=CARTESIAN_POINT('',(-34.6691012382507,-51.3000003695488,-0.6));
#81503=CARTESIAN_POINT('',(-34.6691012382507,-51.3000003695488,-0.9));
#81504=CARTESIAN_POINT('Origin',(-34.6691012382507,-51.7012278437614,-0.6));
#81505=CARTESIAN_POINT('',(-34.6691012382507,-51.7012278437614,-0.6));
#81506=CARTESIAN_POINT('',(-34.6691012382507,-52.3506139218807,-0.6));
#81507=CARTESIAN_POINT('',(-34.6691012382507,-51.7012278437614,-0.9));
#81508=CARTESIAN_POINT('',(-34.6691012382507,-51.7012278437614,-0.6));
#81509=CARTESIAN_POINT('',(-34.6691012382507,-51.7012278437614,-0.9));
#81510=CARTESIAN_POINT('Origin',(-33.5489102080464,-51.7012278437614,-0.6));
#81511=CARTESIAN_POINT('',(-33.5489102080464,-51.7012278437614,-0.6));
#81512=CARTESIAN_POINT('',(-16.7744551040232,-51.7012278437614,-0.6));
#81513=CARTESIAN_POINT('',(-33.5489102080464,-51.7012278437614,-0.9));
#81514=CARTESIAN_POINT('',(-33.5489102080464,-51.7012278437614,-0.6));
#81515=CARTESIAN_POINT('',(-33.5489102080464,-51.7012278437614,-0.9));
#81516=CARTESIAN_POINT('Origin',(-33.5489102080464,-54.7000001072884,-0.6));
#81517=CARTESIAN_POINT('',(-33.5489102080464,-54.7000001072884,-0.6));
#81518=CARTESIAN_POINT('',(-33.5489102080464,-53.8500000536442,-0.6));
#81519=CARTESIAN_POINT('',(-33.5489102080464,-54.7000001072884,-0.9));
#81520=CARTESIAN_POINT('',(-33.5489102080464,-54.7000001072884,-0.6));
#81521=CARTESIAN_POINT('',(-33.5489102080464,-54.7000001072884,-0.9));
#81522=CARTESIAN_POINT('Origin',(-33.0989785864949,-54.7000001072884,-0.6));
#81523=CARTESIAN_POINT('',(-33.0989785864949,-54.7000001072884,-0.6));
#81524=CARTESIAN_POINT('',(-16.5494892932475,-54.7000001072884,-0.6));
#81525=CARTESIAN_POINT('',(-33.0989785864949,-54.7000001072884,-0.9));
#81526=CARTESIAN_POINT('',(-33.0989785864949,-54.7000001072884,-0.6));
#81527=CARTESIAN_POINT('',(-33.0989785864949,-54.7000001072884,-0.9));
#81528=CARTESIAN_POINT('Origin',(-33.0989785864949,-51.7012278437614,-0.6));
#81529=CARTESIAN_POINT('',(-33.0989785864949,-52.3506139218807,-0.6));
#81530=CARTESIAN_POINT('',(-33.0989785864949,-51.7012278437614,-0.9));
#81531=CARTESIAN_POINT('Origin',(-33.321625161916,-53.0000002384186,-0.9));
#81532=CARTESIAN_POINT('Ctrl Pts',(-3.18315122276545,-54.3521146178246,
-0.6));
#81533=CARTESIAN_POINT('Ctrl Pts',(-3.18315122276545,-54.3521146178246,
-0.9));
#81534=CARTESIAN_POINT('Ctrl Pts',(-2.68683526664972,-54.3521146178246,
-0.6));
#81535=CARTESIAN_POINT('Ctrl Pts',(-2.68683526664972,-54.3521146178246,
-0.9));
#81536=CARTESIAN_POINT('Ctrl Pts',(-2.47578475624323,-54.1271488070488,
-0.6));
#81537=CARTESIAN_POINT('Ctrl Pts',(-2.47578475624323,-54.1271488070488,
-0.9));
#81538=CARTESIAN_POINT('',(-3.18315122276545,-54.3521146178246,-0.6));
#81539=CARTESIAN_POINT('',(-2.47578475624323,-54.1271488070488,-0.6));
#81540=CARTESIAN_POINT('Ctrl Pts',(-3.18315122276545,-54.3521146178246,
-0.6));
#81541=CARTESIAN_POINT('Ctrl Pts',(-2.68683526664972,-54.3521146178246,
-0.6));
#81542=CARTESIAN_POINT('Ctrl Pts',(-2.47578475624323,-54.1271488070488,
-0.6));
#81543=CARTESIAN_POINT('',(-3.18315122276545,-54.3521146178246,-0.9));
#81544=CARTESIAN_POINT('',(-3.18315122276545,-54.3521146178246,-0.6));
#81545=CARTESIAN_POINT('',(-2.47578475624323,-54.1271488070488,-0.9));
#81546=CARTESIAN_POINT('Ctrl Pts',(-3.18315122276545,-54.3521146178246,
-0.9));
#81547=CARTESIAN_POINT('Ctrl Pts',(-2.68683526664972,-54.3521146178246,
-0.9));
#81548=CARTESIAN_POINT('Ctrl Pts',(-2.47578475624323,-54.1271488070488,
-0.9));
#81549=CARTESIAN_POINT('',(-2.47578475624323,-54.1271488070488,-0.6));
#81550=CARTESIAN_POINT('Ctrl Pts',(-3.67367122322321,-54.2384724020958,
-0.6));
#81551=CARTESIAN_POINT('Ctrl Pts',(-3.67367122322321,-54.2384724020958,
-0.9));
#81552=CARTESIAN_POINT('Ctrl Pts',(-3.47305629402399,-54.3521146178246,
-0.6));
#81553=CARTESIAN_POINT('Ctrl Pts',(-3.47305629402399,-54.3521146178246,
-0.9));
#81554=CARTESIAN_POINT('Ctrl Pts',(-3.18315122276545,-54.3521146178246,
-0.6));
#81555=CARTESIAN_POINT('Ctrl Pts',(-3.18315122276545,-54.3521146178246,
-0.9));
#81556=CARTESIAN_POINT('',(-3.67367122322321,-54.2384724020958,-0.6));
#81557=CARTESIAN_POINT('Ctrl Pts',(-3.67367122322321,-54.2384724020958,
-0.6));
#81558=CARTESIAN_POINT('Ctrl Pts',(-3.47305629402399,-54.3521146178246,
-0.6));
#81559=CARTESIAN_POINT('Ctrl Pts',(-3.18315122276545,-54.3521146178246,
-0.6));
#81560=CARTESIAN_POINT('',(-3.67367122322321,-54.2384724020958,-0.9));
#81561=CARTESIAN_POINT('',(-3.67367122322321,-54.2384724020958,-0.6));
#81562=CARTESIAN_POINT('Ctrl Pts',(-3.67367122322321,-54.2384724020958,
-0.9));
#81563=CARTESIAN_POINT('Ctrl Pts',(-3.47305629402399,-54.3521146178246,
-0.9));
#81564=CARTESIAN_POINT('Ctrl Pts',(-3.18315122276545,-54.3521146178246,
-0.9));
#81565=CARTESIAN_POINT('Ctrl Pts',(-3.95661685615778,-53.914938390255,-0.6));
#81566=CARTESIAN_POINT('Ctrl Pts',(-3.95661685615778,-53.914938390255,-0.9));
#81567=CARTESIAN_POINT('Ctrl Pts',(-3.87428376823664,-54.1248295903206,
-0.6));
#81568=CARTESIAN_POINT('Ctrl Pts',(-3.87428376823664,-54.1248295903206,
-0.9));
#81569=CARTESIAN_POINT('Ctrl Pts',(-3.67367122322321,-54.2384724020958,
-0.6));
#81570=CARTESIAN_POINT('Ctrl Pts',(-3.67367122322321,-54.2384724020958,
-0.9));
#81571=CARTESIAN_POINT('',(-3.95661685615778,-53.914938390255,-0.6));
#81572=CARTESIAN_POINT('Ctrl Pts',(-3.95661685615778,-53.914938390255,-0.6));
#81573=CARTESIAN_POINT('Ctrl Pts',(-3.87428376823664,-54.1248295903206,
-0.6));
#81574=CARTESIAN_POINT('Ctrl Pts',(-3.67367122322321,-54.2384724020958,
-0.6));
#81575=CARTESIAN_POINT('',(-3.95661685615778,-53.914938390255,-0.9));
#81576=CARTESIAN_POINT('',(-3.95661685615778,-53.914938390255,-0.6));
#81577=CARTESIAN_POINT('Ctrl Pts',(-3.95661685615778,-53.914938390255,-0.9));
#81578=CARTESIAN_POINT('Ctrl Pts',(-3.87428376823664,-54.1248295903206,
-0.9));
#81579=CARTESIAN_POINT('Ctrl Pts',(-3.67367122322321,-54.2384724020958,
-0.9));
#81580=CARTESIAN_POINT('Ctrl Pts',(-4.03894994407892,-53.2620738148689,
-0.6));
#81581=CARTESIAN_POINT('Ctrl Pts',(-4.03894994407892,-53.2620738148689,
-0.9));
#81582=CARTESIAN_POINT('Ctrl Pts',(-4.03894994407892,-53.7050477862358,
-0.6));
#81583=CARTESIAN_POINT('Ctrl Pts',(-4.03894994407892,-53.7050477862358,
-0.9));
#81584=CARTESIAN_POINT('Ctrl Pts',(-3.95661685615778,-53.914938390255,-0.6));
#81585=CARTESIAN_POINT('Ctrl Pts',(-3.95661685615778,-53.914938390255,-0.9));
#81586=CARTESIAN_POINT('',(-4.03894994407892,-53.2620738148689,-0.6));
#81587=CARTESIAN_POINT('Ctrl Pts',(-4.03894994407892,-53.2620738148689,
-0.6));
#81588=CARTESIAN_POINT('Ctrl Pts',(-4.03894994407892,-53.7050477862358,
-0.6));
#81589=CARTESIAN_POINT('Ctrl Pts',(-3.95661685615778,-53.914938390255,-0.6));
#81590=CARTESIAN_POINT('',(-4.03894994407892,-53.2620738148689,-0.9));
#81591=CARTESIAN_POINT('',(-4.03894994407892,-53.2620738148689,-0.6));
#81592=CARTESIAN_POINT('Ctrl Pts',(-4.03894994407892,-53.2620738148689,
-0.9));
#81593=CARTESIAN_POINT('Ctrl Pts',(-4.03894994407892,-53.7050477862358,
-0.9));
#81594=CARTESIAN_POINT('Ctrl Pts',(-3.95661685615778,-53.914938390255,-0.9));
#81595=CARTESIAN_POINT('Origin',(-4.03894994407892,-51.3000003695488,-0.6));
#81596=CARTESIAN_POINT('',(-4.03894994407892,-51.3000003695488,-0.6));
#81597=CARTESIAN_POINT('',(-4.03894994407892,-52.1500001847744,-0.6));
#81598=CARTESIAN_POINT('',(-4.03894994407892,-51.3000003695488,-0.9));
#81599=CARTESIAN_POINT('',(-4.03894994407892,-51.3000003695488,-0.6));
#81600=CARTESIAN_POINT('',(-4.03894994407892,-51.3000003695488,-0.9));
#81601=CARTESIAN_POINT('Origin',(-4.48888156563044,-51.3000003695488,-0.6));
#81602=CARTESIAN_POINT('',(-4.48888156563044,-51.3000003695488,-0.6));
#81603=CARTESIAN_POINT('',(-2.24444078281522,-51.3000003695488,-0.6));
#81604=CARTESIAN_POINT('',(-4.48888156563044,-51.3000003695488,-0.9));
#81605=CARTESIAN_POINT('',(-4.48888156563044,-51.3000003695488,-0.6));
#81606=CARTESIAN_POINT('',(-4.48888156563044,-51.3000003695488,-0.9));
#81607=CARTESIAN_POINT('Origin',(-4.48888156563044,-53.2643930315971,-0.6));
#81608=CARTESIAN_POINT('',(-4.48888156563044,-53.2643930315971,-0.6));
#81609=CARTESIAN_POINT('',(-4.48888156563044,-53.1321965157986,-0.6));
#81610=CARTESIAN_POINT('',(-4.48888156563044,-53.2643930315971,-0.9));
#81611=CARTESIAN_POINT('',(-4.48888156563044,-53.2643930315971,-0.6));
#81612=CARTESIAN_POINT('',(-4.48888156563044,-53.2643930315971,-0.9));
#81613=CARTESIAN_POINT('Ctrl Pts',(-4.35900542885065,-54.1167120337486,
-0.6));
#81614=CARTESIAN_POINT('Ctrl Pts',(-4.35900542885065,-54.1167120337486,
-0.9));
#81615=CARTESIAN_POINT('Ctrl Pts',(-4.48888156563044,-53.8047747015953,
-0.6));
#81616=CARTESIAN_POINT('Ctrl Pts',(-4.48888156563044,-53.8047747015953,
-0.9));
#81617=CARTESIAN_POINT('Ctrl Pts',(-4.48888156563044,-53.2643930315971,
-0.6));
#81618=CARTESIAN_POINT('Ctrl Pts',(-4.48888156563044,-53.2643930315971,
-0.9));
#81619=CARTESIAN_POINT('',(-4.35900542885065,-54.1167120337486,-0.6));
#81620=CARTESIAN_POINT('Ctrl Pts',(-4.35900542885065,-54.1167120337486,
-0.6));
#81621=CARTESIAN_POINT('Ctrl Pts',(-4.48888156563044,-53.8047747015953,
-0.6));
#81622=CARTESIAN_POINT('Ctrl Pts',(-4.48888156563044,-53.2643930315971,
-0.6));
#81623=CARTESIAN_POINT('',(-4.35900542885065,-54.1167120337486,-0.9));
#81624=CARTESIAN_POINT('',(-4.35900542885065,-54.1167120337486,-0.6));
#81625=CARTESIAN_POINT('Ctrl Pts',(-4.35900542885065,-54.1167120337486,
-0.9));
#81626=CARTESIAN_POINT('Ctrl Pts',(-4.48888156563044,-53.8047747015953,
-0.9));
#81627=CARTESIAN_POINT('Ctrl Pts',(-4.48888156563044,-53.2643930315971,
-0.9));
#81628=CARTESIAN_POINT('Ctrl Pts',(-3.92530772835016,-54.5933155417442,
-0.6));
#81629=CARTESIAN_POINT('Ctrl Pts',(-3.92530772835016,-54.5933155417442,
-0.9));
#81630=CARTESIAN_POINT('Ctrl Pts',(-4.22912690788507,-54.4286493659019,
-0.6));
#81631=CARTESIAN_POINT('Ctrl Pts',(-4.22912690788507,-54.4286493659019,
-0.9));
#81632=CARTESIAN_POINT('Ctrl Pts',(-4.35900542885065,-54.1167120337486,
-0.6));
#81633=CARTESIAN_POINT('Ctrl Pts',(-4.35900542885065,-54.1167120337486,
-0.9));
#81634=CARTESIAN_POINT('',(-3.92530772835016,-54.5933155417442,-0.6));
#81635=CARTESIAN_POINT('Ctrl Pts',(-3.92530772835016,-54.5933155417442,
-0.6));
#81636=CARTESIAN_POINT('Ctrl Pts',(-4.22912690788507,-54.4286493659019,
-0.6));
#81637=CARTESIAN_POINT('Ctrl Pts',(-4.35900542885065,-54.1167120337486,
-0.6));
#81638=CARTESIAN_POINT('',(-3.92530772835016,-54.5933155417442,-0.9));
#81639=CARTESIAN_POINT('',(-3.92530772835016,-54.5933155417442,-0.6));
#81640=CARTESIAN_POINT('Ctrl Pts',(-3.92530772835016,-54.5933155417442,
-0.9));
#81641=CARTESIAN_POINT('Ctrl Pts',(-4.22912690788507,-54.4286493659019,
-0.9));
#81642=CARTESIAN_POINT('Ctrl Pts',(-4.35900542885065,-54.1167120337486,
-0.9));
#81643=CARTESIAN_POINT('Ctrl Pts',(-3.14372394233942,-54.7579811215401,
-0.6));
#81644=CARTESIAN_POINT('Ctrl Pts',(-3.14372394233942,-54.7579811215401,
-0.9));
#81645=CARTESIAN_POINT('Ctrl Pts',(-3.62148616462946,-54.7579811215401,
-0.6));
#81646=CARTESIAN_POINT('Ctrl Pts',(-3.62148616462946,-54.7579811215401,
-0.9));
#81647=CARTESIAN_POINT('Ctrl Pts',(-3.92530772835016,-54.5933155417442,
-0.6));
#81648=CARTESIAN_POINT('Ctrl Pts',(-3.92530772835016,-54.5933155417442,
-0.9));
#81649=CARTESIAN_POINT('',(-3.14372394233942,-54.7579811215401,-0.6));
#81650=CARTESIAN_POINT('Ctrl Pts',(-3.14372394233942,-54.7579811215401,
-0.6));
#81651=CARTESIAN_POINT('Ctrl Pts',(-3.62148616462946,-54.7579811215401,
-0.6));
#81652=CARTESIAN_POINT('Ctrl Pts',(-3.92530772835016,-54.5933155417442,
-0.6));
#81653=CARTESIAN_POINT('',(-3.14372394233942,-54.7579811215401,-0.9));
#81654=CARTESIAN_POINT('',(-3.14372394233942,-54.7579811215401,-0.6));
#81655=CARTESIAN_POINT('Ctrl Pts',(-3.14372394233942,-54.7579811215401,
-0.9));
#81656=CARTESIAN_POINT('Ctrl Pts',(-3.62148616462946,-54.7579811215401,
-0.9));
#81657=CARTESIAN_POINT('Ctrl Pts',(-3.92530772835016,-54.5933155417442,
-0.9));
#81658=CARTESIAN_POINT('Ctrl Pts',(-2.34938714653254,-54.5689634680748,
-0.6));
#81659=CARTESIAN_POINT('Ctrl Pts',(-2.34938714653254,-54.5689634680748,
-0.9));
#81660=CARTESIAN_POINT('Ctrl Pts',(-2.65204761177301,-54.7579811215401,
-0.6));
#81661=CARTESIAN_POINT('Ctrl Pts',(-2.65204761177301,-54.7579811215401,
-0.9));
#81662=CARTESIAN_POINT('Ctrl Pts',(-3.14372394233942,-54.7579811215401,
-0.6));
#81663=CARTESIAN_POINT('Ctrl Pts',(-3.14372394233942,-54.7579811215401,
-0.9));
#81664=CARTESIAN_POINT('',(-2.34938714653254,-54.5689634680748,-0.6));
#81665=CARTESIAN_POINT('Ctrl Pts',(-2.34938714653254,-54.5689634680748,
-0.6));
#81666=CARTESIAN_POINT('Ctrl Pts',(-2.65204761177301,-54.7579811215401,
-0.6));
#81667=CARTESIAN_POINT('Ctrl Pts',(-3.14372394233942,-54.7579811215401,
-0.6));
#81668=CARTESIAN_POINT('',(-2.34938714653254,-54.5689634680748,-0.9));
#81669=CARTESIAN_POINT('',(-2.34938714653254,-54.5689634680748,-0.6));
#81670=CARTESIAN_POINT('Ctrl Pts',(-2.34938714653254,-54.5689634680748,
-0.9));
#81671=CARTESIAN_POINT('Ctrl Pts',(-2.65204761177301,-54.7579811215401,
-0.9));
#81672=CARTESIAN_POINT('Ctrl Pts',(-3.14372394233942,-54.7579811215401,
-0.9));
#81673=CARTESIAN_POINT('Ctrl Pts',(-1.93076465278864,-54.0784446597099,
-0.6));
#81674=CARTESIAN_POINT('Ctrl Pts',(-1.93076465278864,-54.0784446597099,
-0.9));
#81675=CARTESIAN_POINT('Ctrl Pts',(-2.04672668129206,-54.3799452185631,
-0.6));
#81676=CARTESIAN_POINT('Ctrl Pts',(-2.04672668129206,-54.3799452185631,
-0.9));
#81677=CARTESIAN_POINT('Ctrl Pts',(-2.34938714653254,-54.5689634680748,
-0.6));
#81678=CARTESIAN_POINT('Ctrl Pts',(-2.34938714653254,-54.5689634680748,
-0.9));
#81679=CARTESIAN_POINT('',(-1.93076465278864,-54.0784446597099,-0.6));
#81680=CARTESIAN_POINT('Ctrl Pts',(-1.93076465278864,-54.0784446597099,
-0.6));
#81681=CARTESIAN_POINT('Ctrl Pts',(-2.04672668129206,-54.3799452185631,
-0.6));
#81682=CARTESIAN_POINT('Ctrl Pts',(-2.34938714653254,-54.5689634680748,
-0.6));
#81683=CARTESIAN_POINT('',(-1.93076465278864,-54.0784446597099,-0.9));
#81684=CARTESIAN_POINT('',(-1.93076465278864,-54.0784446597099,-0.6));
#81685=CARTESIAN_POINT('Ctrl Pts',(-1.93076465278864,-54.0784446597099,
-0.9));
#81686=CARTESIAN_POINT('Ctrl Pts',(-2.04672668129206,-54.3799452185631,
-0.9));
#81687=CARTESIAN_POINT('Ctrl Pts',(-2.34938714653254,-54.5689634680748,
-0.9));
#81688=CARTESIAN_POINT('Ctrl Pts',(-1.81480262428522,-53.2643930315971,
-0.6));
#81689=CARTESIAN_POINT('Ctrl Pts',(-1.81480262428522,-53.2643930315971,
-0.9));
#81690=CARTESIAN_POINT('Ctrl Pts',(-1.81480262428522,-53.7769441008568,
-0.6));
#81691=CARTESIAN_POINT('Ctrl Pts',(-1.81480262428522,-53.7769441008568,
-0.9));
#81692=CARTESIAN_POINT('Ctrl Pts',(-1.93076465278864,-54.0784446597099,
-0.6));
#81693=CARTESIAN_POINT('Ctrl Pts',(-1.93076465278864,-54.0784446597099,
-0.9));
#81694=CARTESIAN_POINT('',(-1.81480262428522,-53.2643930315971,-0.6));
#81695=CARTESIAN_POINT('Ctrl Pts',(-1.81480262428522,-53.2643930315971,
-0.6));
#81696=CARTESIAN_POINT('Ctrl Pts',(-1.81480262428522,-53.7769441008568,
-0.6));
#81697=CARTESIAN_POINT('Ctrl Pts',(-1.93076465278864,-54.0784446597099,
-0.6));
#81698=CARTESIAN_POINT('',(-1.81480262428522,-53.2643930315971,-0.9));
#81699=CARTESIAN_POINT('',(-1.81480262428522,-53.2643930315971,-0.6));
#81700=CARTESIAN_POINT('Ctrl Pts',(-1.81480262428522,-53.2643930315971,
-0.9));
#81701=CARTESIAN_POINT('Ctrl Pts',(-1.81480262428522,-53.7769441008568,
-0.9));
#81702=CARTESIAN_POINT('Ctrl Pts',(-1.93076465278864,-54.0784446597099,
-0.9));
#81703=CARTESIAN_POINT('Origin',(-1.81480262428522,-51.3000003695488,-0.6));
#81704=CARTESIAN_POINT('',(-1.81480262428522,-51.3000003695488,-0.6));
#81705=CARTESIAN_POINT('',(-1.81480262428522,-52.1500001847744,-0.6));
#81706=CARTESIAN_POINT('',(-1.81480262428522,-51.3000003695488,-0.9));
#81707=CARTESIAN_POINT('',(-1.81480262428522,-51.3000003695488,-0.6));
#81708=CARTESIAN_POINT('',(-1.81480262428522,-51.3000003695488,-0.9));
#81709=CARTESIAN_POINT('Origin',(-2.26473424583673,-51.3000003695488,-0.6));
#81710=CARTESIAN_POINT('',(-2.26473424583673,-51.3000003695488,-0.6));
#81711=CARTESIAN_POINT('',(-1.13236712291837,-51.3000003695488,-0.6));
#81712=CARTESIAN_POINT('',(-2.26473424583673,-51.3000003695488,-0.9));
#81713=CARTESIAN_POINT('',(-2.26473424583673,-51.3000003695488,-0.6));
#81714=CARTESIAN_POINT('',(-2.26473424583673,-51.3000003695488,-0.9));
#81715=CARTESIAN_POINT('Origin',(-2.26473424583673,-53.2620738148689,-0.6));
#81716=CARTESIAN_POINT('',(-2.26473424583673,-53.2620738148689,-0.6));
#81717=CARTESIAN_POINT('',(-2.26473424583673,-53.1310369074345,-0.6));
#81718=CARTESIAN_POINT('',(-2.26473424583673,-53.2620738148689,-0.9));
#81719=CARTESIAN_POINT('',(-2.26473424583673,-53.2620738148689,-0.6));
#81720=CARTESIAN_POINT('',(-2.26473424583673,-53.2620738148689,-0.9));
#81721=CARTESIAN_POINT('Ctrl Pts',(-2.47578475624323,-54.1271488070488,
-0.6));
#81722=CARTESIAN_POINT('Ctrl Pts',(-2.47578475624323,-54.1271488070488,
-0.9));
#81723=CARTESIAN_POINT('Ctrl Pts',(-2.26473424583673,-53.902182996273,-0.6));
#81724=CARTESIAN_POINT('Ctrl Pts',(-2.26473424583673,-53.902182996273,-0.9));
#81725=CARTESIAN_POINT('Ctrl Pts',(-2.26473424583673,-53.2620738148689,
-0.6));
#81726=CARTESIAN_POINT('Ctrl Pts',(-2.26473424583673,-53.2620738148689,
-0.9));
#81727=CARTESIAN_POINT('Ctrl Pts',(-2.47578475624323,-54.1271488070488,
-0.6));
#81728=CARTESIAN_POINT('Ctrl Pts',(-2.26473424583673,-53.902182996273,-0.6));
#81729=CARTESIAN_POINT('Ctrl Pts',(-2.26473424583673,-53.2620738148689,
-0.6));
#81730=CARTESIAN_POINT('Ctrl Pts',(-2.47578475624323,-54.1271488070488,
-0.9));
#81731=CARTESIAN_POINT('Ctrl Pts',(-2.26473424583673,-53.902182996273,-0.9));
#81732=CARTESIAN_POINT('Ctrl Pts',(-2.26473424583673,-53.2620738148689,
-0.9));
#81733=CARTESIAN_POINT('Origin',(-3.15184209495783,-53.0289907455444,-0.9));
#81734=CARTESIAN_POINT('Origin',(-10.6418142095208,-53.190177500248,-0.6));
#81735=CARTESIAN_POINT('',(-10.6418142095208,-53.190177500248,-0.6));
#81736=CARTESIAN_POINT('',(-11.1636433377862,-53.190177500248,-0.6));
#81737=CARTESIAN_POINT('',(-5.32090710476041,-53.190177500248,-0.6));
#81738=CARTESIAN_POINT('',(-10.6418142095208,-53.190177500248,-0.9));
#81739=CARTESIAN_POINT('',(-10.6418142095208,-53.190177500248,-0.6));
#81740=CARTESIAN_POINT('',(-11.1636433377862,-53.190177500248,-0.9));
#81741=CARTESIAN_POINT('',(-10.6418142095208,-53.190177500248,-0.9));
#81742=CARTESIAN_POINT('',(-11.1636433377862,-53.190177500248,-0.6));
#81743=CARTESIAN_POINT('Ctrl Pts',(-10.3913364186883,-53.2064120173454,
-0.6));
#81744=CARTESIAN_POINT('Ctrl Pts',(-10.3913364186883,-53.2064120173454,
-0.9));
#81745=CARTESIAN_POINT('Ctrl Pts',(-10.4678711667657,-53.190177500248,-0.6));
#81746=CARTESIAN_POINT('Ctrl Pts',(-10.4678711667657,-53.190177500248,-0.9));
#81747=CARTESIAN_POINT('Ctrl Pts',(-10.6418142095208,-53.190177500248,-0.6));
#81748=CARTESIAN_POINT('Ctrl Pts',(-10.6418142095208,-53.190177500248,-0.9));
#81749=CARTESIAN_POINT('',(-10.3913364186883,-53.2064120173454,-0.6));
#81750=CARTESIAN_POINT('Ctrl Pts',(-10.3913364186883,-53.2064120173454,
-0.6));
#81751=CARTESIAN_POINT('Ctrl Pts',(-10.4678711667657,-53.190177500248,-0.6));
#81752=CARTESIAN_POINT('Ctrl Pts',(-10.6418142095208,-53.190177500248,-0.6));
#81753=CARTESIAN_POINT('',(-10.3913364186883,-53.2064120173454,-0.9));
#81754=CARTESIAN_POINT('',(-10.3913364186883,-53.2064120173454,-0.6));
#81755=CARTESIAN_POINT('Ctrl Pts',(-10.3913364186883,-53.2064120173454,
-0.9));
#81756=CARTESIAN_POINT('Ctrl Pts',(-10.4678711667657,-53.190177500248,-0.9));
#81757=CARTESIAN_POINT('Ctrl Pts',(-10.6418142095208,-53.190177500248,-0.9));
#81758=CARTESIAN_POINT('Ctrl Pts',(-10.1860842481256,-53.2968620657921,
-0.6));
#81759=CARTESIAN_POINT('Ctrl Pts',(-10.1860842481256,-53.2968620657921,
-0.9));
#81760=CARTESIAN_POINT('Ctrl Pts',(-10.2869710698724,-53.2319239974022,
-0.6));
#81761=CARTESIAN_POINT('Ctrl Pts',(-10.2869710698724,-53.2319239974022,
-0.9));
#81762=CARTESIAN_POINT('Ctrl Pts',(-10.3913364186883,-53.2064120173454,
-0.6));
#81763=CARTESIAN_POINT('Ctrl Pts',(-10.3913364186883,-53.2064120173454,
-0.9));
#81764=CARTESIAN_POINT('',(-10.1860842481256,-53.2968620657921,-0.6));
#81765=CARTESIAN_POINT('Ctrl Pts',(-10.1860842481256,-53.2968620657921,
-0.6));
#81766=CARTESIAN_POINT('Ctrl Pts',(-10.2869710698724,-53.2319239974022,
-0.6));
#81767=CARTESIAN_POINT('Ctrl Pts',(-10.3913364186883,-53.2064120173454,
-0.6));
#81768=CARTESIAN_POINT('',(-10.1860842481256,-53.2968620657921,-0.9));
#81769=CARTESIAN_POINT('',(-10.1860842481256,-53.2968620657921,-0.6));
#81770=CARTESIAN_POINT('Ctrl Pts',(-10.1860842481256,-53.2968620657921,
-0.9));
#81771=CARTESIAN_POINT('Ctrl Pts',(-10.2869710698724,-53.2319239974022,
-0.9));
#81772=CARTESIAN_POINT('Ctrl Pts',(-10.3913364186883,-53.2064120173454,
-0.9));
#81773=CARTESIAN_POINT('Ctrl Pts',(-9.9576411023736,-53.5241476893425,-0.6));
#81774=CARTESIAN_POINT('Ctrl Pts',(-9.9576411023736,-53.5241476893425,-0.9));
#81775=CARTESIAN_POINT('Ctrl Pts',(-10.0851974263787,-53.3618007302284,
-0.6));
#81776=CARTESIAN_POINT('Ctrl Pts',(-10.0851974263787,-53.3618007302284,
-0.9));
#81777=CARTESIAN_POINT('Ctrl Pts',(-10.1860842481256,-53.2968620657921,
-0.6));
#81778=CARTESIAN_POINT('Ctrl Pts',(-10.1860842481256,-53.2968620657921,
-0.9));
#81779=CARTESIAN_POINT('',(-9.9576411023736,-53.5241476893425,-0.6));
#81780=CARTESIAN_POINT('Ctrl Pts',(-9.9576411023736,-53.5241476893425,-0.6));
#81781=CARTESIAN_POINT('Ctrl Pts',(-10.0851974263787,-53.3618007302284,
-0.6));
#81782=CARTESIAN_POINT('Ctrl Pts',(-10.1860842481256,-53.2968620657921,
-0.6));
#81783=CARTESIAN_POINT('',(-9.9576411023736,-53.5241476893425,-0.9));
#81784=CARTESIAN_POINT('',(-9.9576411023736,-53.5241476893425,-0.6));
#81785=CARTESIAN_POINT('Ctrl Pts',(-9.9576411023736,-53.5241476893425,-0.9));
#81786=CARTESIAN_POINT('Ctrl Pts',(-10.0851974263787,-53.3618007302284,
-0.9));
#81787=CARTESIAN_POINT('Ctrl Pts',(-10.1860842481256,-53.2968620657921,
-0.9));
#81788=CARTESIAN_POINT('Ctrl Pts',(-9.63294837623835,-53.9926330447197,
-0.6));
#81789=CARTESIAN_POINT('Ctrl Pts',(-9.63294837623835,-53.9926330447197,
-0.9));
#81790=CARTESIAN_POINT('Ctrl Pts',(-9.83008239418268,-53.6864940524101,
-0.6));
#81791=CARTESIAN_POINT('Ctrl Pts',(-9.83008239418268,-53.6864940524101,
-0.9));
#81792=CARTESIAN_POINT('Ctrl Pts',(-9.9576411023736,-53.5241476893425,-0.6));
#81793=CARTESIAN_POINT('Ctrl Pts',(-9.9576411023736,-53.5241476893425,-0.9));
#81794=CARTESIAN_POINT('',(-9.63294837623835,-53.9926330447197,-0.6));
#81795=CARTESIAN_POINT('Ctrl Pts',(-9.63294837623835,-53.9926330447197,
-0.6));
#81796=CARTESIAN_POINT('Ctrl Pts',(-9.83008239418268,-53.6864940524101,
-0.6));
#81797=CARTESIAN_POINT('Ctrl Pts',(-9.9576411023736,-53.5241476893425,-0.6));
#81798=CARTESIAN_POINT('',(-9.63294837623835,-53.9926330447197,-0.9));
#81799=CARTESIAN_POINT('',(-9.63294837623835,-53.9926330447197,-0.6));
#81800=CARTESIAN_POINT('Ctrl Pts',(-9.63294837623835,-53.9926330447197,
-0.9));
#81801=CARTESIAN_POINT('Ctrl Pts',(-9.83008239418268,-53.6864940524101,
-0.9));
#81802=CARTESIAN_POINT('Ctrl Pts',(-9.9576411023736,-53.5241476893425,-0.9));
#81803=CARTESIAN_POINT('Origin',(-9.18301437050104,-54.7000001072884,-0.6));
#81804=CARTESIAN_POINT('',(-9.18301437050104,-54.7000001072884,-0.6));
#81805=CARTESIAN_POINT('',(-8.24537770178333,-56.174112505218,-0.6));
#81806=CARTESIAN_POINT('',(-9.18301437050104,-54.7000001072884,-0.9));
#81807=CARTESIAN_POINT('',(-9.18301437050104,-54.7000001072884,-0.6));
#81808=CARTESIAN_POINT('',(-9.18301437050104,-54.7000001072884,-0.9));
#81809=CARTESIAN_POINT('Origin',(-8.6171231046319,-54.7000001072884,-0.6));
#81810=CARTESIAN_POINT('',(-8.6171231046319,-54.7000001072884,-0.6));
#81811=CARTESIAN_POINT('',(-4.30856155231595,-54.7000001072884,-0.6));
#81812=CARTESIAN_POINT('',(-8.6171231046319,-54.7000001072884,-0.9));
#81813=CARTESIAN_POINT('',(-8.6171231046319,-54.7000001072884,-0.6));
#81814=CARTESIAN_POINT('',(-8.6171231046319,-54.7000001072884,-0.9));
#81815=CARTESIAN_POINT('Origin',(-9.2085275426507,-53.7746248841286,-0.6));
#81816=CARTESIAN_POINT('',(-9.2085275426507,-53.7746248841286,-0.6));
#81817=CARTESIAN_POINT('',(-8.0490517968636,-55.5888657961523,-0.6));
#81818=CARTESIAN_POINT('',(-9.2085275426507,-53.7746248841286,-0.9));
#81819=CARTESIAN_POINT('',(-9.2085275426507,-53.7746248841286,-0.6));
#81820=CARTESIAN_POINT('',(-9.2085275426507,-53.7746248841286,-0.9));
#81821=CARTESIAN_POINT('Ctrl Pts',(-9.58192441612482,-53.3223740458488,
-0.6));
#81822=CARTESIAN_POINT('Ctrl Pts',(-9.58192441612482,-53.3223740458488,
-0.9));
#81823=CARTESIAN_POINT('Ctrl Pts',(-9.38478801399469,-53.5032741427422,
-0.6));
#81824=CARTESIAN_POINT('Ctrl Pts',(-9.38478801399469,-53.5032741427422,
-0.9));
#81825=CARTESIAN_POINT('Ctrl Pts',(-9.2085275426507,-53.7746248841286,-0.6));
#81826=CARTESIAN_POINT('Ctrl Pts',(-9.2085275426507,-53.7746248841286,-0.9));
#81827=CARTESIAN_POINT('',(-9.58192441612482,-53.3223740458488,-0.6));
#81828=CARTESIAN_POINT('Ctrl Pts',(-9.58192441612482,-53.3223740458488,
-0.6));
#81829=CARTESIAN_POINT('Ctrl Pts',(-9.38478801399469,-53.5032741427422,
-0.6));
#81830=CARTESIAN_POINT('Ctrl Pts',(-9.2085275426507,-53.7746248841286,-0.6));
#81831=CARTESIAN_POINT('',(-9.58192441612482,-53.3223740458488,-0.9));
#81832=CARTESIAN_POINT('',(-9.58192441612482,-53.3223740458488,-0.6));
#81833=CARTESIAN_POINT('Ctrl Pts',(-9.58192441612482,-53.3223740458488,
-0.9));
#81834=CARTESIAN_POINT('Ctrl Pts',(-9.38478801399469,-53.5032741427422,
-0.9));
#81835=CARTESIAN_POINT('Ctrl Pts',(-9.2085275426507,-53.7746248841286,-0.9));
#81836=CARTESIAN_POINT('Ctrl Pts',(-9.85327575355768,-53.1530694365501,
-0.6));
#81837=CARTESIAN_POINT('Ctrl Pts',(-9.85327575355768,-53.1530694365501,
-0.9));
#81838=CARTESIAN_POINT('Ctrl Pts',(-9.67469308525324,-53.2388810515404,
-0.6));
#81839=CARTESIAN_POINT('Ctrl Pts',(-9.67469308525324,-53.2388810515404,
-0.9));
#81840=CARTESIAN_POINT('Ctrl Pts',(-9.58192441612482,-53.3223740458488,
-0.6));
#81841=CARTESIAN_POINT('Ctrl Pts',(-9.58192441612482,-53.3223740458488,
-0.9));
#81842=CARTESIAN_POINT('',(-9.85327575355768,-53.1530694365501,-0.6));
#81843=CARTESIAN_POINT('Ctrl Pts',(-9.85327575355768,-53.1530694365501,
-0.6));
#81844=CARTESIAN_POINT('Ctrl Pts',(-9.67469308525324,-53.2388810515404,
-0.6));
#81845=CARTESIAN_POINT('Ctrl Pts',(-9.58192441612482,-53.3223740458488,
-0.6));
#81846=CARTESIAN_POINT('',(-9.85327575355768,-53.1530694365501,-0.9));
#81847=CARTESIAN_POINT('',(-9.85327575355768,-53.1530694365501,-0.6));
#81848=CARTESIAN_POINT('Ctrl Pts',(-9.85327575355768,-53.1530694365501,
-0.9));
#81849=CARTESIAN_POINT('Ctrl Pts',(-9.67469308525324,-53.2388810515404,
-0.9));
#81850=CARTESIAN_POINT('Ctrl Pts',(-9.58192441612482,-53.3223740458488,
-0.9));
#81851=CARTESIAN_POINT('Ctrl Pts',(-9.12967298179865,-52.8376535773277,
-0.6));
#81852=CARTESIAN_POINT('Ctrl Pts',(-9.12967298179865,-52.8376535773277,
-0.9));
#81853=CARTESIAN_POINT('Ctrl Pts',(-9.36391685158014,-53.0858115553856,
-0.6));
#81854=CARTESIAN_POINT('Ctrl Pts',(-9.36391685158014,-53.0858115553856,
-0.9));
#81855=CARTESIAN_POINT('Ctrl Pts',(-9.85327575355768,-53.1530694365501,
-0.6));
#81856=CARTESIAN_POINT('Ctrl Pts',(-9.85327575355768,-53.1530694365501,
-0.9));
#81857=CARTESIAN_POINT('',(-9.12967298179865,-52.8376535773277,-0.6));
#81858=CARTESIAN_POINT('Ctrl Pts',(-9.12967298179865,-52.8376535773277,
-0.6));
#81859=CARTESIAN_POINT('Ctrl Pts',(-9.36391685158014,-53.0858115553856,
-0.6));
#81860=CARTESIAN_POINT('Ctrl Pts',(-9.85327575355768,-53.1530694365501,
-0.6));
#81861=CARTESIAN_POINT('',(-9.12967298179865,-52.8376535773277,-0.9));
#81862=CARTESIAN_POINT('',(-9.12967298179865,-52.8376535773277,-0.6));
#81863=CARTESIAN_POINT('Ctrl Pts',(-9.12967298179865,-52.8376535773277,
-0.9));
#81864=CARTESIAN_POINT('Ctrl Pts',(-9.36391685158014,-53.0858115553856,
-0.9));
#81865=CARTESIAN_POINT('Ctrl Pts',(-9.85327575355768,-53.1530694365501,
-0.9));
#81866=CARTESIAN_POINT('Ctrl Pts',(-8.89542911201715,-52.2276942133904,
-0.6));
#81867=CARTESIAN_POINT('Ctrl Pts',(-8.89542911201715,-52.2276942133904,
-0.9));
#81868=CARTESIAN_POINT('Ctrl Pts',(-8.89542911201715,-52.5894955992699,
-0.6));
#81869=CARTESIAN_POINT('Ctrl Pts',(-8.89542911201715,-52.5894955992699,
-0.9));
#81870=CARTESIAN_POINT('Ctrl Pts',(-9.12967298179865,-52.8376535773277,
-0.6));
#81871=CARTESIAN_POINT('Ctrl Pts',(-9.12967298179865,-52.8376535773277,
-0.9));
#81872=CARTESIAN_POINT('',(-8.89542911201715,-52.2276942133904,-0.6));
#81873=CARTESIAN_POINT('Ctrl Pts',(-8.89542911201715,-52.2276942133904,
-0.6));
#81874=CARTESIAN_POINT('Ctrl Pts',(-8.89542911201715,-52.5894955992699,
-0.6));
#81875=CARTESIAN_POINT('Ctrl Pts',(-9.12967298179865,-52.8376535773277,
-0.6));
#81876=CARTESIAN_POINT('',(-8.89542911201715,-52.2276942133904,-0.9));
#81877=CARTESIAN_POINT('',(-8.89542911201715,-52.2276942133904,-0.6));
#81878=CARTESIAN_POINT('Ctrl Pts',(-8.89542911201715,-52.2276942133904,
-0.9));
#81879=CARTESIAN_POINT('Ctrl Pts',(-8.89542911201715,-52.5894955992699,
-0.9));
#81880=CARTESIAN_POINT('Ctrl Pts',(-9.12967298179865,-52.8376535773277,
-0.9));
#81881=CARTESIAN_POINT('Ctrl Pts',(-9.03690431267023,-51.7151431441307,
-0.6));
#81882=CARTESIAN_POINT('Ctrl Pts',(-9.03690431267023,-51.7151431441307,
-0.9));
#81883=CARTESIAN_POINT('Ctrl Pts',(-8.89542911201715,-51.9470672011375,
-0.6));
#81884=CARTESIAN_POINT('Ctrl Pts',(-8.89542911201715,-51.9470672011375,
-0.9));
#81885=CARTESIAN_POINT('Ctrl Pts',(-8.89542911201715,-52.2276942133904,
-0.6));
#81886=CARTESIAN_POINT('Ctrl Pts',(-8.89542911201715,-52.2276942133904,
-0.9));
#81887=CARTESIAN_POINT('',(-9.03690431267023,-51.7151431441307,-0.6));
#81888=CARTESIAN_POINT('Ctrl Pts',(-9.03690431267023,-51.7151431441307,
-0.6));
#81889=CARTESIAN_POINT('Ctrl Pts',(-8.89542911201715,-51.9470672011375,
-0.6));
#81890=CARTESIAN_POINT('Ctrl Pts',(-8.89542911201715,-52.2276942133904,
-0.6));
#81891=CARTESIAN_POINT('',(-9.03690431267023,-51.7151431441307,-0.9));
#81892=CARTESIAN_POINT('',(-9.03690431267023,-51.7151431441307,-0.6));
#81893=CARTESIAN_POINT('Ctrl Pts',(-9.03690431267023,-51.7151431441307,
-0.9));
#81894=CARTESIAN_POINT('Ctrl Pts',(-8.89542911201715,-51.9470672011375,
-0.9));
#81895=CARTESIAN_POINT('Ctrl Pts',(-8.89542911201715,-52.2276942133904,
-0.9));
#81896=CARTESIAN_POINT('Ctrl Pts',(-9.41493842750788,-51.3916097283363,
-0.6));
#81897=CARTESIAN_POINT('Ctrl Pts',(-9.41493842750788,-51.3916097283363,
-0.9));
#81898=CARTESIAN_POINT('Ctrl Pts',(-9.17837712913752,-51.4832196831703,
-0.6));
#81899=CARTESIAN_POINT('Ctrl Pts',(-9.17837712913752,-51.4832196831703,
-0.9));
#81900=CARTESIAN_POINT('Ctrl Pts',(-9.03690431267023,-51.7151431441307,
-0.6));
#81901=CARTESIAN_POINT('Ctrl Pts',(-9.03690431267023,-51.7151431441307,
-0.9));
#81902=CARTESIAN_POINT('',(-9.41493842750788,-51.3916097283363,-0.6));
#81903=CARTESIAN_POINT('Ctrl Pts',(-9.41493842750788,-51.3916097283363,
-0.6));
#81904=CARTESIAN_POINT('Ctrl Pts',(-9.17837712913752,-51.4832196831703,
-0.6));
#81905=CARTESIAN_POINT('Ctrl Pts',(-9.03690431267023,-51.7151431441307,
-0.6));
#81906=CARTESIAN_POINT('',(-9.41493842750788,-51.3916097283363,-0.9));
#81907=CARTESIAN_POINT('',(-9.41493842750788,-51.3916097283363,-0.6));
#81908=CARTESIAN_POINT('Ctrl Pts',(-9.41493842750788,-51.3916097283363,
-0.9));
#81909=CARTESIAN_POINT('Ctrl Pts',(-9.17837712913752,-51.4832196831703,
-0.9));
#81910=CARTESIAN_POINT('Ctrl Pts',(-9.03690431267023,-51.7151431441307,
-0.9));
#81911=CARTESIAN_POINT('Ctrl Pts',(-10.1060709729791,-51.3000003695488,
-0.6));
#81912=CARTESIAN_POINT('Ctrl Pts',(-10.1060709729791,-51.3000003695488,
-0.9));
#81913=CARTESIAN_POINT('Ctrl Pts',(-9.65150211006403,-51.3000003695488,
-0.6));
#81914=CARTESIAN_POINT('Ctrl Pts',(-9.65150211006403,-51.3000003695488,
-0.9));
#81915=CARTESIAN_POINT('Ctrl Pts',(-9.41493842750788,-51.3916097283363,
-0.6));
#81916=CARTESIAN_POINT('Ctrl Pts',(-9.41493842750788,-51.3916097283363,
-0.9));
#81917=CARTESIAN_POINT('',(-10.1060709729791,-51.3000003695488,-0.6));
#81918=CARTESIAN_POINT('Ctrl Pts',(-10.1060709729791,-51.3000003695488,
-0.6));
#81919=CARTESIAN_POINT('Ctrl Pts',(-9.65150211006403,-51.3000003695488,
-0.6));
#81920=CARTESIAN_POINT('Ctrl Pts',(-9.41493842750788,-51.3916097283363,
-0.6));
#81921=CARTESIAN_POINT('',(-10.1060709729791,-51.3000003695488,-0.9));
#81922=CARTESIAN_POINT('',(-10.1060709729791,-51.3000003695488,-0.6));
#81923=CARTESIAN_POINT('Ctrl Pts',(-10.1060709729791,-51.3000003695488,
-0.9));
#81924=CARTESIAN_POINT('Ctrl Pts',(-9.65150211006403,-51.3000003695488,
-0.9));
#81925=CARTESIAN_POINT('Ctrl Pts',(-9.41493842750788,-51.3916097283363,
-0.9));
#81926=CARTESIAN_POINT('Origin',(-11.6135749593377,-51.3000003695488,-0.6));
#81927=CARTESIAN_POINT('',(-11.6135749593377,-51.3000003695488,-0.6));
#81928=CARTESIAN_POINT('',(-5.80678747966886,-51.3000003695488,-0.6));
#81929=CARTESIAN_POINT('',(-11.6135749593377,-51.3000003695488,-0.9));
#81930=CARTESIAN_POINT('',(-11.6135749593377,-51.3000003695488,-0.6));
#81931=CARTESIAN_POINT('',(-11.6135749593377,-51.3000003695488,-0.9));
#81932=CARTESIAN_POINT('Origin',(-11.6135749593377,-54.7000001072884,-0.6));
#81933=CARTESIAN_POINT('',(-11.6135749593377,-54.7000001072884,-0.6));
#81934=CARTESIAN_POINT('',(-11.6135749593377,-53.8500000536442,-0.6));
#81935=CARTESIAN_POINT('',(-11.6135749593377,-54.7000001072884,-0.9));
#81936=CARTESIAN_POINT('',(-11.6135749593377,-54.7000001072884,-0.6));
#81937=CARTESIAN_POINT('',(-11.6135749593377,-54.7000001072884,-0.9));
#81938=CARTESIAN_POINT('Origin',(-11.1636433377862,-54.7000001072884,-0.6));
#81939=CARTESIAN_POINT('',(-11.1636433377862,-54.7000001072884,-0.6));
#81940=CARTESIAN_POINT('',(-5.5818216688931,-54.7000001072884,-0.6));
#81941=CARTESIAN_POINT('',(-11.1636433377862,-54.7000001072884,-0.9));
#81942=CARTESIAN_POINT('',(-11.1636433377862,-54.7000001072884,-0.6));
#81943=CARTESIAN_POINT('',(-11.1636433377862,-54.7000001072884,-0.9));
#81944=CARTESIAN_POINT('Origin',(-11.1636433377862,-53.190177500248,-0.6));
#81945=CARTESIAN_POINT('',(-11.1636433377862,-53.095088750124,-0.6));
#81946=CARTESIAN_POINT('',(-11.1636433377862,-53.190177500248,-0.9));
#81947=CARTESIAN_POINT('Origin',(-10.1153490319848,-53.0000002384186,-0.9));
#81948=CARTESIAN_POINT('Origin',(-15.6907925382257,-51.7012278437614,-0.6));
#81949=CARTESIAN_POINT('',(-15.6907925382257,-51.7012278437614,-0.6));
#81950=CARTESIAN_POINT('',(-16.8156227841973,-51.7012278437614,-0.6));
#81951=CARTESIAN_POINT('',(-7.84539626911283,-51.7012278437614,-0.6));
#81952=CARTESIAN_POINT('',(-15.6907925382257,-51.7012278437614,-0.9));
#81953=CARTESIAN_POINT('',(-15.6907925382257,-51.7012278437614,-0.6));
#81954=CARTESIAN_POINT('',(-16.8156227841973,-51.7012278437614,-0.9));
#81955=CARTESIAN_POINT('',(-15.6907925382257,-51.7012278437614,-0.9));
#81956=CARTESIAN_POINT('',(-16.8156227841973,-51.7012278437614,-0.6));
#81957=CARTESIAN_POINT('Origin',(-15.6907925382257,-51.3000003695488,-0.6));
#81958=CARTESIAN_POINT('',(-15.6907925382257,-51.3000003695488,-0.6));
#81959=CARTESIAN_POINT('',(-15.6907925382257,-52.1500001847744,-0.6));
#81960=CARTESIAN_POINT('',(-15.6907925382257,-51.3000003695488,-0.9));
#81961=CARTESIAN_POINT('',(-15.6907925382257,-51.3000003695488,-0.6));
#81962=CARTESIAN_POINT('',(-15.6907925382257,-51.3000003695488,-0.9));
#81963=CARTESIAN_POINT('Origin',(-18.3857450261712,-51.3000003695488,-0.6));
#81964=CARTESIAN_POINT('',(-18.3857450261712,-51.3000003695488,-0.6));
#81965=CARTESIAN_POINT('',(-9.1928725130856,-51.3000003695488,-0.6));
#81966=CARTESIAN_POINT('',(-18.3857450261712,-51.3000003695488,-0.9));
#81967=CARTESIAN_POINT('',(-18.3857450261712,-51.3000003695488,-0.6));
#81968=CARTESIAN_POINT('',(-18.3857450261712,-51.3000003695488,-0.9));
#81969=CARTESIAN_POINT('Origin',(-18.3857450261712,-51.7012278437614,-0.6));
#81970=CARTESIAN_POINT('',(-18.3857450261712,-51.7012278437614,-0.6));
#81971=CARTESIAN_POINT('',(-18.3857450261712,-52.3506139218807,-0.6));
#81972=CARTESIAN_POINT('',(-18.3857450261712,-51.7012278437614,-0.9));
#81973=CARTESIAN_POINT('',(-18.3857450261712,-51.7012278437614,-0.6));
#81974=CARTESIAN_POINT('',(-18.3857450261712,-51.7012278437614,-0.9));
#81975=CARTESIAN_POINT('Origin',(-17.2655544057488,-51.7012278437614,-0.6));
#81976=CARTESIAN_POINT('',(-17.2655544057488,-51.7012278437614,-0.6));
#81977=CARTESIAN_POINT('',(-8.63277720287442,-51.7012278437614,-0.6));
#81978=CARTESIAN_POINT('',(-17.2655544057488,-51.7012278437614,-0.9));
#81979=CARTESIAN_POINT('',(-17.2655544057488,-51.7012278437614,-0.6));
#81980=CARTESIAN_POINT('',(-17.2655544057488,-51.7012278437614,-0.9));
#81981=CARTESIAN_POINT('Origin',(-17.2655544057488,-54.7000001072884,-0.6));
#81982=CARTESIAN_POINT('',(-17.2655544057488,-54.7000001072884,-0.6));
#81983=CARTESIAN_POINT('',(-17.2655544057488,-53.8500000536442,-0.6));
#81984=CARTESIAN_POINT('',(-17.2655544057488,-54.7000001072884,-0.9));
#81985=CARTESIAN_POINT('',(-17.2655544057488,-54.7000001072884,-0.6));
#81986=CARTESIAN_POINT('',(-17.2655544057488,-54.7000001072884,-0.9));
#81987=CARTESIAN_POINT('Origin',(-16.8156227841973,-54.7000001072884,-0.6));
#81988=CARTESIAN_POINT('',(-16.8156227841973,-54.7000001072884,-0.6));
#81989=CARTESIAN_POINT('',(-8.40781139209867,-54.7000001072884,-0.6));
#81990=CARTESIAN_POINT('',(-16.8156227841973,-54.7000001072884,-0.9));
#81991=CARTESIAN_POINT('',(-16.8156227841973,-54.7000001072884,-0.6));
#81992=CARTESIAN_POINT('',(-16.8156227841973,-54.7000001072884,-0.9));
#81993=CARTESIAN_POINT('Origin',(-16.8156227841973,-51.7012278437614,-0.6));
#81994=CARTESIAN_POINT('',(-16.8156227841973,-52.3506139218807,-0.6));
#81995=CARTESIAN_POINT('',(-16.8156227841973,-51.7012278437614,-0.9));
#81996=CARTESIAN_POINT('Origin',(-17.0382687821984,-53.0000002384186,-0.9));
#81997=CARTESIAN_POINT('Ctrl Pts',(-23.8846537843347,-51.7406551241875,
-0.6));
#81998=CARTESIAN_POINT('Ctrl Pts',(-23.8846537843347,-51.7406551241875,
-0.9));
#81999=CARTESIAN_POINT('Ctrl Pts',(-23.6225793138146,-51.5064118504524,
-0.6));
#82000=CARTESIAN_POINT('Ctrl Pts',(-23.6225793138146,-51.5064118504524,
-0.9));
#82001=CARTESIAN_POINT('Ctrl Pts',(-23.5135755315423,-51.2860844731331,
-0.6));
#82002=CARTESIAN_POINT('Ctrl Pts',(-23.5135755315423,-51.2860844731331,
-0.9));
#82003=CARTESIAN_POINT('',(-23.8846537843347,-51.7406551241875,-0.6));
#82004=CARTESIAN_POINT('',(-23.5135755315423,-51.2860844731331,-0.6));
#82005=CARTESIAN_POINT('Ctrl Pts',(-23.8846537843347,-51.7406551241875,
-0.6));
#82006=CARTESIAN_POINT('Ctrl Pts',(-23.6225793138146,-51.5064118504524,
-0.6));
#82007=CARTESIAN_POINT('Ctrl Pts',(-23.5135755315423,-51.2860844731331,
-0.6));
#82008=CARTESIAN_POINT('',(-23.8846537843347,-51.7406551241875,-0.9));
#82009=CARTESIAN_POINT('',(-23.8846537843347,-51.7406551241875,-0.6));
#82010=CARTESIAN_POINT('',(-23.5135755315423,-51.2860844731331,-0.9));
#82011=CARTESIAN_POINT('Ctrl Pts',(-23.8846537843347,-51.7406551241875,
-0.9));
#82012=CARTESIAN_POINT('Ctrl Pts',(-23.6225793138146,-51.5064118504524,
-0.9));
#82013=CARTESIAN_POINT('Ctrl Pts',(-23.5135755315423,-51.2860844731331,
-0.9));
#82014=CARTESIAN_POINT('',(-23.5135755315423,-51.2860844731331,-0.6));
#82015=CARTESIAN_POINT('Ctrl Pts',(-24.4969317689538,-52.1395633816719,
-0.6));
#82016=CARTESIAN_POINT('Ctrl Pts',(-24.4969317689538,-52.1395633816719,
-0.9));
#82017=CARTESIAN_POINT('Ctrl Pts',(-24.1467270627618,-51.9748978018761,
-0.6));
#82018=CARTESIAN_POINT('Ctrl Pts',(-24.1467270627618,-51.9748978018761,
-0.9));
#82019=CARTESIAN_POINT('Ctrl Pts',(-23.8846537843347,-51.7406551241875,
-0.6));
#82020=CARTESIAN_POINT('Ctrl Pts',(-23.8846537843347,-51.7406551241875,
-0.9));
#82021=CARTESIAN_POINT('',(-24.4969317689538,-52.1395633816719,-0.6));
#82022=CARTESIAN_POINT('Ctrl Pts',(-24.4969317689538,-52.1395633816719,
-0.6));
#82023=CARTESIAN_POINT('Ctrl Pts',(-24.1467270627618,-51.9748978018761,
-0.6));
#82024=CARTESIAN_POINT('Ctrl Pts',(-23.8846537843347,-51.7406551241875,
-0.6));
#82025=CARTESIAN_POINT('',(-24.4969317689538,-52.1395633816719,-0.9));
#82026=CARTESIAN_POINT('',(-24.4969317689538,-52.1395633816719,-0.6));
#82027=CARTESIAN_POINT('Ctrl Pts',(-24.4969317689538,-52.1395633816719,
-0.9));
#82028=CARTESIAN_POINT('Ctrl Pts',(-24.1467270627618,-51.9748978018761,
-0.9));
#82029=CARTESIAN_POINT('Ctrl Pts',(-23.8846537843347,-51.7406551241875,
-0.9));
#82030=CARTESIAN_POINT('Origin',(-24.4969317689538,-52.5431100726128,-0.6));
#82031=CARTESIAN_POINT('',(-24.4969317689538,-52.5431100726128,-0.6));
#82032=CARTESIAN_POINT('',(-24.4969317689538,-52.7715550363062,-0.6));
#82033=CARTESIAN_POINT('',(-24.4969317689538,-52.5431100726128,-0.9));
#82034=CARTESIAN_POINT('',(-24.4969317689538,-52.5431100726128,-0.6));
#82035=CARTESIAN_POINT('',(-24.4969317689538,-52.5431100726128,-0.9));
#82036=CARTESIAN_POINT('Ctrl Pts',(-24.0574369207025,-52.3274211287498,
-0.6));
#82037=CARTESIAN_POINT('Ctrl Pts',(-24.0574369207025,-52.3274211287498,
-0.9));
#82038=CARTESIAN_POINT('Ctrl Pts',(-24.3021163716912,-52.4712137579918,
-0.6));
#82039=CARTESIAN_POINT('Ctrl Pts',(-24.3021163716912,-52.4712137579918,
-0.9));
#82040=CARTESIAN_POINT('Ctrl Pts',(-24.4969317689538,-52.5431100726128,
-0.6));
#82041=CARTESIAN_POINT('Ctrl Pts',(-24.4969317689538,-52.5431100726128,
-0.9));
#82042=CARTESIAN_POINT('',(-24.0574369207025,-52.3274211287498,-0.6));
#82043=CARTESIAN_POINT('Ctrl Pts',(-24.0574369207025,-52.3274211287498,
-0.6));
#82044=CARTESIAN_POINT('Ctrl Pts',(-24.3021163716912,-52.4712137579918,
-0.6));
#82045=CARTESIAN_POINT('Ctrl Pts',(-24.4969317689538,-52.5431100726128,
-0.6));
#82046=CARTESIAN_POINT('',(-24.0574369207025,-52.3274211287498,-0.9));
#82047=CARTESIAN_POINT('',(-24.0574369207025,-52.3274211287498,-0.6));
#82048=CARTESIAN_POINT('Ctrl Pts',(-24.0574369207025,-52.3274211287498,
-0.9));
#82049=CARTESIAN_POINT('Ctrl Pts',(-24.3021163716912,-52.4712137579918,
-0.9));
#82050=CARTESIAN_POINT('Ctrl Pts',(-24.4969317689538,-52.5431100726128,
-0.9));
#82051=CARTESIAN_POINT('Ctrl Pts',(-23.6620065942407,-52.039835870266,-0.6));
#82052=CARTESIAN_POINT('Ctrl Pts',(-23.6620065942407,-52.039835870266,-0.9));
#82053=CARTESIAN_POINT('Ctrl Pts',(-23.8127574697137,-52.1836284995079,
-0.6));
#82054=CARTESIAN_POINT('Ctrl Pts',(-23.8127574697137,-52.1836284995079,
-0.9));
#82055=CARTESIAN_POINT('Ctrl Pts',(-24.0574369207025,-52.3274211287498,
-0.6));
#82056=CARTESIAN_POINT('Ctrl Pts',(-24.0574369207025,-52.3274211287498,
-0.9));
#82057=CARTESIAN_POINT('',(-23.6620065942407,-52.039835870266,-0.6));
#82058=CARTESIAN_POINT('Ctrl Pts',(-23.6620065942407,-52.039835870266,-0.6));
#82059=CARTESIAN_POINT('Ctrl Pts',(-23.8127574697137,-52.1836284995079,
-0.6));
#82060=CARTESIAN_POINT('Ctrl Pts',(-24.0574369207025,-52.3274211287498,
-0.6));
#82061=CARTESIAN_POINT('',(-23.6620065942407,-52.039835870266,-0.9));
#82062=CARTESIAN_POINT('',(-23.6620065942407,-52.039835870266,-0.6));
#82063=CARTESIAN_POINT('Ctrl Pts',(-23.6620065942407,-52.039835870266,-0.9));
#82064=CARTESIAN_POINT('Ctrl Pts',(-23.8127574697137,-52.1836284995079,
-0.9));
#82065=CARTESIAN_POINT('Ctrl Pts',(-24.0574369207025,-52.3274211287498,
-0.9));
#82066=CARTESIAN_POINT('Origin',(-23.6620065942407,-54.7000001072884,-0.6));
#82067=CARTESIAN_POINT('',(-23.6620065942407,-54.7000001072884,-0.6));
#82068=CARTESIAN_POINT('',(-23.6620065942407,-53.8500000536442,-0.6));
#82069=CARTESIAN_POINT('',(-23.6620065942407,-54.7000001072884,-0.9));
#82070=CARTESIAN_POINT('',(-23.6620065942407,-54.7000001072884,-0.6));
#82071=CARTESIAN_POINT('',(-23.6620065942407,-54.7000001072884,-0.9));
#82072=CARTESIAN_POINT('Origin',(-23.2445440068841,-54.7000001072884,-0.6));
#82073=CARTESIAN_POINT('',(-23.2445440068841,-54.7000001072884,-0.6));
#82074=CARTESIAN_POINT('',(-11.622272003442,-54.7000001072884,-0.6));
#82075=CARTESIAN_POINT('',(-23.2445440068841,-54.7000001072884,-0.9));
#82076=CARTESIAN_POINT('',(-23.2445440068841,-54.7000001072884,-0.6));
#82077=CARTESIAN_POINT('',(-23.2445440068841,-54.7000001072884,-0.9));
#82078=CARTESIAN_POINT('Origin',(-23.2445440068841,-51.2860844731331,-0.6));
#82079=CARTESIAN_POINT('',(-23.2445440068841,-51.2860844731331,-0.6));
#82080=CARTESIAN_POINT('',(-23.2445440068841,-52.1430422365665,-0.6));
#82081=CARTESIAN_POINT('',(-23.2445440068841,-51.2860844731331,-0.9));
#82082=CARTESIAN_POINT('',(-23.2445440068841,-51.2860844731331,-0.6));
#82083=CARTESIAN_POINT('',(-23.2445440068841,-51.2860844731331,-0.9));
#82084=CARTESIAN_POINT('Origin',(-23.5135755315423,-51.2860844731331,-0.6));
#82085=CARTESIAN_POINT('',(-11.7567877657712,-51.2860844731331,-0.6));
#82086=CARTESIAN_POINT('',(-23.5135755315423,-51.2860844731331,-0.9));
#82087=CARTESIAN_POINT('Origin',(-23.8707378879189,-52.9930422902107,-0.9));
#82088=CARTESIAN_POINT('Ctrl Pts',(-27.3136434331536,-54.5573667883873,
-0.6));
#82089=CARTESIAN_POINT('Ctrl Pts',(-27.3136434331536,-54.5573667883873,
-0.9));
#82090=CARTESIAN_POINT('Ctrl Pts',(-27.5583228841424,-54.7579811215401,
-0.6));
#82091=CARTESIAN_POINT('Ctrl Pts',(-27.5583228841424,-54.7579811215401,
-0.9));
#82092=CARTESIAN_POINT('Ctrl Pts',(-27.9317197576165,-54.7579811215401,
-0.6));
#82093=CARTESIAN_POINT('Ctrl Pts',(-27.9317197576165,-54.7579811215401,
-0.9));
#82094=CARTESIAN_POINT('',(-27.3136434331536,-54.5573667883873,-0.6));
#82095=CARTESIAN_POINT('',(-27.9317197576165,-54.7579811215401,-0.6));
#82096=CARTESIAN_POINT('Ctrl Pts',(-27.3136434331536,-54.5573667883873,
-0.6));
#82097=CARTESIAN_POINT('Ctrl Pts',(-27.5583228841424,-54.7579811215401,
-0.6));
#82098=CARTESIAN_POINT('Ctrl Pts',(-27.9317197576165,-54.7579811215401,
-0.6));
#82099=CARTESIAN_POINT('',(-27.3136434331536,-54.5573667883873,-0.9));
#82100=CARTESIAN_POINT('',(-27.3136434331536,-54.5573667883873,-0.6));
#82101=CARTESIAN_POINT('',(-27.9317197576165,-54.7579811215401,-0.9));
#82102=CARTESIAN_POINT('Ctrl Pts',(-27.3136434331536,-54.5573667883873,
-0.9));
#82103=CARTESIAN_POINT('Ctrl Pts',(-27.5583228841424,-54.7579811215401,
-0.9));
#82104=CARTESIAN_POINT('Ctrl Pts',(-27.9317197576165,-54.7579811215401,
-0.9));
#82105=CARTESIAN_POINT('',(-27.9317197576165,-54.7579811215401,-0.6));
#82106=CARTESIAN_POINT('Ctrl Pts',(-26.9460448995233,-53.9891545176506,
-0.6));
#82107=CARTESIAN_POINT('Ctrl Pts',(-26.9460448995233,-53.9891545176506,
-0.9));
#82108=CARTESIAN_POINT('Ctrl Pts',(-27.0689639821649,-54.356753051281,-0.6));
#82109=CARTESIAN_POINT('Ctrl Pts',(-27.0689639821649,-54.356753051281,-0.9));
#82110=CARTESIAN_POINT('Ctrl Pts',(-27.3136434331536,-54.5573667883873,
-0.6));
#82111=CARTESIAN_POINT('Ctrl Pts',(-27.3136434331536,-54.5573667883873,
-0.9));
#82112=CARTESIAN_POINT('',(-26.9460448995233,-53.9891545176506,-0.6));
#82113=CARTESIAN_POINT('Ctrl Pts',(-26.9460448995233,-53.9891545176506,
-0.6));
#82114=CARTESIAN_POINT('Ctrl Pts',(-27.0689639821649,-54.356753051281,-0.6));
#82115=CARTESIAN_POINT('Ctrl Pts',(-27.3136434331536,-54.5573667883873,
-0.6));
#82116=CARTESIAN_POINT('',(-26.9460448995233,-53.9891545176506,-0.9));
#82117=CARTESIAN_POINT('',(-26.9460448995233,-53.9891545176506,-0.6));
#82118=CARTESIAN_POINT('Ctrl Pts',(-26.9460448995233,-53.9891545176506,
-0.9));
#82119=CARTESIAN_POINT('Ctrl Pts',(-27.0689639821649,-54.356753051281,-0.9));
#82120=CARTESIAN_POINT('Ctrl Pts',(-27.3136434331536,-54.5573667883873,
-0.9));
#82121=CARTESIAN_POINT('Ctrl Pts',(-26.8231252208352,-53.0231921076775,
-0.6));
#82122=CARTESIAN_POINT('Ctrl Pts',(-26.8231252208352,-53.0231921076775,
-0.9));
#82123=CARTESIAN_POINT('Ctrl Pts',(-26.8231252208352,-53.6215553879738,
-0.6));
#82124=CARTESIAN_POINT('Ctrl Pts',(-26.8231252208352,-53.6215553879738,
-0.9));
#82125=CARTESIAN_POINT('Ctrl Pts',(-26.9460448995233,-53.9891545176506,
-0.6));
#82126=CARTESIAN_POINT('Ctrl Pts',(-26.9460448995233,-53.9891545176506,
-0.9));
#82127=CARTESIAN_POINT('',(-26.8231252208352,-53.0231921076775,-0.6));
#82128=CARTESIAN_POINT('Ctrl Pts',(-26.8231252208352,-53.0231921076775,
-0.6));
#82129=CARTESIAN_POINT('Ctrl Pts',(-26.8231252208352,-53.6215553879738,
-0.6));
#82130=CARTESIAN_POINT('Ctrl Pts',(-26.9460448995233,-53.9891545176506,
-0.6));
#82131=CARTESIAN_POINT('',(-26.8231252208352,-53.0231921076775,-0.9));
#82132=CARTESIAN_POINT('',(-26.8231252208352,-53.0231921076775,-0.6));
#82133=CARTESIAN_POINT('Ctrl Pts',(-26.8231252208352,-53.0231921076775,
-0.9));
#82134=CARTESIAN_POINT('Ctrl Pts',(-26.8231252208352,-53.6215553879738,
-0.9));
#82135=CARTESIAN_POINT('Ctrl Pts',(-26.9460448995233,-53.9891545176506,
-0.9));
#82136=CARTESIAN_POINT('Ctrl Pts',(-26.8996599689126,-52.2195772528648,
-0.6));
#82137=CARTESIAN_POINT('Ctrl Pts',(-26.8996599689126,-52.2195772528648,
-0.9));
#82138=CARTESIAN_POINT('Ctrl Pts',(-26.8231252208352,-52.5175992846489,
-0.6));
#82139=CARTESIAN_POINT('Ctrl Pts',(-26.8231252208352,-52.5175992846489,
-0.9));
#82140=CARTESIAN_POINT('Ctrl Pts',(-26.8231252208352,-53.0231921076775,
-0.6));
#82141=CARTESIAN_POINT('Ctrl Pts',(-26.8231252208352,-53.0231921076775,
-0.9));
#82142=CARTESIAN_POINT('',(-26.8996599689126,-52.2195772528648,-0.6));
#82143=CARTESIAN_POINT('Ctrl Pts',(-26.8996599689126,-52.2195772528648,
-0.6));
#82144=CARTESIAN_POINT('Ctrl Pts',(-26.8231252208352,-52.5175992846489,
-0.6));
#82145=CARTESIAN_POINT('Ctrl Pts',(-26.8231252208352,-53.0231921076775,
-0.6));
#82146=CARTESIAN_POINT('',(-26.8996599689126,-52.2195772528648,-0.9));
#82147=CARTESIAN_POINT('',(-26.8996599689126,-52.2195772528648,-0.6));
#82148=CARTESIAN_POINT('Ctrl Pts',(-26.8996599689126,-52.2195772528648,
-0.9));
#82149=CARTESIAN_POINT('Ctrl Pts',(-26.8231252208352,-52.5175992846489,
-0.9));
#82150=CARTESIAN_POINT('Ctrl Pts',(-26.8231252208352,-53.0231921076775,
-0.9));
#82151=CARTESIAN_POINT('Ctrl Pts',(-27.1107104793191,-51.7139838337898,
-0.6));
#82152=CARTESIAN_POINT('Ctrl Pts',(-27.1107104793191,-51.7139838337898,
-0.9));
#82153=CARTESIAN_POINT('Ctrl Pts',(-26.97619471699,-51.9215552210808,-0.6));
#82154=CARTESIAN_POINT('Ctrl Pts',(-26.97619471699,-51.9215552210808,-0.9));
#82155=CARTESIAN_POINT('Ctrl Pts',(-26.8996599689126,-52.2195772528648,
-0.6));
#82156=CARTESIAN_POINT('Ctrl Pts',(-26.8996599689126,-52.2195772528648,
-0.9));
#82157=CARTESIAN_POINT('',(-27.1107104793191,-51.7139838337898,-0.6));
#82158=CARTESIAN_POINT('Ctrl Pts',(-27.1107104793191,-51.7139838337898,
-0.6));
#82159=CARTESIAN_POINT('Ctrl Pts',(-26.97619471699,-51.9215552210808,-0.6));
#82160=CARTESIAN_POINT('Ctrl Pts',(-26.8996599689126,-52.2195772528648,
-0.6));
#82161=CARTESIAN_POINT('',(-27.1107104793191,-51.7139838337898,-0.9));
#82162=CARTESIAN_POINT('',(-27.1107104793191,-51.7139838337898,-0.6));
#82163=CARTESIAN_POINT('Ctrl Pts',(-27.1107104793191,-51.7139838337898,
-0.9));
#82164=CARTESIAN_POINT('Ctrl Pts',(-26.97619471699,-51.9215552210808,-0.9));
#82165=CARTESIAN_POINT('Ctrl Pts',(-26.8996599689126,-52.2195772528648,
-0.9));
#82166=CARTESIAN_POINT('Ctrl Pts',(-27.4516383185983,-51.3962487578392,
-0.6));
#82167=CARTESIAN_POINT('Ctrl Pts',(-27.4516383185983,-51.3962487578392,
-0.9));
#82168=CARTESIAN_POINT('Ctrl Pts',(-27.2452262416482,-51.5064124464989,
-0.6));
#82169=CARTESIAN_POINT('Ctrl Pts',(-27.2452262416482,-51.5064124464989,
-0.9));
#82170=CARTESIAN_POINT('Ctrl Pts',(-27.1107104793191,-51.7139838337898,
-0.6));
#82171=CARTESIAN_POINT('Ctrl Pts',(-27.1107104793191,-51.7139838337898,
-0.9));
#82172=CARTESIAN_POINT('',(-27.4516383185983,-51.3962487578392,-0.6));
#82173=CARTESIAN_POINT('Ctrl Pts',(-27.4516383185983,-51.3962487578392,
-0.6));
#82174=CARTESIAN_POINT('Ctrl Pts',(-27.2452262416482,-51.5064124464989,
-0.6));
#82175=CARTESIAN_POINT('Ctrl Pts',(-27.1107104793191,-51.7139838337898,
-0.6));
#82176=CARTESIAN_POINT('',(-27.4516383185983,-51.3962487578392,-0.9));
#82177=CARTESIAN_POINT('',(-27.4516383185983,-51.3962487578392,-0.6));
#82178=CARTESIAN_POINT('Ctrl Pts',(-27.4516383185983,-51.3962487578392,
-0.9));
#82179=CARTESIAN_POINT('Ctrl Pts',(-27.2452262416482,-51.5064124464989,
-0.9));
#82180=CARTESIAN_POINT('Ctrl Pts',(-27.1107104793191,-51.7139838337898,
-0.9));
#82181=CARTESIAN_POINT('Ctrl Pts',(-27.9317197576165,-51.2860850691795,
-0.6));
#82182=CARTESIAN_POINT('Ctrl Pts',(-27.9317197576165,-51.2860850691795,
-0.9));
#82183=CARTESIAN_POINT('Ctrl Pts',(-27.6580503955483,-51.2860850691795,
-0.6));
#82184=CARTESIAN_POINT('Ctrl Pts',(-27.6580503955483,-51.2860850691795,
-0.9));
#82185=CARTESIAN_POINT('Ctrl Pts',(-27.4516383185983,-51.3962487578392,
-0.6));
#82186=CARTESIAN_POINT('Ctrl Pts',(-27.4516383185983,-51.3962487578392,
-0.9));
#82187=CARTESIAN_POINT('',(-27.9317197576165,-51.2860850691795,-0.6));
#82188=CARTESIAN_POINT('Ctrl Pts',(-27.9317197576165,-51.2860850691795,
-0.6));
#82189=CARTESIAN_POINT('Ctrl Pts',(-27.6580503955483,-51.2860850691795,
-0.6));
#82190=CARTESIAN_POINT('Ctrl Pts',(-27.4516383185983,-51.3962487578392,
-0.6));
#82191=CARTESIAN_POINT('',(-27.9317197576165,-51.2860850691795,-0.9));
#82192=CARTESIAN_POINT('',(-27.9317197576165,-51.2860850691795,-0.6));
#82193=CARTESIAN_POINT('Ctrl Pts',(-27.9317197576165,-51.2860850691795,
-0.9));
#82194=CARTESIAN_POINT('Ctrl Pts',(-27.6580503955483,-51.2860850691795,
-0.9));
#82195=CARTESIAN_POINT('Ctrl Pts',(-27.4516383185983,-51.3962487578392,
-0.9));
#82196=CARTESIAN_POINT('Ctrl Pts',(-28.5474774613976,-51.4855388998985,
-0.6));
#82197=CARTESIAN_POINT('Ctrl Pts',(-28.5474774613976,-51.4855388998985,
-0.9));
#82198=CARTESIAN_POINT('Ctrl Pts',(-28.3027980104089,-51.2860850691795,
-0.6));
#82199=CARTESIAN_POINT('Ctrl Pts',(-28.3027980104089,-51.2860850691795,
-0.9));
#82200=CARTESIAN_POINT('Ctrl Pts',(-27.9317197576165,-51.2860850691795,
-0.6));
#82201=CARTESIAN_POINT('Ctrl Pts',(-27.9317197576165,-51.2860850691795,
-0.9));
#82202=CARTESIAN_POINT('',(-28.5474774613976,-51.4855388998985,-0.6));
#82203=CARTESIAN_POINT('Ctrl Pts',(-28.5474774613976,-51.4855388998985,
-0.6));
#82204=CARTESIAN_POINT('Ctrl Pts',(-28.3027980104089,-51.2860850691795,
-0.6));
#82205=CARTESIAN_POINT('Ctrl Pts',(-27.9317197576165,-51.2860850691795,
-0.6));
#82206=CARTESIAN_POINT('',(-28.5474774613976,-51.4855388998985,-0.9));
#82207=CARTESIAN_POINT('',(-28.5474774613976,-51.4855388998985,-0.6));
#82208=CARTESIAN_POINT('Ctrl Pts',(-28.5474774613976,-51.4855388998985,
-0.9));
#82209=CARTESIAN_POINT('Ctrl Pts',(-28.3027980104089,-51.2860850691795,
-0.9));
#82210=CARTESIAN_POINT('Ctrl Pts',(-27.9317197576165,-51.2860850691795,
-0.9));
#82211=CARTESIAN_POINT('Ctrl Pts',(-28.9162359014153,-52.0525924563408,
-0.6));
#82212=CARTESIAN_POINT('Ctrl Pts',(-28.9162359014153,-52.0525924563408,
-0.9));
#82213=CARTESIAN_POINT('Ctrl Pts',(-28.7921569123864,-51.684993326664,-0.6));
#82214=CARTESIAN_POINT('Ctrl Pts',(-28.7921569123864,-51.684993326664,-0.9));
#82215=CARTESIAN_POINT('Ctrl Pts',(-28.5474774613976,-51.4855388998985,
-0.6));
#82216=CARTESIAN_POINT('Ctrl Pts',(-28.5474774613976,-51.4855388998985,
-0.9));
#82217=CARTESIAN_POINT('',(-28.9162359014153,-52.0525924563408,-0.6));
#82218=CARTESIAN_POINT('Ctrl Pts',(-28.9162359014153,-52.0525924563408,
-0.6));
#82219=CARTESIAN_POINT('Ctrl Pts',(-28.7921569123864,-51.684993326664,-0.6));
#82220=CARTESIAN_POINT('Ctrl Pts',(-28.5474774613976,-51.4855388998985,
-0.6));
#82221=CARTESIAN_POINT('',(-28.9162359014153,-52.0525924563408,-0.9));
#82222=CARTESIAN_POINT('',(-28.9162359014153,-52.0525924563408,-0.6));
#82223=CARTESIAN_POINT('Ctrl Pts',(-28.9162359014153,-52.0525924563408,
-0.9));
#82224=CARTESIAN_POINT('Ctrl Pts',(-28.7921569123864,-51.684993326664,-0.9));
#82225=CARTESIAN_POINT('Ctrl Pts',(-28.5474774613976,-51.4855388998985,
-0.9));
#82226=CARTESIAN_POINT('Ctrl Pts',(-29.0403148904443,-53.0231921076775,
-0.6));
#82227=CARTESIAN_POINT('Ctrl Pts',(-29.0403148904443,-53.0231921076775,
-0.9));
#82228=CARTESIAN_POINT('Ctrl Pts',(-29.0403148904443,-52.4201909899712,
-0.6));
#82229=CARTESIAN_POINT('Ctrl Pts',(-29.0403148904443,-52.4201909899712,
-0.9));
#82230=CARTESIAN_POINT('Ctrl Pts',(-28.9162359014153,-52.0525924563408,
-0.6));
#82231=CARTESIAN_POINT('Ctrl Pts',(-28.9162359014153,-52.0525924563408,
-0.9));
#82232=CARTESIAN_POINT('',(-29.0403148904443,-53.0231921076775,-0.6));
#82233=CARTESIAN_POINT('Ctrl Pts',(-29.0403148904443,-53.0231921076775,
-0.6));
#82234=CARTESIAN_POINT('Ctrl Pts',(-29.0403148904443,-52.4201909899712,
-0.6));
#82235=CARTESIAN_POINT('Ctrl Pts',(-28.9162359014153,-52.0525924563408,
-0.6));
#82236=CARTESIAN_POINT('',(-29.0403148904443,-53.0231921076775,-0.9));
#82237=CARTESIAN_POINT('',(-29.0403148904443,-53.0231921076775,-0.6));
#82238=CARTESIAN_POINT('Ctrl Pts',(-29.0403148904443,-53.0231921076775,
-0.9));
#82239=CARTESIAN_POINT('Ctrl Pts',(-29.0403148904443,-52.4201909899712,
-0.9));
#82240=CARTESIAN_POINT('Ctrl Pts',(-28.9162359014153,-52.0525924563408,
-0.9));
#82241=CARTESIAN_POINT('Ctrl Pts',(-28.7040254846215,-54.4054571986198,
-0.6));
#82242=CARTESIAN_POINT('Ctrl Pts',(-28.7040254846215,-54.4054571986198,
-0.9));
#82243=CARTESIAN_POINT('Ctrl Pts',(-29.0403148904443,-53.9810369610786,
-0.6));
#82244=CARTESIAN_POINT('Ctrl Pts',(-29.0403148904443,-53.9810369610786,
-0.9));
#82245=CARTESIAN_POINT('Ctrl Pts',(-29.0403148904443,-53.0231921076775,
-0.6));
#82246=CARTESIAN_POINT('Ctrl Pts',(-29.0403148904443,-53.0231921076775,
-0.9));
#82247=CARTESIAN_POINT('',(-28.7040254846215,-54.4054571986198,-0.6));
#82248=CARTESIAN_POINT('Ctrl Pts',(-28.7040254846215,-54.4054571986198,
-0.6));
#82249=CARTESIAN_POINT('Ctrl Pts',(-29.0403148904443,-53.9810369610786,
-0.6));
#82250=CARTESIAN_POINT('Ctrl Pts',(-29.0403148904443,-53.0231921076775,
-0.6));
#82251=CARTESIAN_POINT('',(-28.7040254846215,-54.4054571986198,-0.9));
#82252=CARTESIAN_POINT('',(-28.7040254846215,-54.4054571986198,-0.6));
#82253=CARTESIAN_POINT('Ctrl Pts',(-28.7040254846215,-54.4054571986198,
-0.9));
#82254=CARTESIAN_POINT('Ctrl Pts',(-29.0403148904443,-53.9810369610786,
-0.9));
#82255=CARTESIAN_POINT('Ctrl Pts',(-29.0403148904443,-53.0231921076775,
-0.9));
#82256=CARTESIAN_POINT('Ctrl Pts',(-27.9317197576165,-54.7579811215401,
-0.6));
#82257=CARTESIAN_POINT('Ctrl Pts',(-27.9317197576165,-54.7579811215401,
-0.9));
#82258=CARTESIAN_POINT('Ctrl Pts',(-28.4233978763223,-54.7579811215401,
-0.6));
#82259=CARTESIAN_POINT('Ctrl Pts',(-28.4233978763223,-54.7579811215401,
-0.9));
#82260=CARTESIAN_POINT('Ctrl Pts',(-28.7040254846215,-54.4054571986198,
-0.6));
#82261=CARTESIAN_POINT('Ctrl Pts',(-28.7040254846215,-54.4054571986198,
-0.9));
#82262=CARTESIAN_POINT('Ctrl Pts',(-27.9317197576165,-54.7579811215401,
-0.6));
#82263=CARTESIAN_POINT('Ctrl Pts',(-28.4233978763223,-54.7579811215401,
-0.6));
#82264=CARTESIAN_POINT('Ctrl Pts',(-28.7040254846215,-54.4054571986198,
-0.6));
#82265=CARTESIAN_POINT('Ctrl Pts',(-27.9317197576165,-54.7579811215401,
-0.9));
#82266=CARTESIAN_POINT('Ctrl Pts',(-28.4233978763223,-54.7579811215401,
-0.9));
#82267=CARTESIAN_POINT('Ctrl Pts',(-28.7040254846215,-54.4054571986198,
-0.9));
#82268=CARTESIAN_POINT('Origin',(-27.9317200556397,-53.0220330953598,-0.9));
#82269=CARTESIAN_POINT('Ctrl Pts',(-30.7495922222733,-51.7406551241875,
-0.6));
#82270=CARTESIAN_POINT('Ctrl Pts',(-30.7495922222733,-51.7406551241875,
-0.9));
#82271=CARTESIAN_POINT('Ctrl Pts',(-30.487518645823,-51.5064118504524,-0.6));
#82272=CARTESIAN_POINT('Ctrl Pts',(-30.487518645823,-51.5064118504524,-0.9));
#82273=CARTESIAN_POINT('Ctrl Pts',(-30.3785142675042,-51.2860844731331,
-0.6));
#82274=CARTESIAN_POINT('Ctrl Pts',(-30.3785142675042,-51.2860844731331,
-0.9));
#82275=CARTESIAN_POINT('',(-30.7495922222733,-51.7406551241875,-0.6));
#82276=CARTESIAN_POINT('',(-30.3785142675042,-51.2860844731331,-0.6));
#82277=CARTESIAN_POINT('Ctrl Pts',(-30.7495922222733,-51.7406551241875,
-0.6));
#82278=CARTESIAN_POINT('Ctrl Pts',(-30.487518645823,-51.5064118504524,-0.6));
#82279=CARTESIAN_POINT('Ctrl Pts',(-30.3785142675042,-51.2860844731331,
-0.6));
#82280=CARTESIAN_POINT('',(-30.7495922222733,-51.7406551241875,-0.9));
#82281=CARTESIAN_POINT('',(-30.7495922222733,-51.7406551241875,-0.6));
#82282=CARTESIAN_POINT('',(-30.3785142675042,-51.2860844731331,-0.9));
#82283=CARTESIAN_POINT('Ctrl Pts',(-30.7495922222733,-51.7406551241875,
-0.9));
#82284=CARTESIAN_POINT('Ctrl Pts',(-30.487518645823,-51.5064118504524,-0.9));
#82285=CARTESIAN_POINT('Ctrl Pts',(-30.3785142675042,-51.2860844731331,
-0.9));
#82286=CARTESIAN_POINT('',(-30.3785142675042,-51.2860844731331,-0.6));
#82287=CARTESIAN_POINT('Ctrl Pts',(-31.3618705049157,-52.1395633816719,
-0.6));
#82288=CARTESIAN_POINT('Ctrl Pts',(-31.3618705049157,-52.1395633816719,
-0.9));
#82289=CARTESIAN_POINT('Ctrl Pts',(-31.0116657987237,-51.9748978018761,
-0.6));
#82290=CARTESIAN_POINT('Ctrl Pts',(-31.0116657987237,-51.9748978018761,
-0.9));
#82291=CARTESIAN_POINT('Ctrl Pts',(-30.7495922222733,-51.7406551241875,
-0.6));
#82292=CARTESIAN_POINT('Ctrl Pts',(-30.7495922222733,-51.7406551241875,
-0.9));
#82293=CARTESIAN_POINT('',(-31.3618705049157,-52.1395633816719,-0.6));
#82294=CARTESIAN_POINT('Ctrl Pts',(-31.3618705049157,-52.1395633816719,
-0.6));
#82295=CARTESIAN_POINT('Ctrl Pts',(-31.0116657987237,-51.9748978018761,
-0.6));
#82296=CARTESIAN_POINT('Ctrl Pts',(-30.7495922222733,-51.7406551241875,
-0.6));
#82297=CARTESIAN_POINT('',(-31.3618705049157,-52.1395633816719,-0.9));
#82298=CARTESIAN_POINT('',(-31.3618705049157,-52.1395633816719,-0.6));
#82299=CARTESIAN_POINT('Ctrl Pts',(-31.3618705049157,-52.1395633816719,
-0.9));
#82300=CARTESIAN_POINT('Ctrl Pts',(-31.0116657987237,-51.9748978018761,
-0.9));
#82301=CARTESIAN_POINT('Ctrl Pts',(-30.7495922222733,-51.7406551241875,
-0.9));
#82302=CARTESIAN_POINT('Origin',(-31.3618705049157,-52.5431100726128,-0.6));
#82303=CARTESIAN_POINT('',(-31.3618705049157,-52.5431100726128,-0.6));
#82304=CARTESIAN_POINT('',(-31.3618705049157,-52.7715550363064,-0.6));
#82305=CARTESIAN_POINT('',(-31.3618705049157,-52.5431100726128,-0.9));
#82306=CARTESIAN_POINT('',(-31.3618705049157,-52.5431100726128,-0.6));
#82307=CARTESIAN_POINT('',(-31.3618705049157,-52.5431100726128,-0.9));
#82308=CARTESIAN_POINT('Ctrl Pts',(-30.9223753586411,-52.3274211287498,
-0.6));
#82309=CARTESIAN_POINT('Ctrl Pts',(-30.9223753586411,-52.3274211287498,
-0.9));
#82310=CARTESIAN_POINT('Ctrl Pts',(-31.1670548096299,-52.4712137579918,
-0.6));
#82311=CARTESIAN_POINT('Ctrl Pts',(-31.1670548096299,-52.4712137579918,
-0.9));
#82312=CARTESIAN_POINT('Ctrl Pts',(-31.3618705049157,-52.5431100726128,
-0.6));
#82313=CARTESIAN_POINT('Ctrl Pts',(-31.3618705049157,-52.5431100726128,
-0.9));
#82314=CARTESIAN_POINT('',(-30.9223753586411,-52.3274211287498,-0.6));
#82315=CARTESIAN_POINT('Ctrl Pts',(-30.9223753586411,-52.3274211287498,
-0.6));
#82316=CARTESIAN_POINT('Ctrl Pts',(-31.1670548096299,-52.4712137579918,
-0.6));
#82317=CARTESIAN_POINT('Ctrl Pts',(-31.3618705049157,-52.5431100726128,
-0.6));
#82318=CARTESIAN_POINT('',(-30.9223753586411,-52.3274211287498,-0.9));
#82319=CARTESIAN_POINT('',(-30.9223753586411,-52.3274211287498,-0.6));
#82320=CARTESIAN_POINT('Ctrl Pts',(-30.9223753586411,-52.3274211287498,
-0.9));
#82321=CARTESIAN_POINT('Ctrl Pts',(-31.1670548096299,-52.4712137579918,
-0.9));
#82322=CARTESIAN_POINT('Ctrl Pts',(-31.3618705049157,-52.5431100726128,
-0.9));
#82323=CARTESIAN_POINT('Ctrl Pts',(-30.5269453302026,-52.039835870266,-0.6));
#82324=CARTESIAN_POINT('Ctrl Pts',(-30.5269453302026,-52.039835870266,-0.9));
#82325=CARTESIAN_POINT('Ctrl Pts',(-30.6776959076524,-52.1836284995079,
-0.6));
#82326=CARTESIAN_POINT('Ctrl Pts',(-30.6776959076524,-52.1836284995079,
-0.9));
#82327=CARTESIAN_POINT('Ctrl Pts',(-30.9223753586411,-52.3274211287498,
-0.6));
#82328=CARTESIAN_POINT('Ctrl Pts',(-30.9223753586411,-52.3274211287498,
-0.9));
#82329=CARTESIAN_POINT('',(-30.5269453302026,-52.039835870266,-0.6));
#82330=CARTESIAN_POINT('Ctrl Pts',(-30.5269453302026,-52.039835870266,-0.6));
#82331=CARTESIAN_POINT('Ctrl Pts',(-30.6776959076524,-52.1836284995079,
-0.6));
#82332=CARTESIAN_POINT('Ctrl Pts',(-30.9223753586411,-52.3274211287498,
-0.6));
#82333=CARTESIAN_POINT('',(-30.5269453302026,-52.039835870266,-0.9));
#82334=CARTESIAN_POINT('',(-30.5269453302026,-52.039835870266,-0.6));
#82335=CARTESIAN_POINT('Ctrl Pts',(-30.5269453302026,-52.039835870266,-0.9));
#82336=CARTESIAN_POINT('Ctrl Pts',(-30.6776959076524,-52.1836284995079,
-0.9));
#82337=CARTESIAN_POINT('Ctrl Pts',(-30.9223753586411,-52.3274211287498,
-0.9));
#82338=CARTESIAN_POINT('Origin',(-30.5269453302026,-54.7000001072884,-0.6));
#82339=CARTESIAN_POINT('',(-30.5269453302026,-54.7000001072884,-0.6));
#82340=CARTESIAN_POINT('',(-30.5269453302026,-53.8500000536442,-0.6));
#82341=CARTESIAN_POINT('',(-30.5269453302026,-54.7000001072884,-0.9));
#82342=CARTESIAN_POINT('',(-30.5269453302026,-54.7000001072884,-0.6));
#82343=CARTESIAN_POINT('',(-30.5269453302026,-54.7000001072884,-0.9));
#82344=CARTESIAN_POINT('Origin',(-30.109482742846,-54.7000001072884,-0.6));
#82345=CARTESIAN_POINT('',(-30.109482742846,-54.7000001072884,-0.6));
#82346=CARTESIAN_POINT('',(-15.054741371423,-54.7000001072884,-0.6));
#82347=CARTESIAN_POINT('',(-30.109482742846,-54.7000001072884,-0.9));
#82348=CARTESIAN_POINT('',(-30.109482742846,-54.7000001072884,-0.6));
#82349=CARTESIAN_POINT('',(-30.109482742846,-54.7000001072884,-0.9));
#82350=CARTESIAN_POINT('Origin',(-30.109482742846,-51.2860844731331,-0.6));
#82351=CARTESIAN_POINT('',(-30.109482742846,-51.2860844731331,-0.6));
#82352=CARTESIAN_POINT('',(-30.109482742846,-52.1430422365665,-0.6));
#82353=CARTESIAN_POINT('',(-30.109482742846,-51.2860844731331,-0.9));
#82354=CARTESIAN_POINT('',(-30.109482742846,-51.2860844731331,-0.6));
#82355=CARTESIAN_POINT('',(-30.109482742846,-51.2860844731331,-0.9));
#82356=CARTESIAN_POINT('Origin',(-30.3785142675042,-51.2860844731331,-0.6));
#82357=CARTESIAN_POINT('',(-15.1892571337521,-51.2860844731331,-0.6));
#82358=CARTESIAN_POINT('',(-30.3785142675042,-51.2860844731331,-0.9));
#82359=CARTESIAN_POINT('Origin',(-30.7356766238809,-52.9930422902107,-0.9));
#82360=CARTESIAN_POINT('Origin',(-26.4450899139047,-53.2597545981407,-0.6));
#82361=CARTESIAN_POINT('',(-26.4450899139047,-53.2597545981407,-0.6));
#82362=CARTESIAN_POINT('',(-25.1625523343682,-53.2597545981407,-0.6));
#82363=CARTESIAN_POINT('',(-13.2225449569523,-53.2597545981407,-0.6));
#82364=CARTESIAN_POINT('',(-26.4450899139047,-53.2597545981407,-0.9));
#82365=CARTESIAN_POINT('',(-26.4450899139047,-53.2597545981407,-0.6));
#82366=CARTESIAN_POINT('',(-25.1625523343682,-53.2597545981407,-0.9));
#82367=CARTESIAN_POINT('',(-26.4450899139047,-53.2597545981407,-0.9));
#82368=CARTESIAN_POINT('',(-25.1625523343682,-53.2597545981407,-0.6));
#82369=CARTESIAN_POINT('Origin',(-26.4450899139047,-53.6795364022255,-0.6));
#82370=CARTESIAN_POINT('',(-26.4450899139047,-53.6795364022255,-0.6));
#82371=CARTESIAN_POINT('',(-26.4450899139047,-53.3397682011127,-0.6));
#82372=CARTESIAN_POINT('',(-26.4450899139047,-53.6795364022255,-0.9));
#82373=CARTESIAN_POINT('',(-26.4450899139047,-53.6795364022255,-0.6));
#82374=CARTESIAN_POINT('',(-26.4450899139047,-53.6795364022255,-0.9));
#82375=CARTESIAN_POINT('Origin',(-25.1625523343682,-53.6795364022255,-0.6));
#82376=CARTESIAN_POINT('',(-25.1625523343682,-53.6795364022255,-0.6));
#82377=CARTESIAN_POINT('',(-12.5812761671841,-53.6795364022255,-0.6));
#82378=CARTESIAN_POINT('',(-25.1625523343682,-53.6795364022255,-0.9));
#82379=CARTESIAN_POINT('',(-25.1625523343682,-53.6795364022255,-0.6));
#82380=CARTESIAN_POINT('',(-25.1625523343682,-53.6795364022255,-0.9));
#82381=CARTESIAN_POINT('Origin',(-25.1625523343682,-53.2597545981407,-0.6));
#82382=CARTESIAN_POINT('',(-25.1625523343682,-53.1298772990704,-0.6));
#82383=CARTESIAN_POINT('',(-25.1625523343682,-53.2597545981407,-0.9));
#82384=CARTESIAN_POINT('Origin',(-25.8038211241364,-53.4696455001831,-0.9));
#82385=CARTESIAN_POINT('Ctrl Pts',(-20.1901099458337,-54.3451569676399,
-0.6));
#82386=CARTESIAN_POINT('Ctrl Pts',(-20.1901099458337,-54.3451569676399,
-0.9));
#82387=CARTESIAN_POINT('Ctrl Pts',(-20.5171224847436,-54.7579811215401,
-0.6));
#82388=CARTESIAN_POINT('Ctrl Pts',(-20.5171224847436,-54.7579811215401,
-0.9));
#82389=CARTESIAN_POINT('Ctrl Pts',(-21.0830161347985,-54.7579811215401,
-0.6));
#82390=CARTESIAN_POINT('Ctrl Pts',(-21.0830161347985,-54.7579811215401,
-0.9));
#82391=CARTESIAN_POINT('',(-20.1901099458337,-54.3451569676399,-0.6));
#82392=CARTESIAN_POINT('',(-21.0830161347985,-54.7579811215401,-0.6));
#82393=CARTESIAN_POINT('Ctrl Pts',(-20.1901099458337,-54.3451569676399,
-0.6));
#82394=CARTESIAN_POINT('Ctrl Pts',(-20.5171224847436,-54.7579811215401,
-0.6));
#82395=CARTESIAN_POINT('Ctrl Pts',(-21.0830161347985,-54.7579811215401,
-0.6));
#82396=CARTESIAN_POINT('',(-20.1901099458337,-54.3451569676399,-0.9));
#82397=CARTESIAN_POINT('',(-20.1901099458337,-54.3451569676399,-0.6));
#82398=CARTESIAN_POINT('',(-21.0830161347985,-54.7579811215401,-0.9));
#82399=CARTESIAN_POINT('Ctrl Pts',(-20.1901099458337,-54.3451569676399,
-0.9));
#82400=CARTESIAN_POINT('Ctrl Pts',(-20.5171224847436,-54.7579811215401,
-0.9));
#82401=CARTESIAN_POINT('Ctrl Pts',(-21.0830161347985,-54.7579811215401,
-0.9));
#82402=CARTESIAN_POINT('',(-21.0830161347985,-54.7579811215401,-0.6));
#82403=CARTESIAN_POINT('Ctrl Pts',(-19.9210784211755,-53.5473398566246,
-0.6));
#82404=CARTESIAN_POINT('Ctrl Pts',(-19.9210784211755,-53.5473398566246,
-0.9));
#82405=CARTESIAN_POINT('Ctrl Pts',(-19.9210784211755,-54.0088675618172,
-0.6));
#82406=CARTESIAN_POINT('Ctrl Pts',(-19.9210784211755,-54.0088675618172,
-0.9));
#82407=CARTESIAN_POINT('Ctrl Pts',(-20.1901099458337,-54.3451569676399,
-0.6));
#82408=CARTESIAN_POINT('Ctrl Pts',(-20.1901099458337,-54.3451569676399,
-0.9));
#82409=CARTESIAN_POINT('',(-19.9210784211755,-53.5473398566246,-0.6));
#82410=CARTESIAN_POINT('Ctrl Pts',(-19.9210784211755,-53.5473398566246,
-0.6));
#82411=CARTESIAN_POINT('Ctrl Pts',(-19.9210784211755,-54.0088675618172,
-0.6));
#82412=CARTESIAN_POINT('Ctrl Pts',(-20.1901099458337,-54.3451569676399,
-0.6));
#82413=CARTESIAN_POINT('',(-19.9210784211755,-53.5473398566246,-0.9));
#82414=CARTESIAN_POINT('',(-19.9210784211755,-53.5473398566246,-0.6));
#82415=CARTESIAN_POINT('Ctrl Pts',(-19.9210784211755,-53.5473398566246,
-0.9));
#82416=CARTESIAN_POINT('Ctrl Pts',(-19.9210784211755,-54.0088675618172,
-0.9));
#82417=CARTESIAN_POINT('Ctrl Pts',(-20.1901099458337,-54.3451569676399,
-0.9));
#82418=CARTESIAN_POINT('Ctrl Pts',(-20.2272174134851,-52.7541605830193,
-0.6));
#82419=CARTESIAN_POINT('Ctrl Pts',(-20.2272174134851,-52.7541605830193,
-0.9));
#82420=CARTESIAN_POINT('Ctrl Pts',(-19.9210784211755,-53.0626193881035,
-0.6));
#82421=CARTESIAN_POINT('Ctrl Pts',(-19.9210784211755,-53.0626193881035,
-0.9));
#82422=CARTESIAN_POINT('Ctrl Pts',(-19.9210784211755,-53.5473398566246,
-0.6));
#82423=CARTESIAN_POINT('Ctrl Pts',(-19.9210784211755,-53.5473398566246,
-0.9));
#82424=CARTESIAN_POINT('',(-20.2272174134851,-52.7541605830193,-0.6));
#82425=CARTESIAN_POINT('Ctrl Pts',(-20.2272174134851,-52.7541605830193,
-0.6));
#82426=CARTESIAN_POINT('Ctrl Pts',(-19.9210784211755,-53.0626193881035,
-0.6));
#82427=CARTESIAN_POINT('Ctrl Pts',(-19.9210784211755,-53.5473398566246,
-0.6));
#82428=CARTESIAN_POINT('',(-20.2272174134851,-52.7541605830193,-0.9));
#82429=CARTESIAN_POINT('',(-20.2272174134851,-52.7541605830193,-0.6));
#82430=CARTESIAN_POINT('Ctrl Pts',(-20.2272174134851,-52.7541605830193,
-0.9));
#82431=CARTESIAN_POINT('Ctrl Pts',(-19.9210784211755,-53.0626193881035,
-0.9));
#82432=CARTESIAN_POINT('Ctrl Pts',(-19.9210784211755,-53.5473398566246,
-0.9));
#82433=CARTESIAN_POINT('Ctrl Pts',(-20.9786507859826,-52.4457023739815,
-0.6));
#82434=CARTESIAN_POINT('Ctrl Pts',(-20.9786507859826,-52.4457023739815,
-0.9));
#82435=CARTESIAN_POINT('Ctrl Pts',(-20.5333575978875,-52.4457023739815,
-0.6));
#82436=CARTESIAN_POINT('Ctrl Pts',(-20.5333575978875,-52.4457023739815,
-0.9));
#82437=CARTESIAN_POINT('Ctrl Pts',(-20.2272174134851,-52.7541605830193,
-0.6));
#82438=CARTESIAN_POINT('Ctrl Pts',(-20.2272174134851,-52.7541605830193,
-0.9));
#82439=CARTESIAN_POINT('',(-20.9786507859826,-52.4457023739815,-0.6));
#82440=CARTESIAN_POINT('Ctrl Pts',(-20.9786507859826,-52.4457023739815,
-0.6));
#82441=CARTESIAN_POINT('Ctrl Pts',(-20.5333575978875,-52.4457023739815,
-0.6));
#82442=CARTESIAN_POINT('Ctrl Pts',(-20.2272174134851,-52.7541605830193,
-0.6));
#82443=CARTESIAN_POINT('',(-20.9786507859826,-52.4457023739815,-0.9));
#82444=CARTESIAN_POINT('',(-20.9786507859826,-52.4457023739815,-0.6));
#82445=CARTESIAN_POINT('Ctrl Pts',(-20.9786507859826,-52.4457023739815,
-0.9));
#82446=CARTESIAN_POINT('Ctrl Pts',(-20.5333575978875,-52.4457023739815,
-0.9));
#82447=CARTESIAN_POINT('Ctrl Pts',(-20.2272174134851,-52.7541605830193,
-0.9));
#82448=CARTESIAN_POINT('Ctrl Pts',(-21.6210791841149,-52.6590721011162,
-0.6));
#82449=CARTESIAN_POINT('Ctrl Pts',(-21.6210791841149,-52.6590721011162,
-0.9));
#82450=CARTESIAN_POINT('Ctrl Pts',(-21.3149389997125,-52.4457023739815,
-0.6));
#82451=CARTESIAN_POINT('Ctrl Pts',(-21.3149389997125,-52.4457023739815,
-0.9));
#82452=CARTESIAN_POINT('Ctrl Pts',(-20.9786507859826,-52.4457023739815,
-0.6));
#82453=CARTESIAN_POINT('Ctrl Pts',(-20.9786507859826,-52.4457023739815,
-0.9));
#82454=CARTESIAN_POINT('',(-21.6210791841149,-52.6590721011162,-0.6));
#82455=CARTESIAN_POINT('Ctrl Pts',(-21.6210791841149,-52.6590721011162,
-0.6));
#82456=CARTESIAN_POINT('Ctrl Pts',(-21.3149389997125,-52.4457023739815,
-0.6));
#82457=CARTESIAN_POINT('Ctrl Pts',(-20.9786507859826,-52.4457023739815,
-0.6));
#82458=CARTESIAN_POINT('',(-21.6210791841149,-52.6590721011162,-0.9));
#82459=CARTESIAN_POINT('',(-21.6210791841149,-52.6590721011162,-0.6));
#82460=CARTESIAN_POINT('Ctrl Pts',(-21.6210791841149,-52.6590721011162,
-0.9));
#82461=CARTESIAN_POINT('Ctrl Pts',(-21.3149389997125,-52.4457023739815,
-0.9));
#82462=CARTESIAN_POINT('Ctrl Pts',(-20.9786507859826,-52.4457023739815,
-0.9));
#82463=CARTESIAN_POINT('Origin',(-21.437859274447,-51.7452935576439,-0.6));
#82464=CARTESIAN_POINT('',(-21.437859274447,-51.7452935576439,-0.6));
#82465=CARTESIAN_POINT('',(-21.1445044486643,-50.2822356077188,-0.6));
#82466=CARTESIAN_POINT('',(-21.437859274447,-51.7452935576439,-0.9));
#82467=CARTESIAN_POINT('',(-21.437859274447,-51.7452935576439,-0.6));
#82468=CARTESIAN_POINT('',(-21.437859274447,-51.7452935576439,-0.9));
#82469=CARTESIAN_POINT('Origin',(-20.0811061635613,-51.7452935576439,-0.6));
#82470=CARTESIAN_POINT('',(-20.0811061635613,-51.7452935576439,-0.6));
#82471=CARTESIAN_POINT('',(-10.0405530817807,-51.7452935576439,-0.6));
#82472=CARTESIAN_POINT('',(-20.0811061635613,-51.7452935576439,-0.9));
#82473=CARTESIAN_POINT('',(-20.0811061635613,-51.7452935576439,-0.6));
#82474=CARTESIAN_POINT('',(-20.0811061635613,-51.7452935576439,-0.9));
#82475=CARTESIAN_POINT('Origin',(-20.0811061635613,-51.346384704113,-0.6));
#82476=CARTESIAN_POINT('',(-20.0811061635613,-51.346384704113,-0.6));
#82477=CARTESIAN_POINT('',(-20.0811061635613,-52.1731923520565,-0.6));
#82478=CARTESIAN_POINT('',(-20.0811061635613,-51.346384704113,-0.9));
#82479=CARTESIAN_POINT('',(-20.0811061635613,-51.346384704113,-0.6));
#82480=CARTESIAN_POINT('',(-20.0811061635613,-51.346384704113,-0.9));
#82481=CARTESIAN_POINT('Origin',(-21.7718288674951,-51.346384704113,-0.6));
#82482=CARTESIAN_POINT('',(-21.7718288674951,-51.346384704113,-0.6));
#82483=CARTESIAN_POINT('',(-10.8859144337475,-51.346384704113,-0.6));
#82484=CARTESIAN_POINT('',(-21.7718288674951,-51.346384704113,-0.9));
#82485=CARTESIAN_POINT('',(-21.7718288674951,-51.346384704113,-0.6));
#82486=CARTESIAN_POINT('',(-21.7718288674951,-51.346384704113,-0.9));
#82487=CARTESIAN_POINT('Origin',(-22.1011600270867,-53.0927692055702,-0.6));
#82488=CARTESIAN_POINT('',(-22.1011600270867,-53.0927692055702,-0.6));
#82489=CARTESIAN_POINT('',(-21.7132280182382,-51.0356348344644,-0.6));
#82490=CARTESIAN_POINT('',(-22.1011600270867,-53.0927692055702,-0.9));
#82491=CARTESIAN_POINT('',(-22.1011600270867,-53.0927692055702,-0.6));
#82492=CARTESIAN_POINT('',(-22.1011600270867,-53.0927692055702,-0.9));
#82493=CARTESIAN_POINT('Origin',(-21.7092094197869,-53.1437925696373,-0.6));
#82494=CARTESIAN_POINT('',(-21.7092094197869,-53.1437925696373,-0.6));
#82495=CARTESIAN_POINT('',(-11.0446884509171,-54.5320790676332,-0.6));
#82496=CARTESIAN_POINT('',(-21.7092094197869,-53.1437925696373,-0.9));
#82497=CARTESIAN_POINT('',(-21.7092094197869,-53.1437925696373,-0.6));
#82498=CARTESIAN_POINT('',(-21.7092094197869,-53.1437925696373,-0.9));
#82499=CARTESIAN_POINT('Ctrl Pts',(-21.454093195498,-52.9060707688332,-0.6));
#82500=CARTESIAN_POINT('Ctrl Pts',(-21.454093195498,-52.9060707688332,-0.9));
#82501=CARTESIAN_POINT('Ctrl Pts',(-21.6164407506585,-52.9976807236671,
-0.6));
#82502=CARTESIAN_POINT('Ctrl Pts',(-21.6164407506585,-52.9976807236671,
-0.9));
#82503=CARTESIAN_POINT('Ctrl Pts',(-21.7092094197869,-53.1437925696373,
-0.6));
#82504=CARTESIAN_POINT('Ctrl Pts',(-21.7092094197869,-53.1437925696373,
-0.9));
#82505=CARTESIAN_POINT('',(-21.454093195498,-52.9060707688332,-0.6));
#82506=CARTESIAN_POINT('Ctrl Pts',(-21.454093195498,-52.9060707688332,-0.6));
#82507=CARTESIAN_POINT('Ctrl Pts',(-21.6164407506585,-52.9976807236671,
-0.6));
#82508=CARTESIAN_POINT('Ctrl Pts',(-21.7092094197869,-53.1437925696373,
-0.6));
#82509=CARTESIAN_POINT('',(-21.454093195498,-52.9060707688332,-0.9));
#82510=CARTESIAN_POINT('',(-21.454093195498,-52.9060707688332,-0.6));
#82511=CARTESIAN_POINT('Ctrl Pts',(-21.454093195498,-52.9060707688332,-0.9));
#82512=CARTESIAN_POINT('Ctrl Pts',(-21.6164407506585,-52.9976807236671,
-0.9));
#82513=CARTESIAN_POINT('Ctrl Pts',(-21.7092094197869,-53.1437925696373,
-0.9));
#82514=CARTESIAN_POINT('Ctrl Pts',(-21.0899731889367,-52.8144608139992,
-0.6));
#82515=CARTESIAN_POINT('Ctrl Pts',(-21.0899731889367,-52.8144608139992,
-0.9));
#82516=CARTESIAN_POINT('Ctrl Pts',(-21.2917468324304,-52.8144608139992,
-0.6));
#82517=CARTESIAN_POINT('Ctrl Pts',(-21.2917468324304,-52.8144608139992,
-0.9));
#82518=CARTESIAN_POINT('Ctrl Pts',(-21.454093195498,-52.9060707688332,-0.6));
#82519=CARTESIAN_POINT('Ctrl Pts',(-21.454093195498,-52.9060707688332,-0.9));
#82520=CARTESIAN_POINT('',(-21.0899731889367,-52.8144608139992,-0.6));
#82521=CARTESIAN_POINT('Ctrl Pts',(-21.0899731889367,-52.8144608139992,
-0.6));
#82522=CARTESIAN_POINT('Ctrl Pts',(-21.2917468324304,-52.8144608139992,
-0.6));
#82523=CARTESIAN_POINT('Ctrl Pts',(-21.454093195498,-52.9060707688332,-0.6));
#82524=CARTESIAN_POINT('',(-21.0899731889367,-52.8144608139992,-0.9));
#82525=CARTESIAN_POINT('',(-21.0899731889367,-52.8144608139992,-0.6));
#82526=CARTESIAN_POINT('Ctrl Pts',(-21.0899731889367,-52.8144608139992,
-0.9));
#82527=CARTESIAN_POINT('Ctrl Pts',(-21.2917468324304,-52.8144608139992,
-0.9));
#82528=CARTESIAN_POINT('Ctrl Pts',(-21.454093195498,-52.9060707688332,-0.9));
#82529=CARTESIAN_POINT('Ctrl Pts',(-20.5646667256951,-53.0208728909492,
-0.6));
#82530=CARTESIAN_POINT('Ctrl Pts',(-20.5646667256951,-53.0208728909492,
-0.9));
#82531=CARTESIAN_POINT('Ctrl Pts',(-20.7652804628015,-52.8144608139992,
-0.6));
#82532=CARTESIAN_POINT('Ctrl Pts',(-20.7652804628015,-52.8144608139992,
-0.9));
#82533=CARTESIAN_POINT('Ctrl Pts',(-21.0899731889367,-52.8144608139992,
-0.6));
#82534=CARTESIAN_POINT('Ctrl Pts',(-21.0899731889367,-52.8144608139992,
-0.9));
#82535=CARTESIAN_POINT('',(-20.5646667256951,-53.0208728909492,-0.6));
#82536=CARTESIAN_POINT('Ctrl Pts',(-20.5646667256951,-53.0208728909492,
-0.6));
#82537=CARTESIAN_POINT('Ctrl Pts',(-20.7652804628015,-52.8144608139992,
-0.6));
#82538=CARTESIAN_POINT('Ctrl Pts',(-21.0899731889367,-52.8144608139992,
-0.6));
#82539=CARTESIAN_POINT('',(-20.5646667256951,-53.0208728909492,-0.9));
#82540=CARTESIAN_POINT('',(-20.5646667256951,-53.0208728909492,-0.6));
#82541=CARTESIAN_POINT('Ctrl Pts',(-20.5646667256951,-53.0208728909492,
-0.9));
#82542=CARTESIAN_POINT('Ctrl Pts',(-20.7652804628015,-52.8144608139992,
-0.9));
#82543=CARTESIAN_POINT('Ctrl Pts',(-21.0899731889367,-52.8144608139992,
-0.9));
#82544=CARTESIAN_POINT('Ctrl Pts',(-20.3640529885888,-53.584447324276,-0.6));
#82545=CARTESIAN_POINT('Ctrl Pts',(-20.3640529885888,-53.584447324276,-0.9));
#82546=CARTESIAN_POINT('Ctrl Pts',(-20.3640529885888,-53.2272849678993,
-0.6));
#82547=CARTESIAN_POINT('Ctrl Pts',(-20.3640529885888,-53.2272849678993,
-0.9));
#82548=CARTESIAN_POINT('Ctrl Pts',(-20.5646667256951,-53.0208728909492,
-0.6));
#82549=CARTESIAN_POINT('Ctrl Pts',(-20.5646667256951,-53.0208728909492,
-0.9));
#82550=CARTESIAN_POINT('',(-20.3640529885888,-53.584447324276,-0.6));
#82551=CARTESIAN_POINT('Ctrl Pts',(-20.3640529885888,-53.584447324276,-0.6));
#82552=CARTESIAN_POINT('Ctrl Pts',(-20.3640529885888,-53.2272849678993,
-0.6));
#82553=CARTESIAN_POINT('Ctrl Pts',(-20.5646667256951,-53.0208728909492,
-0.6));
#82554=CARTESIAN_POINT('',(-20.3640529885888,-53.584447324276,-0.9));
#82555=CARTESIAN_POINT('',(-20.3640529885888,-53.584447324276,-0.6));
#82556=CARTESIAN_POINT('Ctrl Pts',(-20.3640529885888,-53.584447324276,-0.9));
#82557=CARTESIAN_POINT('Ctrl Pts',(-20.3640529885888,-53.2272849678993,
-0.9));
#82558=CARTESIAN_POINT('Ctrl Pts',(-20.5646667256951,-53.0208728909492,
-0.9));
#82559=CARTESIAN_POINT('Ctrl Pts',(-20.5727836862206,-54.1874490380287,
-0.6));
#82560=CARTESIAN_POINT('Ctrl Pts',(-20.5727836862206,-54.1874490380287,
-0.9));
#82561=CARTESIAN_POINT('Ctrl Pts',(-20.3640529885888,-53.9601640105247,
-0.6));
#82562=CARTESIAN_POINT('Ctrl Pts',(-20.3640529885888,-53.9601640105247,
-0.9));
#82563=CARTESIAN_POINT('Ctrl Pts',(-20.3640529885888,-53.584447324276,-0.6));
#82564=CARTESIAN_POINT('Ctrl Pts',(-20.3640529885888,-53.584447324276,-0.9));
#82565=CARTESIAN_POINT('',(-20.5727836862206,-54.1874490380287,-0.6));
#82566=CARTESIAN_POINT('Ctrl Pts',(-20.5727836862206,-54.1874490380287,
-0.6));
#82567=CARTESIAN_POINT('Ctrl Pts',(-20.3640529885888,-53.9601640105247,
-0.6));
#82568=CARTESIAN_POINT('Ctrl Pts',(-20.3640529885888,-53.584447324276,-0.6));
#82569=CARTESIAN_POINT('',(-20.5727836862206,-54.1874490380287,-0.9));
#82570=CARTESIAN_POINT('',(-20.5727836862206,-54.1874490380287,-0.6));
#82571=CARTESIAN_POINT('Ctrl Pts',(-20.5727836862206,-54.1874490380287,
-0.9));
#82572=CARTESIAN_POINT('Ctrl Pts',(-20.3640529885888,-53.9601640105247,
-0.9));
#82573=CARTESIAN_POINT('Ctrl Pts',(-20.3640529885888,-53.584447324276,-0.9));
#82574=CARTESIAN_POINT('Ctrl Pts',(-21.0830161347985,-54.4147340655327,
-0.6));
#82575=CARTESIAN_POINT('Ctrl Pts',(-21.0830161347985,-54.4147340655327,
-0.9));
#82576=CARTESIAN_POINT('Ctrl Pts',(-20.7815155759454,-54.4147340655327,
-0.6));
#82577=CARTESIAN_POINT('Ctrl Pts',(-20.7815155759454,-54.4147340655327,
-0.9));
#82578=CARTESIAN_POINT('Ctrl Pts',(-20.5727836862206,-54.1874490380287,
-0.6));
#82579=CARTESIAN_POINT('Ctrl Pts',(-20.5727836862206,-54.1874490380287,
-0.9));
#82580=CARTESIAN_POINT('',(-21.0830161347985,-54.4147340655327,-0.6));
#82581=CARTESIAN_POINT('Ctrl Pts',(-21.0830161347985,-54.4147340655327,
-0.6));
#82582=CARTESIAN_POINT('Ctrl Pts',(-20.7815155759454,-54.4147340655327,
-0.6));
#82583=CARTESIAN_POINT('Ctrl Pts',(-20.5727836862206,-54.1874490380287,
-0.6));
#82584=CARTESIAN_POINT('',(-21.0830161347985,-54.4147340655327,-0.9));
#82585=CARTESIAN_POINT('',(-21.0830161347985,-54.4147340655327,-0.6));
#82586=CARTESIAN_POINT('Ctrl Pts',(-21.0830161347985,-54.4147340655327,
-0.9));
#82587=CARTESIAN_POINT('Ctrl Pts',(-20.7815155759454,-54.4147340655327,
-0.9));
#82588=CARTESIAN_POINT('Ctrl Pts',(-20.5727836862206,-54.1874490380287,
-0.9));
#82589=CARTESIAN_POINT('Ctrl Pts',(-21.5109154954553,-54.2535470128059,
-0.6));
#82590=CARTESIAN_POINT('Ctrl Pts',(-21.5109154954553,-54.2535470128059,
-0.9));
#82591=CARTESIAN_POINT('Ctrl Pts',(-21.333493925631,-54.4147340655327,-0.6));
#82592=CARTESIAN_POINT('Ctrl Pts',(-21.333493925631,-54.4147340655327,-0.9));
#82593=CARTESIAN_POINT('Ctrl Pts',(-21.0830161347985,-54.4147340655327,
-0.6));
#82594=CARTESIAN_POINT('Ctrl Pts',(-21.0830161347985,-54.4147340655327,
-0.9));
#82595=CARTESIAN_POINT('',(-21.5109154954553,-54.2535470128059,-0.6));
#82596=CARTESIAN_POINT('Ctrl Pts',(-21.5109154954553,-54.2535470128059,
-0.6));
#82597=CARTESIAN_POINT('Ctrl Pts',(-21.333493925631,-54.4147340655327,-0.6));
#82598=CARTESIAN_POINT('Ctrl Pts',(-21.0830161347985,-54.4147340655327,
-0.6));
#82599=CARTESIAN_POINT('',(-21.5109154954553,-54.2535470128059,-0.9));
#82600=CARTESIAN_POINT('',(-21.5109154954553,-54.2535470128059,-0.6));
#82601=CARTESIAN_POINT('Ctrl Pts',(-21.5109154954553,-54.2535470128059,
-0.9));
#82602=CARTESIAN_POINT('Ctrl Pts',(-21.333493925631,-54.4147340655327,-0.9));
#82603=CARTESIAN_POINT('Ctrl Pts',(-21.0830161347985,-54.4147340655327,
-0.9));
#82604=CARTESIAN_POINT('Ctrl Pts',(-21.7370400205255,-53.7723056674004,
-0.6));
#82605=CARTESIAN_POINT('Ctrl Pts',(-21.7370400205255,-53.7723056674004,
-0.9));
#82606=CARTESIAN_POINT('Ctrl Pts',(-21.6883370652795,-54.0923599600792,
-0.6));
#82607=CARTESIAN_POINT('Ctrl Pts',(-21.6883370652795,-54.0923599600792,
-0.9));
#82608=CARTESIAN_POINT('Ctrl Pts',(-21.5109154954553,-54.2535470128059,
-0.6));
#82609=CARTESIAN_POINT('Ctrl Pts',(-21.5109154954553,-54.2535470128059,
-0.9));
#82610=CARTESIAN_POINT('',(-21.7370400205255,-53.7723056674004,-0.6));
#82611=CARTESIAN_POINT('Ctrl Pts',(-21.7370400205255,-53.7723056674004,
-0.6));
#82612=CARTESIAN_POINT('Ctrl Pts',(-21.6883370652795,-54.0923599600792,
-0.6));
#82613=CARTESIAN_POINT('Ctrl Pts',(-21.5109154954553,-54.2535470128059,
-0.6));
#82614=CARTESIAN_POINT('',(-21.7370400205255,-53.7723056674004,-0.9));
#82615=CARTESIAN_POINT('',(-21.7370400205255,-53.7723056674004,-0.6));
#82616=CARTESIAN_POINT('Ctrl Pts',(-21.7370400205255,-53.7723056674004,
-0.9));
#82617=CARTESIAN_POINT('Ctrl Pts',(-21.6883370652795,-54.0923599600792,
-0.9));
#82618=CARTESIAN_POINT('Ctrl Pts',(-21.5109154954553,-54.2535470128059,
-0.9));
#82619=CARTESIAN_POINT('Origin',(-22.1753761544824,-53.8094131350517,-0.6));
#82620=CARTESIAN_POINT('',(-22.1753761544824,-53.8094131350517,-0.6));
#82621=CARTESIAN_POINT('',(-11.1325660081367,-52.8745809627946,-0.6));
#82622=CARTESIAN_POINT('',(-22.1753761544824,-53.8094131350517,-0.9));
#82623=CARTESIAN_POINT('',(-22.1753761544824,-53.8094131350517,-0.6));
#82624=CARTESIAN_POINT('',(-22.1753761544824,-53.8094131350517,-0.9));
#82625=CARTESIAN_POINT('Ctrl Pts',(-21.8402466550469,-54.4982264637947,
-0.6));
#82626=CARTESIAN_POINT('Ctrl Pts',(-21.8402466550469,-54.4982264637947,
-0.9));
#82627=CARTESIAN_POINT('Ctrl Pts',(-22.1336302533746,-54.2384724020958,
-0.6));
#82628=CARTESIAN_POINT('Ctrl Pts',(-22.1336302533746,-54.2384724020958,
-0.9));
#82629=CARTESIAN_POINT('Ctrl Pts',(-22.1753761544824,-53.8094131350517,
-0.6));
#82630=CARTESIAN_POINT('Ctrl Pts',(-22.1753761544824,-53.8094131350517,
-0.9));
#82631=CARTESIAN_POINT('',(-21.8402466550469,-54.4982264637947,-0.6));
#82632=CARTESIAN_POINT('Ctrl Pts',(-21.8402466550469,-54.4982264637947,
-0.6));
#82633=CARTESIAN_POINT('Ctrl Pts',(-22.1336302533746,-54.2384724020958,
-0.6));
#82634=CARTESIAN_POINT('Ctrl Pts',(-22.1753761544824,-53.8094131350517,
-0.6));
#82635=CARTESIAN_POINT('',(-21.8402466550469,-54.4982264637947,-0.9));
#82636=CARTESIAN_POINT('',(-21.8402466550469,-54.4982264637947,-0.6));
#82637=CARTESIAN_POINT('Ctrl Pts',(-21.8402466550469,-54.4982264637947,
-0.9));
#82638=CARTESIAN_POINT('Ctrl Pts',(-22.1336302533746,-54.2384724020958,
-0.9));
#82639=CARTESIAN_POINT('Ctrl Pts',(-22.1753761544824,-53.8094131350517,
-0.9));
#82640=CARTESIAN_POINT('Ctrl Pts',(-21.0830161347985,-54.7579811215401,
-0.6));
#82641=CARTESIAN_POINT('Ctrl Pts',(-21.0830161347985,-54.7579811215401,
-0.9));
#82642=CARTESIAN_POINT('Ctrl Pts',(-21.5468630567193,-54.7579811215401,
-0.6));
#82643=CARTESIAN_POINT('Ctrl Pts',(-21.5468630567193,-54.7579811215401,
-0.9));
#82644=CARTESIAN_POINT('Ctrl Pts',(-21.8402466550469,-54.4982264637947,
-0.6));
#82645=CARTESIAN_POINT('Ctrl Pts',(-21.8402466550469,-54.4982264637947,
-0.9));
#82646=CARTESIAN_POINT('Ctrl Pts',(-21.0830161347985,-54.7579811215401,
-0.6));
#82647=CARTESIAN_POINT('Ctrl Pts',(-21.5468630567193,-54.7579811215401,
-0.6));
#82648=CARTESIAN_POINT('Ctrl Pts',(-21.8402466550469,-54.4982264637947,
-0.6));
#82649=CARTESIAN_POINT('Ctrl Pts',(-21.0830161347985,-54.7579811215401,
-0.9));
#82650=CARTESIAN_POINT('Ctrl Pts',(-21.5468630567193,-54.7579811215401,
-0.9));
#82651=CARTESIAN_POINT('Ctrl Pts',(-21.8402466550469,-54.4982264637947,
-0.9));
#82652=CARTESIAN_POINT('Origin',(-21.0482272878289,-53.0521829128265,-0.9));
#82653=CARTESIAN_POINT('Ctrl Pts',(-13.8261279836297,-54.7579811215401,
-0.6));
#82654=CARTESIAN_POINT('Ctrl Pts',(-13.8261279836297,-54.7579811215401,
-0.9));
#82655=CARTESIAN_POINT('Ctrl Pts',(-14.3062100186944,-54.7579811215401,
-0.6));
#82656=CARTESIAN_POINT('Ctrl Pts',(-14.3062100186944,-54.7579811215401,
-0.9));
#82657=CARTESIAN_POINT('Ctrl Pts',(-14.684244133532,-54.5260576605797,-0.6));
#82658=CARTESIAN_POINT('Ctrl Pts',(-14.684244133532,-54.5260576605797,-0.9));
#82659=CARTESIAN_POINT('',(-13.8261279836297,-54.7579811215401,-0.6));
#82660=CARTESIAN_POINT('',(-14.684244133532,-54.5260576605797,-0.6));
#82661=CARTESIAN_POINT('Ctrl Pts',(-13.8261279836297,-54.7579811215401,
-0.6));
#82662=CARTESIAN_POINT('Ctrl Pts',(-14.3062100186944,-54.7579811215401,
-0.6));
#82663=CARTESIAN_POINT('Ctrl Pts',(-14.684244133532,-54.5260576605797,-0.6));
#82664=CARTESIAN_POINT('',(-13.8261279836297,-54.7579811215401,-0.9));
#82665=CARTESIAN_POINT('',(-13.8261279836297,-54.7579811215401,-0.6));
#82666=CARTESIAN_POINT('',(-14.684244133532,-54.5260576605797,-0.9));
#82667=CARTESIAN_POINT('Ctrl Pts',(-13.8261279836297,-54.7579811215401,
-0.9));
#82668=CARTESIAN_POINT('Ctrl Pts',(-14.3062100186944,-54.7579811215401,
-0.9));
#82669=CARTESIAN_POINT('Ctrl Pts',(-14.684244133532,-54.5260576605797,-0.9));
#82670=CARTESIAN_POINT('',(-14.684244133532,-54.5260576605797,-0.6));
#82671=CARTESIAN_POINT('Ctrl Pts',(-13.0004796758294,-54.5480899214745,
-0.6));
#82672=CARTESIAN_POINT('Ctrl Pts',(-13.0004796758294,-54.5480899214745,
-0.9));
#82673=CARTESIAN_POINT('Ctrl Pts',(-13.3831534162164,-54.7579811215401,
-0.6));
#82674=CARTESIAN_POINT('Ctrl Pts',(-13.3831534162164,-54.7579811215401,
-0.9));
#82675=CARTESIAN_POINT('Ctrl Pts',(-13.8261279836297,-54.7579811215401,
-0.6));
#82676=CARTESIAN_POINT('Ctrl Pts',(-13.8261279836297,-54.7579811215401,
-0.9));
#82677=CARTESIAN_POINT('',(-13.0004796758294,-54.5480899214745,-0.6));
#82678=CARTESIAN_POINT('Ctrl Pts',(-13.0004796758294,-54.5480899214745,
-0.6));
#82679=CARTESIAN_POINT('Ctrl Pts',(-13.3831534162164,-54.7579811215401,
-0.6));
#82680=CARTESIAN_POINT('Ctrl Pts',(-13.8261279836297,-54.7579811215401,
-0.6));
#82681=CARTESIAN_POINT('',(-13.0004796758294,-54.5480899214745,-0.9));
#82682=CARTESIAN_POINT('',(-13.0004796758294,-54.5480899214745,-0.6));
#82683=CARTESIAN_POINT('Ctrl Pts',(-13.0004796758294,-54.5480899214745,
-0.9));
#82684=CARTESIAN_POINT('Ctrl Pts',(-13.3831534162164,-54.7579811215401,
-0.9));
#82685=CARTESIAN_POINT('Ctrl Pts',(-13.8261279836297,-54.7579811215401,
-0.9));
#82686=CARTESIAN_POINT('Ctrl Pts',(-12.4090728536248,-53.9300135970116,
-0.6));
#82687=CARTESIAN_POINT('Ctrl Pts',(-12.4090728536248,-53.9300135970116,
-0.9));
#82688=CARTESIAN_POINT('Ctrl Pts',(-12.6178059354424,-54.3381993174553,
-0.6));
#82689=CARTESIAN_POINT('Ctrl Pts',(-12.6178059354424,-54.3381993174553,
-0.9));
#82690=CARTESIAN_POINT('Ctrl Pts',(-13.0004796758294,-54.5480899214745,
-0.6));
#82691=CARTESIAN_POINT('Ctrl Pts',(-13.0004796758294,-54.5480899214745,
-0.9));
#82692=CARTESIAN_POINT('',(-12.4090728536248,-53.9300135970116,-0.6));
#82693=CARTESIAN_POINT('Ctrl Pts',(-12.4090728536248,-53.9300135970116,
-0.6));
#82694=CARTESIAN_POINT('Ctrl Pts',(-12.6178059354424,-54.3381993174553,
-0.6));
#82695=CARTESIAN_POINT('Ctrl Pts',(-13.0004796758294,-54.5480899214745,
-0.6));
#82696=CARTESIAN_POINT('',(-12.4090728536248,-53.9300135970116,-0.9));
#82697=CARTESIAN_POINT('',(-12.4090728536248,-53.9300135970116,-0.6));
#82698=CARTESIAN_POINT('Ctrl Pts',(-12.4090728536248,-53.9300135970116,
-0.9));
#82699=CARTESIAN_POINT('Ctrl Pts',(-12.6178059354424,-54.3381993174553,
-0.9));
#82700=CARTESIAN_POINT('Ctrl Pts',(-13.0004796758294,-54.5480899214745,
-0.9));
#82701=CARTESIAN_POINT('Ctrl Pts',(-12.200342155993,-53.0046383738518,-0.6));
#82702=CARTESIAN_POINT('Ctrl Pts',(-12.200342155993,-53.0046383738518,-0.9));
#82703=CARTESIAN_POINT('Ctrl Pts',(-12.200342155993,-53.5218278765678,-0.6));
#82704=CARTESIAN_POINT('Ctrl Pts',(-12.200342155993,-53.5218278765678,-0.9));
#82705=CARTESIAN_POINT('Ctrl Pts',(-12.4090728536248,-53.9300135970116,
-0.6));
#82706=CARTESIAN_POINT('Ctrl Pts',(-12.4090728536248,-53.9300135970116,
-0.9));
#82707=CARTESIAN_POINT('',(-12.200342155993,-53.0046383738518,-0.6));
#82708=CARTESIAN_POINT('Ctrl Pts',(-12.200342155993,-53.0046383738518,-0.6));
#82709=CARTESIAN_POINT('Ctrl Pts',(-12.200342155993,-53.5218278765678,-0.6));
#82710=CARTESIAN_POINT('Ctrl Pts',(-12.4090728536248,-53.9300135970116,
-0.6));
#82711=CARTESIAN_POINT('',(-12.200342155993,-53.0046383738518,-0.9));
#82712=CARTESIAN_POINT('',(-12.200342155993,-53.0046383738518,-0.6));
#82713=CARTESIAN_POINT('Ctrl Pts',(-12.200342155993,-53.0046383738518,-0.9));
#82714=CARTESIAN_POINT('Ctrl Pts',(-12.200342155993,-53.5218278765678,-0.9));
#82715=CARTESIAN_POINT('Ctrl Pts',(-12.4090728536248,-53.9300135970116,
-0.9));
#82716=CARTESIAN_POINT('Ctrl Pts',(-12.3986372724175,-52.0920191407204,
-0.6));
#82717=CARTESIAN_POINT('Ctrl Pts',(-12.3986372724175,-52.0920191407204,
-0.9));
#82718=CARTESIAN_POINT('Ctrl Pts',(-12.200342155993,-52.4944065213203,-0.6));
#82719=CARTESIAN_POINT('Ctrl Pts',(-12.200342155993,-52.4944065213203,-0.9));
#82720=CARTESIAN_POINT('Ctrl Pts',(-12.200342155993,-53.0046383738518,-0.6));
#82721=CARTESIAN_POINT('Ctrl Pts',(-12.200342155993,-53.0046383738518,-0.9));
#82722=CARTESIAN_POINT('',(-12.3986372724175,-52.0920191407204,-0.6));
#82723=CARTESIAN_POINT('Ctrl Pts',(-12.3986372724175,-52.0920191407204,
-0.6));
#82724=CARTESIAN_POINT('Ctrl Pts',(-12.200342155993,-52.4944065213203,-0.6));
#82725=CARTESIAN_POINT('Ctrl Pts',(-12.200342155993,-53.0046383738518,-0.6));
#82726=CARTESIAN_POINT('',(-12.3986372724175,-52.0920191407204,-0.9));
#82727=CARTESIAN_POINT('',(-12.3986372724175,-52.0920191407204,-0.6));
#82728=CARTESIAN_POINT('Ctrl Pts',(-12.3986372724175,-52.0920191407204,
-0.9));
#82729=CARTESIAN_POINT('Ctrl Pts',(-12.200342155993,-52.4944065213203,-0.9));
#82730=CARTESIAN_POINT('Ctrl Pts',(-12.200342155993,-53.0046383738518,-0.9));
#82731=CARTESIAN_POINT('Ctrl Pts',(-12.9749665036798,-51.4646653532982,
-0.6));
#82732=CARTESIAN_POINT('Ctrl Pts',(-12.9749665036798,-51.4646653532982,
-0.9));
#82733=CARTESIAN_POINT('Ctrl Pts',(-12.5969323888421,-51.6896311640739,
-0.6));
#82734=CARTESIAN_POINT('Ctrl Pts',(-12.5969323888421,-51.6896311640739,
-0.9));
#82735=CARTESIAN_POINT('Ctrl Pts',(-12.3986372724175,-52.0920191407204,
-0.6));
#82736=CARTESIAN_POINT('Ctrl Pts',(-12.3986372724175,-52.0920191407204,
-0.9));
#82737=CARTESIAN_POINT('',(-12.9749665036798,-51.4646653532982,-0.6));
#82738=CARTESIAN_POINT('Ctrl Pts',(-12.9749665036798,-51.4646653532982,
-0.6));
#82739=CARTESIAN_POINT('Ctrl Pts',(-12.5969323888421,-51.6896311640739,
-0.6));
#82740=CARTESIAN_POINT('Ctrl Pts',(-12.3986372724175,-52.0920191407204,
-0.6));
#82741=CARTESIAN_POINT('',(-12.9749665036798,-51.4646653532982,-0.9));
#82742=CARTESIAN_POINT('',(-12.9749665036798,-51.4646653532982,-0.6));
#82743=CARTESIAN_POINT('Ctrl Pts',(-12.9749665036798,-51.4646653532982,
-0.9));
#82744=CARTESIAN_POINT('Ctrl Pts',(-12.5969323888421,-51.6896311640739,
-0.9));
#82745=CARTESIAN_POINT('Ctrl Pts',(-12.3986372724175,-52.0920191407204,
-0.9));
#82746=CARTESIAN_POINT('Ctrl Pts',(-13.823808170855,-51.2396995425224,-0.6));
#82747=CARTESIAN_POINT('Ctrl Pts',(-13.823808170855,-51.2396995425224,-0.9));
#82748=CARTESIAN_POINT('Ctrl Pts',(-13.3530030027032,-51.2396995425224,
-0.6));
#82749=CARTESIAN_POINT('Ctrl Pts',(-13.3530030027032,-51.2396995425224,
-0.9));
#82750=CARTESIAN_POINT('Ctrl Pts',(-12.9749665036798,-51.4646653532982,
-0.6));
#82751=CARTESIAN_POINT('Ctrl Pts',(-12.9749665036798,-51.4646653532982,
-0.9));
#82752=CARTESIAN_POINT('',(-13.823808170855,-51.2396995425224,-0.6));
#82753=CARTESIAN_POINT('Ctrl Pts',(-13.823808170855,-51.2396995425224,-0.6));
#82754=CARTESIAN_POINT('Ctrl Pts',(-13.3530030027032,-51.2396995425224,
-0.6));
#82755=CARTESIAN_POINT('Ctrl Pts',(-12.9749665036798,-51.4646653532982,
-0.6));
#82756=CARTESIAN_POINT('',(-13.823808170855,-51.2396995425224,-0.9));
#82757=CARTESIAN_POINT('',(-13.823808170855,-51.2396995425224,-0.6));
#82758=CARTESIAN_POINT('Ctrl Pts',(-13.823808170855,-51.2396995425224,-0.9));
#82759=CARTESIAN_POINT('Ctrl Pts',(-13.3530030027032,-51.2396995425224,
-0.9));
#82760=CARTESIAN_POINT('Ctrl Pts',(-12.9749665036798,-51.4646653532982,
-0.9));
#82761=CARTESIAN_POINT('Ctrl Pts',(-14.9973401799798,-51.7186216711998,
-0.6));
#82762=CARTESIAN_POINT('Ctrl Pts',(-14.9973401799798,-51.7186216711998,
-0.9));
#82763=CARTESIAN_POINT('Ctrl Pts',(-14.5427713170648,-51.2396995425224,
-0.6));
#82764=CARTESIAN_POINT('Ctrl Pts',(-14.5427713170648,-51.2396995425224,
-0.9));
#82765=CARTESIAN_POINT('Ctrl Pts',(-13.823808170855,-51.2396995425224,-0.6));
#82766=CARTESIAN_POINT('Ctrl Pts',(-13.823808170855,-51.2396995425224,-0.9));
#82767=CARTESIAN_POINT('',(-14.9973401799798,-51.7186216711998,-0.6));
#82768=CARTESIAN_POINT('Ctrl Pts',(-14.9973401799798,-51.7186216711998,
-0.6));
#82769=CARTESIAN_POINT('Ctrl Pts',(-14.5427713170648,-51.2396995425224,
-0.6));
#82770=CARTESIAN_POINT('Ctrl Pts',(-13.823808170855,-51.2396995425224,-0.6));
#82771=CARTESIAN_POINT('',(-14.9973401799798,-51.7186216711998,-0.9));
#82772=CARTESIAN_POINT('',(-14.9973401799798,-51.7186216711998,-0.6));
#82773=CARTESIAN_POINT('Ctrl Pts',(-14.9973401799798,-51.7186216711998,
-0.9));
#82774=CARTESIAN_POINT('Ctrl Pts',(-14.5427713170648,-51.2396995425224,
-0.9));
#82775=CARTESIAN_POINT('Ctrl Pts',(-13.823808170855,-51.2396995425224,-0.9));
#82776=CARTESIAN_POINT('Ctrl Pts',(-15.4519114270806,-53.0440656542778,
-0.6));
#82777=CARTESIAN_POINT('Ctrl Pts',(-15.4519114270806,-53.0440656542778,
-0.9));
#82778=CARTESIAN_POINT('Ctrl Pts',(-15.4519114270806,-52.1975443959236,
-0.6));
#82779=CARTESIAN_POINT('Ctrl Pts',(-15.4519114270806,-52.1975443959236,
-0.9));
#82780=CARTESIAN_POINT('Ctrl Pts',(-14.9973401799798,-51.7186216711998,
-0.6));
#82781=CARTESIAN_POINT('Ctrl Pts',(-14.9973401799798,-51.7186216711998,
-0.9));
#82782=CARTESIAN_POINT('',(-15.4519114270806,-53.0440656542778,-0.6));
#82783=CARTESIAN_POINT('Ctrl Pts',(-15.4519114270806,-53.0440656542778,
-0.6));
#82784=CARTESIAN_POINT('Ctrl Pts',(-15.4519114270806,-52.1975443959236,
-0.6));
#82785=CARTESIAN_POINT('Ctrl Pts',(-14.9973401799798,-51.7186216711998,
-0.6));
#82786=CARTESIAN_POINT('',(-15.4519114270806,-53.0440656542778,-0.9));
#82787=CARTESIAN_POINT('',(-15.4519114270806,-53.0440656542778,-0.6));
#82788=CARTESIAN_POINT('Ctrl Pts',(-15.4519114270806,-53.0440656542778,
-0.9));
#82789=CARTESIAN_POINT('Ctrl Pts',(-15.4519114270806,-52.1975443959236,
-0.9));
#82790=CARTESIAN_POINT('Ctrl Pts',(-14.9973401799798,-51.7186216711998,
-0.9));
#82791=CARTESIAN_POINT('Ctrl Pts',(-15.2570960298181,-53.8929061293602,
-0.6));
#82792=CARTESIAN_POINT('Ctrl Pts',(-15.2570960298181,-53.8929061293602,
-0.9));
#82793=CARTESIAN_POINT('Ctrl Pts',(-15.4519114270806,-53.4916780591011,
-0.6));
#82794=CARTESIAN_POINT('Ctrl Pts',(-15.4519114270806,-53.4916780591011,
-0.9));
#82795=CARTESIAN_POINT('Ctrl Pts',(-15.4519114270806,-53.0440656542778,
-0.6));
#82796=CARTESIAN_POINT('Ctrl Pts',(-15.4519114270806,-53.0440656542778,
-0.9));
#82797=CARTESIAN_POINT('',(-15.2570960298181,-53.8929061293602,-0.6));
#82798=CARTESIAN_POINT('Ctrl Pts',(-15.2570960298181,-53.8929061293602,
-0.6));
#82799=CARTESIAN_POINT('Ctrl Pts',(-15.4519114270806,-53.4916780591011,
-0.6));
#82800=CARTESIAN_POINT('Ctrl Pts',(-15.4519114270806,-53.0440656542778,
-0.6));
#82801=CARTESIAN_POINT('',(-15.2570960298181,-53.8929061293602,-0.9));
#82802=CARTESIAN_POINT('',(-15.2570960298181,-53.8929061293602,-0.6));
#82803=CARTESIAN_POINT('Ctrl Pts',(-15.2570960298181,-53.8929061293602,
-0.9));
#82804=CARTESIAN_POINT('Ctrl Pts',(-15.4519114270806,-53.4916780591011,
-0.9));
#82805=CARTESIAN_POINT('Ctrl Pts',(-15.4519114270806,-53.0440656542778,
-0.9));
#82806=CARTESIAN_POINT('Ctrl Pts',(-14.684244133532,-54.5260576605797,-0.6));
#82807=CARTESIAN_POINT('Ctrl Pts',(-14.684244133532,-54.5260576605797,-0.9));
#82808=CARTESIAN_POINT('Ctrl Pts',(-15.0622806325555,-54.2941336035728,
-0.6));
#82809=CARTESIAN_POINT('Ctrl Pts',(-15.0622806325555,-54.2941336035728,
-0.9));
#82810=CARTESIAN_POINT('Ctrl Pts',(-15.2570960298181,-53.8929061293602,
-0.6));
#82811=CARTESIAN_POINT('Ctrl Pts',(-15.2570960298181,-53.8929061293602,
-0.9));
#82812=CARTESIAN_POINT('Ctrl Pts',(-14.684244133532,-54.5260576605797,-0.6));
#82813=CARTESIAN_POINT('Ctrl Pts',(-15.0622806325555,-54.2941336035728,
-0.6));
#82814=CARTESIAN_POINT('Ctrl Pts',(-15.2570960298181,-53.8929061293602,
-0.6));
#82815=CARTESIAN_POINT('Ctrl Pts',(-14.684244133532,-54.5260576605797,-0.9));
#82816=CARTESIAN_POINT('Ctrl Pts',(-15.0622806325555,-54.2941336035728,
-0.9));
#82817=CARTESIAN_POINT('Ctrl Pts',(-15.2570960298181,-53.8929061293602,
-0.9));
#82818=CARTESIAN_POINT('Origin',(-13.8261267915368,-52.9988403320313,-0.9));
#82819=CARTESIAN_POINT('Ctrl Pts',(-5.29945466667414,-52.0896999239922,
-0.6));
#82820=CARTESIAN_POINT('Ctrl Pts',(-5.29945466667414,-52.0896999239922,
-0.9));
#82821=CARTESIAN_POINT('Ctrl Pts',(-5.10115955024958,-52.4920873045921,
-0.6));
#82822=CARTESIAN_POINT('Ctrl Pts',(-5.10115955024958,-52.4920873045921,
-0.9));
#82823=CARTESIAN_POINT('Ctrl Pts',(-5.10115955024958,-52.9976807236671,
-0.6));
#82824=CARTESIAN_POINT('Ctrl Pts',(-5.10115955024958,-52.9976807236671,
-0.9));
#82825=CARTESIAN_POINT('',(-5.29945466667414,-52.0896999239922,-0.6));
#82826=CARTESIAN_POINT('',(-5.10115955024958,-52.9976807236671,-0.6));
#82827=CARTESIAN_POINT('Ctrl Pts',(-5.29945466667414,-52.0896999239922,
-0.6));
#82828=CARTESIAN_POINT('Ctrl Pts',(-5.10115955024958,-52.4920873045921,
-0.6));
#82829=CARTESIAN_POINT('Ctrl Pts',(-5.10115955024958,-52.9976807236671,
-0.6));
#82830=CARTESIAN_POINT('',(-5.29945466667414,-52.0896999239922,-0.9));
#82831=CARTESIAN_POINT('',(-5.29945466667414,-52.0896999239922,-0.6));
#82832=CARTESIAN_POINT('',(-5.10115955024958,-52.9976807236671,-0.9));
#82833=CARTESIAN_POINT('Ctrl Pts',(-5.29945466667414,-52.0896999239922,
-0.9));
#82834=CARTESIAN_POINT('Ctrl Pts',(-5.10115955024958,-52.4920873045921,
-0.9));
#82835=CARTESIAN_POINT('Ctrl Pts',(-5.10115955024958,-52.9976807236671,
-0.9));
#82836=CARTESIAN_POINT('',(-5.10115955024958,-52.9976807236671,-0.6));
#82837=CARTESIAN_POINT('Ctrl Pts',(-5.87578389793634,-51.4635060429573,
-0.6));
#82838=CARTESIAN_POINT('Ctrl Pts',(-5.87578389793634,-51.4635060429573,
-0.9));
#82839=CARTESIAN_POINT('Ctrl Pts',(-5.4977497830987,-51.6873125433922,-0.6));
#82840=CARTESIAN_POINT('Ctrl Pts',(-5.4977497830987,-51.6873125433922,-0.9));
#82841=CARTESIAN_POINT('Ctrl Pts',(-5.29945466667414,-52.0896999239922,
-0.6));
#82842=CARTESIAN_POINT('Ctrl Pts',(-5.29945466667414,-52.0896999239922,
-0.9));
#82843=CARTESIAN_POINT('',(-5.87578389793634,-51.4635060429573,-0.6));
#82844=CARTESIAN_POINT('Ctrl Pts',(-5.87578389793634,-51.4635060429573,
-0.6));
#82845=CARTESIAN_POINT('Ctrl Pts',(-5.4977497830987,-51.6873125433922,-0.6));
#82846=CARTESIAN_POINT('Ctrl Pts',(-5.29945466667414,-52.0896999239922,
-0.6));
#82847=CARTESIAN_POINT('',(-5.87578389793634,-51.4635060429573,-0.9));
#82848=CARTESIAN_POINT('',(-5.87578389793634,-51.4635060429573,-0.6));
#82849=CARTESIAN_POINT('Ctrl Pts',(-5.87578389793634,-51.4635060429573,
-0.9));
#82850=CARTESIAN_POINT('Ctrl Pts',(-5.4977497830987,-51.6873125433922,-0.9));
#82851=CARTESIAN_POINT('Ctrl Pts',(-5.29945466667414,-52.0896999239922,
-0.9));
#82852=CARTESIAN_POINT('Ctrl Pts',(-6.72462556511164,-51.2396995425224,
-0.6));
#82853=CARTESIAN_POINT('Ctrl Pts',(-6.72462556511164,-51.2396995425224,
-0.9));
#82854=CARTESIAN_POINT('Ctrl Pts',(-6.25382039695978,-51.2396995425224,
-0.6));
#82855=CARTESIAN_POINT('Ctrl Pts',(-6.25382039695978,-51.2396995425224,
-0.9));
#82856=CARTESIAN_POINT('Ctrl Pts',(-5.87578389793634,-51.4635060429573,
-0.6));
#82857=CARTESIAN_POINT('Ctrl Pts',(-5.87578389793634,-51.4635060429573,
-0.9));
#82858=CARTESIAN_POINT('',(-6.72462556511164,-51.2396995425224,-0.6));
#82859=CARTESIAN_POINT('Ctrl Pts',(-6.72462556511164,-51.2396995425224,
-0.6));
#82860=CARTESIAN_POINT('Ctrl Pts',(-6.25382039695978,-51.2396995425224,
-0.6));
#82861=CARTESIAN_POINT('Ctrl Pts',(-5.87578389793634,-51.4635060429573,
-0.6));
#82862=CARTESIAN_POINT('',(-6.72462556511164,-51.2396995425224,-0.9));
#82863=CARTESIAN_POINT('',(-6.72462556511164,-51.2396995425224,-0.6));
#82864=CARTESIAN_POINT('Ctrl Pts',(-6.72462556511164,-51.2396995425224,
-0.9));
#82865=CARTESIAN_POINT('Ctrl Pts',(-6.25382039695978,-51.2396995425224,
-0.9));
#82866=CARTESIAN_POINT('Ctrl Pts',(-5.87578389793634,-51.4635060429573,
-0.9));
#82867=CARTESIAN_POINT('Ctrl Pts',(-7.56766650825739,-51.4553884863853,
-0.6));
#82868=CARTESIAN_POINT('Ctrl Pts',(-7.56766650825739,-51.4553884863853,
-0.9));
#82869=CARTESIAN_POINT('Ctrl Pts',(-7.19079110771418,-51.2396995425224,
-0.6));
#82870=CARTESIAN_POINT('Ctrl Pts',(-7.19079110771418,-51.2396995425224,
-0.9));
#82871=CARTESIAN_POINT('Ctrl Pts',(-6.72462556511164,-51.2396995425224,
-0.6));
#82872=CARTESIAN_POINT('Ctrl Pts',(-6.72462556511164,-51.2396995425224,
-0.9));
#82873=CARTESIAN_POINT('',(-7.56766650825739,-51.4553884863853,-0.6));
#82874=CARTESIAN_POINT('Ctrl Pts',(-7.56766650825739,-51.4553884863853,
-0.6));
#82875=CARTESIAN_POINT('Ctrl Pts',(-7.19079110771418,-51.2396995425224,
-0.6));
#82876=CARTESIAN_POINT('Ctrl Pts',(-6.72462556511164,-51.2396995425224,
-0.6));
#82877=CARTESIAN_POINT('',(-7.56766650825739,-51.4553884863853,-0.9));
#82878=CARTESIAN_POINT('',(-7.56766650825739,-51.4553884863853,-0.6));
#82879=CARTESIAN_POINT('Ctrl Pts',(-7.56766650825739,-51.4553884863853,
-0.9));
#82880=CARTESIAN_POINT('Ctrl Pts',(-7.19079110771418,-51.2396995425224,
-0.9));
#82881=CARTESIAN_POINT('Ctrl Pts',(-6.72462556511164,-51.2396995425224,
-0.9));
#82882=CARTESIAN_POINT('Ctrl Pts',(-8.14863536506891,-52.0839015841484,
-0.6));
#82883=CARTESIAN_POINT('Ctrl Pts',(-8.14863536506891,-52.0839015841484,
-0.9));
#82884=CARTESIAN_POINT('Ctrl Pts',(-7.94454429298639,-51.6710774302483,
-0.6));
#82885=CARTESIAN_POINT('Ctrl Pts',(-7.94454429298639,-51.6710774302483,
-0.9));
#82886=CARTESIAN_POINT('Ctrl Pts',(-7.56766650825739,-51.4553884863853,
-0.6));
#82887=CARTESIAN_POINT('Ctrl Pts',(-7.56766650825739,-51.4553884863853,
-0.9));
#82888=CARTESIAN_POINT('',(-8.14863536506891,-52.0839015841484,-0.6));
#82889=CARTESIAN_POINT('Ctrl Pts',(-8.14863536506891,-52.0839015841484,
-0.6));
#82890=CARTESIAN_POINT('Ctrl Pts',(-7.94454429298639,-51.6710774302483,
-0.6));
#82891=CARTESIAN_POINT('Ctrl Pts',(-7.56766650825739,-51.4553884863853,
-0.6));
#82892=CARTESIAN_POINT('',(-8.14863536506891,-52.0839015841484,-0.9));
#82893=CARTESIAN_POINT('',(-8.14863536506891,-52.0839015841484,-0.6));
#82894=CARTESIAN_POINT('Ctrl Pts',(-8.14863536506891,-52.0839015841484,
-0.9));
#82895=CARTESIAN_POINT('Ctrl Pts',(-7.94454429298639,-51.6710774302483,
-0.9));
#82896=CARTESIAN_POINT('Ctrl Pts',(-7.56766650825739,-51.4553884863853,
-0.9));
#82897=CARTESIAN_POINT('Ctrl Pts',(-8.35272882133722,-52.9999999403954,
-0.6));
#82898=CARTESIAN_POINT('Ctrl Pts',(-8.35272882133722,-52.9999999403954,
-0.9));
#82899=CARTESIAN_POINT('Ctrl Pts',(-8.35272882133722,-52.4967257380486,
-0.6));
#82900=CARTESIAN_POINT('Ctrl Pts',(-8.35272882133722,-52.4967257380486,
-0.9));
#82901=CARTESIAN_POINT('Ctrl Pts',(-8.14863536506891,-52.0839015841484,
-0.6));
#82902=CARTESIAN_POINT('Ctrl Pts',(-8.14863536506891,-52.0839015841484,
-0.9));
#82903=CARTESIAN_POINT('',(-8.35272882133722,-52.9999999403954,-0.6));
#82904=CARTESIAN_POINT('Ctrl Pts',(-8.35272882133722,-52.9999999403954,
-0.6));
#82905=CARTESIAN_POINT('Ctrl Pts',(-8.35272882133722,-52.4967257380486,
-0.6));
#82906=CARTESIAN_POINT('Ctrl Pts',(-8.14863536506891,-52.0839015841484,
-0.6));
#82907=CARTESIAN_POINT('',(-8.35272882133722,-52.9999999403954,-0.9));
#82908=CARTESIAN_POINT('',(-8.35272882133722,-52.9999999403954,-0.6));
#82909=CARTESIAN_POINT('Ctrl Pts',(-8.35272882133722,-52.9999999403954,
-0.9));
#82910=CARTESIAN_POINT('Ctrl Pts',(-8.35272882133722,-52.4967257380486,
-0.9));
#82911=CARTESIAN_POINT('Ctrl Pts',(-8.14863536506891,-52.0839015841484,
-0.9));
#82912=CARTESIAN_POINT('Ctrl Pts',(-8.14979646354914,-53.9091406464577,
-0.6));
#82913=CARTESIAN_POINT('Ctrl Pts',(-8.14979646354914,-53.9091406464577,
-0.9));
#82914=CARTESIAN_POINT('Ctrl Pts',(-8.35272882133722,-53.5055933594704,
-0.6));
#82915=CARTESIAN_POINT('Ctrl Pts',(-8.35272882133722,-53.5055933594704,
-0.9));
#82916=CARTESIAN_POINT('Ctrl Pts',(-8.35272882133722,-52.9999999403954,
-0.6));
#82917=CARTESIAN_POINT('Ctrl Pts',(-8.35272882133722,-52.9999999403954,
-0.9));
#82918=CARTESIAN_POINT('',(-8.14979646354914,-53.9091406464577,-0.6));
#82919=CARTESIAN_POINT('Ctrl Pts',(-8.14979646354914,-53.9091406464577,
-0.6));
#82920=CARTESIAN_POINT('Ctrl Pts',(-8.35272882133722,-53.5055933594704,
-0.6));
#82921=CARTESIAN_POINT('Ctrl Pts',(-8.35272882133722,-52.9999999403954,
-0.6));
#82922=CARTESIAN_POINT('',(-8.14979646354914,-53.9091406464577,-0.9));
#82923=CARTESIAN_POINT('',(-8.14979646354914,-53.9091406464577,-0.6));
#82924=CARTESIAN_POINT('Ctrl Pts',(-8.14979646354914,-53.9091406464577,
-0.9));
#82925=CARTESIAN_POINT('Ctrl Pts',(-8.35272882133722,-53.5055933594704,
-0.9));
#82926=CARTESIAN_POINT('Ctrl Pts',(-8.35272882133722,-52.9999999403954,
-0.9));
#82927=CARTESIAN_POINT('Ctrl Pts',(-7.57114741951227,-54.5353345274925,
-0.6));
#82928=CARTESIAN_POINT('Ctrl Pts',(-7.57114741951227,-54.5353345274925,
-0.9));
#82929=CARTESIAN_POINT('Ctrl Pts',(-7.94686172157526,-54.312687933445,-0.6));
#82930=CARTESIAN_POINT('Ctrl Pts',(-7.94686172157526,-54.312687933445,-0.9));
#82931=CARTESIAN_POINT('Ctrl Pts',(-8.14979646354914,-53.9091406464577,
-0.6));
#82932=CARTESIAN_POINT('Ctrl Pts',(-8.14979646354914,-53.9091406464577,
-0.9));
#82933=CARTESIAN_POINT('',(-7.57114741951227,-54.5353345274925,-0.6));
#82934=CARTESIAN_POINT('Ctrl Pts',(-7.57114741951227,-54.5353345274925,
-0.6));
#82935=CARTESIAN_POINT('Ctrl Pts',(-7.94686172157526,-54.312687933445,-0.6));
#82936=CARTESIAN_POINT('Ctrl Pts',(-8.14979646354914,-53.9091406464577,
-0.6));
#82937=CARTESIAN_POINT('',(-7.57114741951227,-54.5353345274925,-0.9));
#82938=CARTESIAN_POINT('',(-7.57114741951227,-54.5353345274925,-0.6));
#82939=CARTESIAN_POINT('Ctrl Pts',(-7.57114741951227,-54.5353345274925,
-0.9));
#82940=CARTESIAN_POINT('Ctrl Pts',(-7.94686172157526,-54.312687933445,-0.9));
#82941=CARTESIAN_POINT('Ctrl Pts',(-8.14979646354914,-53.9091406464577,
-0.9));
#82942=CARTESIAN_POINT('Ctrl Pts',(-6.73390243202448,-54.7579811215401,
-0.6));
#82943=CARTESIAN_POINT('Ctrl Pts',(-6.73390243202448,-54.7579811215401,
-0.9));
#82944=CARTESIAN_POINT('Ctrl Pts',(-7.19543073326349,-54.7579811215401,
-0.6));
#82945=CARTESIAN_POINT('Ctrl Pts',(-7.19543073326349,-54.7579811215401,
-0.9));
#82946=CARTESIAN_POINT('Ctrl Pts',(-7.57114741951227,-54.5353345274925,
-0.6));
#82947=CARTESIAN_POINT('Ctrl Pts',(-7.57114741951227,-54.5353345274925,
-0.9));
#82948=CARTESIAN_POINT('',(-6.73390243202448,-54.7579811215401,-0.6));
#82949=CARTESIAN_POINT('Ctrl Pts',(-6.73390243202448,-54.7579811215401,
-0.6));
#82950=CARTESIAN_POINT('Ctrl Pts',(-7.19543073326349,-54.7579811215401,
-0.6));
#82951=CARTESIAN_POINT('Ctrl Pts',(-7.57114741951227,-54.5353345274925,
-0.6));
#82952=CARTESIAN_POINT('',(-6.73390243202448,-54.7579811215401,-0.9));
#82953=CARTESIAN_POINT('',(-6.73390243202448,-54.7579811215401,-0.6));
#82954=CARTESIAN_POINT('Ctrl Pts',(-6.73390243202448,-54.7579811215401,
-0.9));
#82955=CARTESIAN_POINT('Ctrl Pts',(-7.19543073326349,-54.7579811215401,
-0.9));
#82956=CARTESIAN_POINT('Ctrl Pts',(-7.57114741951227,-54.5353345274925,
-0.9));
#82957=CARTESIAN_POINT('Ctrl Pts',(-5.89897725731134,-54.5469306111336,
-0.6));
#82958=CARTESIAN_POINT('Ctrl Pts',(-5.89897725731134,-54.5469306111336,
-0.9));
#82959=CARTESIAN_POINT('Ctrl Pts',(-6.27701137214899,-54.7579811215401,
-0.6));
#82960=CARTESIAN_POINT('Ctrl Pts',(-6.27701137214899,-54.7579811215401,
-0.9));
#82961=CARTESIAN_POINT('Ctrl Pts',(-6.73390243202448,-54.7579811215401,
-0.6));
#82962=CARTESIAN_POINT('Ctrl Pts',(-6.73390243202448,-54.7579811215401,
-0.9));
#82963=CARTESIAN_POINT('',(-5.89897725731134,-54.5469306111336,-0.6));
#82964=CARTESIAN_POINT('Ctrl Pts',(-5.89897725731134,-54.5469306111336,
-0.6));
#82965=CARTESIAN_POINT('Ctrl Pts',(-6.27701137214899,-54.7579811215401,
-0.6));
#82966=CARTESIAN_POINT('Ctrl Pts',(-6.73390243202448,-54.7579811215401,
-0.6));
#82967=CARTESIAN_POINT('',(-5.89897725731134,-54.5469306111336,-0.9));
#82968=CARTESIAN_POINT('',(-5.89897725731134,-54.5469306111336,-0.6));
#82969=CARTESIAN_POINT('Ctrl Pts',(-5.89897725731134,-54.5469306111336,
-0.9));
#82970=CARTESIAN_POINT('Ctrl Pts',(-6.27701137214899,-54.7579811215401,
-0.9));
#82971=CARTESIAN_POINT('Ctrl Pts',(-6.73390243202448,-54.7579811215401,
-0.9));
#82972=CARTESIAN_POINT('Ctrl Pts',(-5.16841743141413,-54.9643931984901,
-0.6));
#82973=CARTESIAN_POINT('Ctrl Pts',(-5.16841743141413,-54.9643931984901,
-0.9));
#82974=CARTESIAN_POINT('Ctrl Pts',(-5.53485725075006,-54.8321966528893,
-0.6));
#82975=CARTESIAN_POINT('Ctrl Pts',(-5.53485725075006,-54.8321966528893,
-0.9));
#82976=CARTESIAN_POINT('Ctrl Pts',(-5.89897725731134,-54.5469306111336,
-0.6));
#82977=CARTESIAN_POINT('Ctrl Pts',(-5.89897725731134,-54.5469306111336,
-0.9));
#82978=CARTESIAN_POINT('',(-5.16841743141413,-54.9643931984901,-0.6));
#82979=CARTESIAN_POINT('Ctrl Pts',(-5.16841743141413,-54.9643931984901,
-0.6));
#82980=CARTESIAN_POINT('Ctrl Pts',(-5.53485725075006,-54.8321966528893,
-0.6));
#82981=CARTESIAN_POINT('Ctrl Pts',(-5.89897725731134,-54.5469306111336,
-0.6));
#82982=CARTESIAN_POINT('',(-5.16841743141413,-54.9643931984901,-0.9));
#82983=CARTESIAN_POINT('',(-5.16841743141413,-54.9643931984901,-0.6));
#82984=CARTESIAN_POINT('Ctrl Pts',(-5.16841743141413,-54.9643931984901,
-0.9));
#82985=CARTESIAN_POINT('Ctrl Pts',(-5.53485725075006,-54.8321966528893,
-0.9));
#82986=CARTESIAN_POINT('Ctrl Pts',(-5.89897725731134,-54.5469306111336,
-0.9));
#82987=CARTESIAN_POINT('Origin',(-5.03622148185968,-54.6512959599495,-0.6));
#82988=CARTESIAN_POINT('',(-5.03622148185968,-54.6512959599495,-0.6));
#82989=CARTESIAN_POINT('',(-4.359374539743,-53.0482293818458,-0.6));
#82990=CARTESIAN_POINT('',(-5.03622148185968,-54.6512959599495,-0.9));
#82991=CARTESIAN_POINT('',(-5.03622148185968,-54.6512959599495,-0.6));
#82992=CARTESIAN_POINT('',(-5.03622148185968,-54.6512959599495,-0.9));
#82993=CARTESIAN_POINT('Ctrl Pts',(-5.61371181160212,-54.3358801007271,
-0.6));
#82994=CARTESIAN_POINT('Ctrl Pts',(-5.61371181160212,-54.3358801007271,
-0.9));
#82995=CARTESIAN_POINT('Ctrl Pts',(-5.30061338096857,-54.55156904459,-0.6));
#82996=CARTESIAN_POINT('Ctrl Pts',(-5.30061338096857,-54.55156904459,-0.9));
#82997=CARTESIAN_POINT('Ctrl Pts',(-5.03622148185968,-54.6512959599495,
-0.6));
#82998=CARTESIAN_POINT('Ctrl Pts',(-5.03622148185968,-54.6512959599495,
-0.9));
#82999=CARTESIAN_POINT('',(-5.61371181160212,-54.3358801007271,-0.6));
#83000=CARTESIAN_POINT('Ctrl Pts',(-5.61371181160212,-54.3358801007271,
-0.6));
#83001=CARTESIAN_POINT('Ctrl Pts',(-5.30061338096857,-54.55156904459,-0.6));
#83002=CARTESIAN_POINT('Ctrl Pts',(-5.03622148185968,-54.6512959599495,
-0.6));
#83003=CARTESIAN_POINT('',(-5.61371181160212,-54.3358801007271,-0.9));
#83004=CARTESIAN_POINT('',(-5.61371181160212,-54.3358801007271,-0.6));
#83005=CARTESIAN_POINT('Ctrl Pts',(-5.61371181160212,-54.3358801007271,
-0.9));
#83006=CARTESIAN_POINT('Ctrl Pts',(-5.30061338096857,-54.55156904459,-0.9));
#83007=CARTESIAN_POINT('Ctrl Pts',(-5.03622148185968,-54.6512959599495,
-0.9));
#83008=CARTESIAN_POINT('Ctrl Pts',(-5.22871825844049,-53.7525920271873,
-0.6));
#83009=CARTESIAN_POINT('Ctrl Pts',(-5.22871825844049,-53.7525920271873,
-0.9));
#83010=CARTESIAN_POINT('Ctrl Pts',(-5.35627696663141,-54.0877215266228,
-0.6));
#83011=CARTESIAN_POINT('Ctrl Pts',(-5.35627696663141,-54.0877215266228,
-0.9));
#83012=CARTESIAN_POINT('Ctrl Pts',(-5.61371181160212,-54.3358801007271,
-0.6));
#83013=CARTESIAN_POINT('Ctrl Pts',(-5.61371181160212,-54.3358801007271,
-0.9));
#83014=CARTESIAN_POINT('',(-5.22871825844049,-53.7525920271873,-0.6));
#83015=CARTESIAN_POINT('Ctrl Pts',(-5.22871825844049,-53.7525920271873,
-0.6));
#83016=CARTESIAN_POINT('Ctrl Pts',(-5.35627696663141,-54.0877215266228,
-0.6));
#83017=CARTESIAN_POINT('Ctrl Pts',(-5.61371181160212,-54.3358801007271,
-0.6));
#83018=CARTESIAN_POINT('',(-5.22871825844049,-53.7525920271873,-0.9));
#83019=CARTESIAN_POINT('',(-5.22871825844049,-53.7525920271873,-0.6));
#83020=CARTESIAN_POINT('Ctrl Pts',(-5.22871825844049,-53.7525920271873,
-0.9));
#83021=CARTESIAN_POINT('Ctrl Pts',(-5.35627696663141,-54.0877215266228,
-0.9));
#83022=CARTESIAN_POINT('Ctrl Pts',(-5.61371181160212,-54.3358801007271,
-0.9));
#83023=CARTESIAN_POINT('Ctrl Pts',(-5.10115955024958,-52.9976807236671,
-0.6));
#83024=CARTESIAN_POINT('Ctrl Pts',(-5.10115955024958,-52.9976807236671,
-0.9));
#83025=CARTESIAN_POINT('Ctrl Pts',(-5.10115955024958,-53.4174625277519,
-0.6));
#83026=CARTESIAN_POINT('Ctrl Pts',(-5.10115955024958,-53.4174625277519,
-0.9));
#83027=CARTESIAN_POINT('Ctrl Pts',(-5.22871825844049,-53.7525920271873,
-0.6));
#83028=CARTESIAN_POINT('Ctrl Pts',(-5.22871825844049,-53.7525920271873,
-0.9));
#83029=CARTESIAN_POINT('Ctrl Pts',(-5.10115955024958,-52.9976807236671,
-0.6));
#83030=CARTESIAN_POINT('Ctrl Pts',(-5.10115955024958,-53.4174625277519,
-0.6));
#83031=CARTESIAN_POINT('Ctrl Pts',(-5.22871825844049,-53.7525920271873,
-0.6));
#83032=CARTESIAN_POINT('Ctrl Pts',(-5.10115955024958,-52.9976807236671,
-0.9));
#83033=CARTESIAN_POINT('Ctrl Pts',(-5.10115955024958,-53.4174625277519,
-0.9));
#83034=CARTESIAN_POINT('Ctrl Pts',(-5.22871825844049,-53.7525920271873,
-0.9));
#83035=CARTESIAN_POINT('Origin',(-6.69447515159845,-53.1020463705063,-0.9));
#83036=CARTESIAN_POINT('Origin',(-0.606480576097965,-54.2987720370293,-0.6));
#83037=CARTESIAN_POINT('',(-0.606480576097965,-54.2987720370293,-0.6));
#83038=CARTESIAN_POINT('',(1.48083116859198,-54.2987720370293,-0.6));
#83039=CARTESIAN_POINT('',(-0.303240288048983,-54.2987720370293,-0.6));
#83040=CARTESIAN_POINT('',(-0.606480576097965,-54.2987720370293,-0.9));
#83041=CARTESIAN_POINT('',(-0.606480576097965,-54.2987720370293,-0.6));
#83042=CARTESIAN_POINT('',(1.48083116859198,-54.2987720370293,-0.9));
#83043=CARTESIAN_POINT('',(-0.606480576097965,-54.2987720370293,-0.9));
#83044=CARTESIAN_POINT('',(1.48083116859198,-54.2987720370293,-0.6));
#83045=CARTESIAN_POINT('Origin',(-0.606480576097965,-53.1414733529091,-0.6));
#83046=CARTESIAN_POINT('',(-0.606480576097965,-53.1414733529091,-0.6));
#83047=CARTESIAN_POINT('',(-0.606480576097965,-53.0707366764545,-0.6));
#83048=CARTESIAN_POINT('',(-0.606480576097965,-53.1414733529091,-0.9));
#83049=CARTESIAN_POINT('',(-0.606480576097965,-53.1414733529091,-0.6));
#83050=CARTESIAN_POINT('',(-0.606480576097965,-53.1414733529091,-0.9));
#83051=CARTESIAN_POINT('Origin',(1.2744202837348,-53.1414733529091,-0.6));
#83052=CARTESIAN_POINT('',(1.2744202837348,-53.1414733529091,-0.6));
#83053=CARTESIAN_POINT('',(0.637210141867399,-53.1414733529091,-0.6));
#83054=CARTESIAN_POINT('',(1.2744202837348,-53.1414733529091,-0.9));
#83055=CARTESIAN_POINT('',(1.2744202837348,-53.1414733529091,-0.6));
#83056=CARTESIAN_POINT('',(1.2744202837348,-53.1414733529091,-0.9));
#83057=CARTESIAN_POINT('Origin',(1.2744202837348,-52.7425650954247,-0.6));
#83058=CARTESIAN_POINT('',(1.2744202837348,-52.7425650954247,-0.6));
#83059=CARTESIAN_POINT('',(1.2744202837348,-52.8712825477123,-0.6));
#83060=CARTESIAN_POINT('',(1.2744202837348,-52.7425650954247,-0.9));
#83061=CARTESIAN_POINT('',(1.2744202837348,-52.7425650954247,-0.6));
#83062=CARTESIAN_POINT('',(1.2744202837348,-52.7425650954247,-0.9));
#83063=CARTESIAN_POINT('Origin',(-0.606480576097965,-52.7425650954247,-0.6));
#83064=CARTESIAN_POINT('',(-0.606480576097965,-52.7425650954247,-0.6));
#83065=CARTESIAN_POINT('',(-0.303240288048983,-52.7425650954247,-0.6));
#83066=CARTESIAN_POINT('',(-0.606480576097965,-52.7425650954247,-0.9));
#83067=CARTESIAN_POINT('',(-0.606480576097965,-52.7425650954247,-0.6));
#83068=CARTESIAN_POINT('',(-0.606480576097965,-52.7425650954247,-0.9));
#83069=CARTESIAN_POINT('Origin',(-0.606480576097965,-51.7012278437614,-0.6));
#83070=CARTESIAN_POINT('',(-0.606480576097965,-51.7012278437614,-0.6));
#83071=CARTESIAN_POINT('',(-0.606480576097965,-52.3506139218807,-0.6));
#83072=CARTESIAN_POINT('',(-0.606480576097965,-51.7012278437614,-0.9));
#83073=CARTESIAN_POINT('',(-0.606480576097965,-51.7012278437614,-0.6));
#83074=CARTESIAN_POINT('',(-0.606480576097965,-51.7012278437614,-0.9));
#83075=CARTESIAN_POINT('Origin',(1.40197899192572,-51.7012278437614,-0.6));
#83076=CARTESIAN_POINT('',(1.40197899192572,-51.7012278437614,-0.6));
#83077=CARTESIAN_POINT('',(0.700989495962858,-51.7012278437614,-0.6));
#83078=CARTESIAN_POINT('',(1.40197899192572,-51.7012278437614,-0.9));
#83079=CARTESIAN_POINT('',(1.40197899192572,-51.7012278437614,-0.6));
#83080=CARTESIAN_POINT('',(1.40197899192572,-51.7012278437614,-0.9));
#83081=CARTESIAN_POINT('Origin',(1.40197899192572,-51.3000003695488,-0.6));
#83082=CARTESIAN_POINT('',(1.40197899192572,-51.3000003695488,-0.6));
#83083=CARTESIAN_POINT('',(1.40197899192572,-52.1500001847744,-0.6));
#83084=CARTESIAN_POINT('',(1.40197899192572,-51.3000003695488,-0.9));
#83085=CARTESIAN_POINT('',(1.40197899192572,-51.3000003695488,-0.6));
#83086=CARTESIAN_POINT('',(1.40197899192572,-51.3000003695488,-0.9));
#83087=CARTESIAN_POINT('Origin',(-1.05641219764948,-51.3000003695488,-0.6));
#83088=CARTESIAN_POINT('',(-1.05641219764948,-51.3000003695488,-0.6));
#83089=CARTESIAN_POINT('',(-0.528206098824739,-51.3000003695488,-0.6));
#83090=CARTESIAN_POINT('',(-1.05641219764948,-51.3000003695488,-0.9));
#83091=CARTESIAN_POINT('',(-1.05641219764948,-51.3000003695488,-0.6));
#83092=CARTESIAN_POINT('',(-1.05641219764948,-51.3000003695488,-0.9));
#83093=CARTESIAN_POINT('Origin',(-1.05641219764948,-54.7000001072884,-0.6));
#83094=CARTESIAN_POINT('',(-1.05641219764948,-54.7000001072884,-0.6));
#83095=CARTESIAN_POINT('',(-1.05641219764948,-53.8500000536442,-0.6));
#83096=CARTESIAN_POINT('',(-1.05641219764948,-54.7000001072884,-0.9));
#83097=CARTESIAN_POINT('',(-1.05641219764948,-54.7000001072884,-0.6));
#83098=CARTESIAN_POINT('',(-1.05641219764948,-54.7000001072884,-0.9));
#83099=CARTESIAN_POINT('Origin',(1.48083116859198,-54.7000001072884,-0.6));
#83100=CARTESIAN_POINT('',(1.48083116859198,-54.7000001072884,-0.6));
#83101=CARTESIAN_POINT('',(0.740415584295988,-54.7000001072884,-0.6));
#83102=CARTESIAN_POINT('',(1.48083116859198,-54.7000001072884,-0.9));
#83103=CARTESIAN_POINT('',(1.48083116859198,-54.7000001072884,-0.6));
#83104=CARTESIAN_POINT('',(1.48083116859198,-54.7000001072884,-0.9));
#83105=CARTESIAN_POINT('Origin',(1.48083116859198,-54.2987720370293,-0.6));
#83106=CARTESIAN_POINT('',(1.48083116859198,-53.6493860185146,-0.6));
#83107=CARTESIAN_POINT('',(1.48083116859198,-54.2987720370293,-0.9));
#83108=CARTESIAN_POINT('Origin',(0.212209485471249,-53.0000002384186,-0.9));
#83109=CARTESIAN_POINT('Origin',(1.88669826835394,-53.2597545981407,-0.6));
#83110=CARTESIAN_POINT('',(1.88669826835394,-53.2597545981407,-0.6));
#83111=CARTESIAN_POINT('',(3.16923525184393,-53.2597545981407,-0.6));
#83112=CARTESIAN_POINT('',(0.94334913417697,-53.2597545981407,-0.6));
#83113=CARTESIAN_POINT('',(1.88669826835394,-53.2597545981407,-0.9));
#83114=CARTESIAN_POINT('',(1.88669826835394,-53.2597545981407,-0.6));
#83115=CARTESIAN_POINT('',(3.16923525184393,-53.2597545981407,-0.9));
#83116=CARTESIAN_POINT('',(1.88669826835394,-53.2597545981407,-0.9));
#83117=CARTESIAN_POINT('',(3.16923525184393,-53.2597545981407,-0.6));
#83118=CARTESIAN_POINT('Origin',(1.88669826835394,-53.6795364022255,-0.6));
#83119=CARTESIAN_POINT('',(1.88669826835394,-53.6795364022255,-0.6));
#83120=CARTESIAN_POINT('',(1.88669826835394,-53.3397682011127,-0.6));
#83121=CARTESIAN_POINT('',(1.88669826835394,-53.6795364022255,-0.9));
#83122=CARTESIAN_POINT('',(1.88669826835394,-53.6795364022255,-0.6));
#83123=CARTESIAN_POINT('',(1.88669826835394,-53.6795364022255,-0.9));
#83124=CARTESIAN_POINT('Origin',(3.16923525184393,-53.6795364022255,-0.6));
#83125=CARTESIAN_POINT('',(3.16923525184393,-53.6795364022255,-0.6));
#83126=CARTESIAN_POINT('',(1.58461762592196,-53.6795364022255,-0.6));
#83127=CARTESIAN_POINT('',(3.16923525184393,-53.6795364022255,-0.9));
#83128=CARTESIAN_POINT('',(3.16923525184393,-53.6795364022255,-0.6));
#83129=CARTESIAN_POINT('',(3.16923525184393,-53.6795364022255,-0.9));
#83130=CARTESIAN_POINT('Origin',(3.16923525184393,-53.2597545981407,-0.6));
#83131=CARTESIAN_POINT('',(3.16923525184393,-53.1298772990704,-0.6));
#83132=CARTESIAN_POINT('',(3.16923525184393,-53.2597545981407,-0.9));
#83133=CARTESIAN_POINT('Origin',(2.52796676009893,-53.4696455001831,-0.9));
#83134=CARTESIAN_POINT('Ctrl Pts',(7.81467344611883,-54.7579811215401,-0.6));
#83135=CARTESIAN_POINT('Ctrl Pts',(7.81467344611883,-54.7579811215401,-0.9));
#83136=CARTESIAN_POINT('Ctrl Pts',(7.33458425849676,-54.7579811215401,-0.6));
#83137=CARTESIAN_POINT('Ctrl Pts',(7.33458425849676,-54.7579811215401,-0.9));
#83138=CARTESIAN_POINT('Ctrl Pts',(6.95654775947332,-54.5260576605797,-0.6));
#83139=CARTESIAN_POINT('Ctrl Pts',(6.95654775947332,-54.5260576605797,-0.9));
#83140=CARTESIAN_POINT('',(7.81467344611883,-54.7579811215401,-0.6));
#83141=CARTESIAN_POINT('',(6.95654775947332,-54.5260576605797,-0.6));
#83142=CARTESIAN_POINT('Ctrl Pts',(7.81467344611883,-54.7579811215401,-0.6));
#83143=CARTESIAN_POINT('Ctrl Pts',(7.33458425849676,-54.7579811215401,-0.6));
#83144=CARTESIAN_POINT('Ctrl Pts',(6.95654775947332,-54.5260576605797,-0.6));
#83145=CARTESIAN_POINT('',(7.81467344611883,-54.7579811215401,-0.9));
#83146=CARTESIAN_POINT('',(7.81467344611883,-54.7579811215401,-0.6));
#83147=CARTESIAN_POINT('',(6.95654775947332,-54.5260576605797,-0.9));
#83148=CARTESIAN_POINT('Ctrl Pts',(7.81467344611883,-54.7579811215401,-0.9));
#83149=CARTESIAN_POINT('Ctrl Pts',(7.33458425849676,-54.7579811215401,-0.9));
#83150=CARTESIAN_POINT('Ctrl Pts',(6.95654775947332,-54.5260576605797,-0.9));
#83151=CARTESIAN_POINT('',(6.95654775947332,-54.5260576605797,-0.6));
#83152=CARTESIAN_POINT('Ctrl Pts',(8.64031698554754,-54.5480899214745,-0.6));
#83153=CARTESIAN_POINT('Ctrl Pts',(8.64031698554754,-54.5480899214745,-0.9));
#83154=CARTESIAN_POINT('Ctrl Pts',(8.25764562934637,-54.7579811215401,-0.6));
#83155=CARTESIAN_POINT('Ctrl Pts',(8.25764562934637,-54.7579811215401,-0.9));
#83156=CARTESIAN_POINT('Ctrl Pts',(7.81467344611883,-54.7579811215401,-0.6));
#83157=CARTESIAN_POINT('Ctrl Pts',(7.81467344611883,-54.7579811215401,-0.9));
#83158=CARTESIAN_POINT('',(8.64031698554754,-54.5480899214745,-0.6));
#83159=CARTESIAN_POINT('Ctrl Pts',(8.64031698554754,-54.5480899214745,-0.6));
#83160=CARTESIAN_POINT('Ctrl Pts',(8.25764562934637,-54.7579811215401,-0.6));
#83161=CARTESIAN_POINT('Ctrl Pts',(7.81467344611883,-54.7579811215401,-0.6));
#83162=CARTESIAN_POINT('',(8.64031698554754,-54.5480899214745,-0.9));
#83163=CARTESIAN_POINT('',(8.64031698554754,-54.5480899214745,-0.6));
#83164=CARTESIAN_POINT('Ctrl Pts',(8.64031698554754,-54.5480899214745,-0.9));
#83165=CARTESIAN_POINT('Ctrl Pts',(8.25764562934637,-54.7579811215401,-0.9));
#83166=CARTESIAN_POINT('Ctrl Pts',(7.81467344611883,-54.7579811215401,-0.9));
#83167=CARTESIAN_POINT('Ctrl Pts',(9.23171903938055,-53.9300135970116,-0.6));
#83168=CARTESIAN_POINT('Ctrl Pts',(9.23171903938055,-53.9300135970116,-0.9));
#83169=CARTESIAN_POINT('Ctrl Pts',(9.02298834174871,-54.3381993174553,-0.6));
#83170=CARTESIAN_POINT('Ctrl Pts',(9.02298834174871,-54.3381993174553,-0.9));
#83171=CARTESIAN_POINT('Ctrl Pts',(8.64031698554754,-54.5480899214745,-0.6));
#83172=CARTESIAN_POINT('Ctrl Pts',(8.64031698554754,-54.5480899214745,-0.9));
#83173=CARTESIAN_POINT('',(9.23171903938055,-53.9300135970116,-0.6));
#83174=CARTESIAN_POINT('Ctrl Pts',(9.23171903938055,-53.9300135970116,-0.6));
#83175=CARTESIAN_POINT('Ctrl Pts',(9.02298834174871,-54.3381993174553,-0.6));
#83176=CARTESIAN_POINT('Ctrl Pts',(8.64031698554754,-54.5480899214745,-0.6));
#83177=CARTESIAN_POINT('',(9.23171903938055,-53.9300135970116,-0.9));
#83178=CARTESIAN_POINT('',(9.23171903938055,-53.9300135970116,-0.6));
#83179=CARTESIAN_POINT('Ctrl Pts',(9.23171903938055,-53.9300135970116,-0.9));
#83180=CARTESIAN_POINT('Ctrl Pts',(9.02298834174871,-54.3381993174553,-0.9));
#83181=CARTESIAN_POINT('Ctrl Pts',(8.64031698554754,-54.5480899214745,-0.9));
#83182=CARTESIAN_POINT('Ctrl Pts',(9.44044973701239,-53.0046383738518,-0.6));
#83183=CARTESIAN_POINT('Ctrl Pts',(9.44044973701239,-53.0046383738518,-0.9));
#83184=CARTESIAN_POINT('Ctrl Pts',(9.44044973701239,-53.5218278765678,-0.6));
#83185=CARTESIAN_POINT('Ctrl Pts',(9.44044973701239,-53.5218278765678,-0.9));
#83186=CARTESIAN_POINT('Ctrl Pts',(9.23171903938055,-53.9300135970116,-0.6));
#83187=CARTESIAN_POINT('Ctrl Pts',(9.23171903938055,-53.9300135970116,-0.9));
#83188=CARTESIAN_POINT('',(9.44044973701239,-53.0046383738518,-0.6));
#83189=CARTESIAN_POINT('Ctrl Pts',(9.44044973701239,-53.0046383738518,-0.6));
#83190=CARTESIAN_POINT('Ctrl Pts',(9.44044973701239,-53.5218278765678,-0.6));
#83191=CARTESIAN_POINT('Ctrl Pts',(9.23171903938055,-53.9300135970116,-0.6));
#83192=CARTESIAN_POINT('',(9.44044973701239,-53.0046383738518,-0.9));
#83193=CARTESIAN_POINT('',(9.44044973701239,-53.0046383738518,-0.6));
#83194=CARTESIAN_POINT('Ctrl Pts',(9.44044973701239,-53.0046383738518,-0.9));
#83195=CARTESIAN_POINT('Ctrl Pts',(9.44044973701239,-53.5218278765678,-0.9));
#83196=CARTESIAN_POINT('Ctrl Pts',(9.23171903938055,-53.9300135970116,-0.9));
#83197=CARTESIAN_POINT('Ctrl Pts',(9.2421617731452,-52.0920191407204,-0.6));
#83198=CARTESIAN_POINT('Ctrl Pts',(9.2421617731452,-52.0920191407204,-0.9));
#83199=CARTESIAN_POINT('Ctrl Pts',(9.44044973701239,-52.4944065213203,-0.6));
#83200=CARTESIAN_POINT('Ctrl Pts',(9.44044973701239,-52.4944065213203,-0.9));
#83201=CARTESIAN_POINT('Ctrl Pts',(9.44044973701239,-53.0046383738518,-0.6));
#83202=CARTESIAN_POINT('Ctrl Pts',(9.44044973701239,-53.0046383738518,-0.9));
#83203=CARTESIAN_POINT('',(9.2421617731452,-52.0920191407204,-0.6));
#83204=CARTESIAN_POINT('Ctrl Pts',(9.2421617731452,-52.0920191407204,-0.6));
#83205=CARTESIAN_POINT('Ctrl Pts',(9.44044973701239,-52.4944065213203,-0.6));
#83206=CARTESIAN_POINT('Ctrl Pts',(9.44044973701239,-53.0046383738518,-0.6));
#83207=CARTESIAN_POINT('',(9.2421617731452,-52.0920191407204,-0.9));
#83208=CARTESIAN_POINT('',(9.2421617731452,-52.0920191407204,-0.6));
#83209=CARTESIAN_POINT('Ctrl Pts',(9.2421617731452,-52.0920191407204,-0.9));
#83210=CARTESIAN_POINT('Ctrl Pts',(9.44044973701239,-52.4944065213203,-0.9));
#83211=CARTESIAN_POINT('Ctrl Pts',(9.44044973701239,-53.0046383738518,-0.9));
#83212=CARTESIAN_POINT('Ctrl Pts',(8.66582777351141,-51.4646653532982,-0.6));
#83213=CARTESIAN_POINT('Ctrl Pts',(8.66582777351141,-51.4646653532982,-0.9));
#83214=CARTESIAN_POINT('Ctrl Pts',(9.04386427253485,-51.6896311640739,-0.6));
#83215=CARTESIAN_POINT('Ctrl Pts',(9.04386427253485,-51.6896311640739,-0.9));
#83216=CARTESIAN_POINT('Ctrl Pts',(9.2421617731452,-52.0920191407204,-0.6));
#83217=CARTESIAN_POINT('Ctrl Pts',(9.2421617731452,-52.0920191407204,-0.9));
#83218=CARTESIAN_POINT('',(8.66582777351141,-51.4646653532982,-0.6));
#83219=CARTESIAN_POINT('Ctrl Pts',(8.66582777351141,-51.4646653532982,-0.6));
#83220=CARTESIAN_POINT('Ctrl Pts',(9.04386427253485,-51.6896311640739,-0.6));
#83221=CARTESIAN_POINT('Ctrl Pts',(9.2421617731452,-52.0920191407204,-0.6));
#83222=CARTESIAN_POINT('',(8.66582777351141,-51.4646653532982,-0.9));
#83223=CARTESIAN_POINT('',(8.66582777351141,-51.4646653532982,-0.6));
#83224=CARTESIAN_POINT('Ctrl Pts',(8.66582777351141,-51.4646653532982,-0.9));
#83225=CARTESIAN_POINT('Ctrl Pts',(9.04386427253485,-51.6896311640739,-0.9));
#83226=CARTESIAN_POINT('Ctrl Pts',(9.2421617731452,-52.0920191407204,-0.9));
#83227=CARTESIAN_POINT('Ctrl Pts',(7.8169908747077,-51.2396995425224,-0.6));
#83228=CARTESIAN_POINT('Ctrl Pts',(7.8169908747077,-51.2396995425224,-0.9));
#83229=CARTESIAN_POINT('Ctrl Pts',(8.28779127448797,-51.2396995425224,-0.6));
#83230=CARTESIAN_POINT('Ctrl Pts',(8.28779127448797,-51.2396995425224,-0.9));
#83231=CARTESIAN_POINT('Ctrl Pts',(8.66582777351141,-51.4646653532982,-0.6));
#83232=CARTESIAN_POINT('Ctrl Pts',(8.66582777351141,-51.4646653532982,-0.9));
#83233=CARTESIAN_POINT('',(7.8169908747077,-51.2396995425224,-0.6));
#83234=CARTESIAN_POINT('Ctrl Pts',(7.8169908747077,-51.2396995425224,-0.6));
#83235=CARTESIAN_POINT('Ctrl Pts',(8.28779127448797,-51.2396995425224,-0.6));
#83236=CARTESIAN_POINT('Ctrl Pts',(8.66582777351141,-51.4646653532982,-0.6));
#83237=CARTESIAN_POINT('',(7.8169908747077,-51.2396995425224,-0.9));
#83238=CARTESIAN_POINT('',(7.8169908747077,-51.2396995425224,-0.6));
#83239=CARTESIAN_POINT('Ctrl Pts',(7.8169908747077,-51.2396995425224,-0.9));
#83240=CARTESIAN_POINT('Ctrl Pts',(8.28779127448797,-51.2396995425224,-0.9));
#83241=CARTESIAN_POINT('Ctrl Pts',(8.66582777351141,-51.4646653532982,-0.9));
#83242=CARTESIAN_POINT('Ctrl Pts',(6.64345648139715,-51.7186216711998,-0.6));
#83243=CARTESIAN_POINT('Ctrl Pts',(6.64345648139715,-51.7186216711998,-0.9));
#83244=CARTESIAN_POINT('Ctrl Pts',(7.09802534431219,-51.2396995425224,-0.6));
#83245=CARTESIAN_POINT('Ctrl Pts',(7.09802534431219,-51.2396995425224,-0.9));
#83246=CARTESIAN_POINT('Ctrl Pts',(7.8169908747077,-51.2396995425224,-0.6));
#83247=CARTESIAN_POINT('Ctrl Pts',(7.8169908747077,-51.2396995425224,-0.9));
#83248=CARTESIAN_POINT('',(6.64345648139715,-51.7186216711998,-0.6));
#83249=CARTESIAN_POINT('Ctrl Pts',(6.64345648139715,-51.7186216711998,-0.6));
#83250=CARTESIAN_POINT('Ctrl Pts',(7.09802534431219,-51.2396995425224,-0.6));
#83251=CARTESIAN_POINT('Ctrl Pts',(7.8169908747077,-51.2396995425224,-0.6));
#83252=CARTESIAN_POINT('',(6.64345648139715,-51.7186216711998,-0.9));
#83253=CARTESIAN_POINT('',(6.64345648139715,-51.7186216711998,-0.6));
#83254=CARTESIAN_POINT('Ctrl Pts',(6.64345648139715,-51.7186216711998,-0.9));
#83255=CARTESIAN_POINT('Ctrl Pts',(7.09802534431219,-51.2396995425224,-0.9));
#83256=CARTESIAN_POINT('Ctrl Pts',(7.8169908747077,-51.2396995425224,-0.9));
#83257=CARTESIAN_POINT('Ctrl Pts',(6.18888761848211,-53.0440656542778,-0.6));
#83258=CARTESIAN_POINT('Ctrl Pts',(6.18888761848211,-53.0440656542778,-0.9));
#83259=CARTESIAN_POINT('Ctrl Pts',(6.18888761848211,-52.1975443959236,-0.6));
#83260=CARTESIAN_POINT('Ctrl Pts',(6.18888761848211,-52.1975443959236,-0.9));
#83261=CARTESIAN_POINT('Ctrl Pts',(6.64345648139715,-51.7186216711998,-0.6));
#83262=CARTESIAN_POINT('Ctrl Pts',(6.64345648139715,-51.7186216711998,-0.9));
#83263=CARTESIAN_POINT('',(6.18888761848211,-53.0440656542778,-0.6));
#83264=CARTESIAN_POINT('Ctrl Pts',(6.18888761848211,-53.0440656542778,-0.6));
#83265=CARTESIAN_POINT('Ctrl Pts',(6.18888761848211,-52.1975443959236,-0.6));
#83266=CARTESIAN_POINT('Ctrl Pts',(6.64345648139715,-51.7186216711998,-0.6));
#83267=CARTESIAN_POINT('',(6.18888761848211,-53.0440656542778,-0.9));
#83268=CARTESIAN_POINT('',(6.18888761848211,-53.0440656542778,-0.6));
#83269=CARTESIAN_POINT('Ctrl Pts',(6.18888761848211,-53.0440656542778,-0.9));
#83270=CARTESIAN_POINT('Ctrl Pts',(6.18888761848211,-52.1975443959236,-0.9));
#83271=CARTESIAN_POINT('Ctrl Pts',(6.64345648139715,-51.7186216711998,-0.9));
#83272=CARTESIAN_POINT('Ctrl Pts',(6.38370420783758,-53.8929061293602,-0.6));
#83273=CARTESIAN_POINT('Ctrl Pts',(6.38370420783758,-53.8929061293602,-0.9));
#83274=CARTESIAN_POINT('Ctrl Pts',(6.18888761848211,-53.4916780591011,-0.6));
#83275=CARTESIAN_POINT('Ctrl Pts',(6.18888761848211,-53.4916780591011,-0.9));
#83276=CARTESIAN_POINT('Ctrl Pts',(6.18888761848211,-53.0440656542778,-0.6));
#83277=CARTESIAN_POINT('Ctrl Pts',(6.18888761848211,-53.0440656542778,-0.9));
#83278=CARTESIAN_POINT('',(6.38370420783758,-53.8929061293602,-0.6));
#83279=CARTESIAN_POINT('Ctrl Pts',(6.38370420783758,-53.8929061293602,-0.6));
#83280=CARTESIAN_POINT('Ctrl Pts',(6.18888761848211,-53.4916780591011,-0.6));
#83281=CARTESIAN_POINT('Ctrl Pts',(6.18888761848211,-53.0440656542778,-0.6));
#83282=CARTESIAN_POINT('',(6.38370420783758,-53.8929061293602,-0.9));
#83283=CARTESIAN_POINT('',(6.38370420783758,-53.8929061293602,-0.6));
#83284=CARTESIAN_POINT('Ctrl Pts',(6.38370420783758,-53.8929061293602,-0.9));
#83285=CARTESIAN_POINT('Ctrl Pts',(6.18888761848211,-53.4916780591011,-0.9));
#83286=CARTESIAN_POINT('Ctrl Pts',(6.18888761848211,-53.0440656542778,-0.9));
#83287=CARTESIAN_POINT('Ctrl Pts',(6.95654775947332,-54.5260576605797,-0.6));
#83288=CARTESIAN_POINT('Ctrl Pts',(6.95654775947332,-54.5260576605797,-0.9));
#83289=CARTESIAN_POINT('Ctrl Pts',(6.57852079719305,-54.2941336035728,-0.6));
#83290=CARTESIAN_POINT('Ctrl Pts',(6.57852079719305,-54.2941336035728,-0.9));
#83291=CARTESIAN_POINT('Ctrl Pts',(6.38370420783758,-53.8929061293602,-0.6));
#83292=CARTESIAN_POINT('Ctrl Pts',(6.38370420783758,-53.8929061293602,-0.9));
#83293=CARTESIAN_POINT('Ctrl Pts',(6.95654775947332,-54.5260576605797,-0.6));
#83294=CARTESIAN_POINT('Ctrl Pts',(6.57852079719305,-54.2941336035728,-0.6));
#83295=CARTESIAN_POINT('Ctrl Pts',(6.38370420783758,-53.8929061293602,-0.6));
#83296=CARTESIAN_POINT('Ctrl Pts',(6.95654775947332,-54.5260576605797,-0.9));
#83297=CARTESIAN_POINT('Ctrl Pts',(6.57852079719305,-54.2941336035728,-0.9));
#83298=CARTESIAN_POINT('Ctrl Pts',(6.38370420783758,-53.8929061293602,-0.9));
#83299=CARTESIAN_POINT('Origin',(7.81466867774725,-52.9988403320313,-0.9));
#83300=CARTESIAN_POINT('Origin',(14.4384088739753,-52.9791269898415,-0.6));
#83301=CARTESIAN_POINT('',(14.4384088739753,-52.9791269898415,-0.6));
#83302=CARTESIAN_POINT('',(13.8817873224616,-53.5218278765678,-0.6));
#83303=CARTESIAN_POINT('',(10.7321883094972,-56.5926579091458,-0.6));
#83304=CARTESIAN_POINT('',(14.4384088739753,-52.9791269898415,-0.9));
#83305=CARTESIAN_POINT('',(14.4384088739753,-52.9791269898415,-0.6));
#83306=CARTESIAN_POINT('',(13.8817873224616,-53.5218278765678,-0.9));
#83307=CARTESIAN_POINT('',(14.4384088739753,-52.9791269898415,-0.9));
#83308=CARTESIAN_POINT('',(13.8817873224616,-53.5218278765678,-0.6));
#83309=CARTESIAN_POINT('Origin',(15.649041198194,-54.7000001072884,-0.6));
#83310=CARTESIAN_POINT('',(15.649041198194,-54.7000001072884,-0.6));
#83311=CARTESIAN_POINT('',(12.6586197719514,-50.4492166618859,-0.6));
#83312=CARTESIAN_POINT('',(15.649041198194,-54.7000001072884,-0.9));
#83313=CARTESIAN_POINT('',(15.649041198194,-54.7000001072884,-0.6));
#83314=CARTESIAN_POINT('',(15.649041198194,-54.7000001072884,-0.9));
#83315=CARTESIAN_POINT('Origin',(16.2427702173591,-54.7000001072884,-0.6));
#83316=CARTESIAN_POINT('',(16.2427702173591,-54.7000001072884,-0.6));
#83317=CARTESIAN_POINT('',(8.12138510867953,-54.7000001072884,-0.6));
#83318=CARTESIAN_POINT('',(16.2427702173591,-54.7000001072884,-0.9));
#83319=CARTESIAN_POINT('',(16.2427702173591,-54.7000001072884,-0.6));
#83320=CARTESIAN_POINT('',(16.2427702173591,-54.7000001072884,-0.9));
#83321=CARTESIAN_POINT('Origin',(14.7538175806403,-52.6776264309883,-0.6));
#83322=CARTESIAN_POINT('',(14.7538175806403,-52.6776264309883,-0.6));
#83323=CARTESIAN_POINT('',(12.2377001613175,-49.2601035965936,-0.6));
#83324=CARTESIAN_POINT('',(14.7538175806403,-52.6776264309883,-0.9));
#83325=CARTESIAN_POINT('',(14.7538175806403,-52.6776264309883,-0.6));
#83326=CARTESIAN_POINT('',(14.7538175806403,-52.6776264309883,-0.9));
#83327=CARTESIAN_POINT('Origin',(16.1801519617438,-51.3000003695488,-0.6));
#83328=CARTESIAN_POINT('',(16.1801519617438,-51.3000003695488,-0.6));
#83329=CARTESIAN_POINT('',(11.569878082483,-55.7528366263105,-0.6));
#83330=CARTESIAN_POINT('',(16.1801519617438,-51.3000003695488,-0.9));
#83331=CARTESIAN_POINT('',(16.1801519617438,-51.3000003695488,-0.6));
#83332=CARTESIAN_POINT('',(16.1801519617438,-51.3000003695488,-0.9));
#83333=CARTESIAN_POINT('Origin',(15.5701914057136,-51.3000003695488,-0.6));
#83334=CARTESIAN_POINT('',(15.5701914057136,-51.3000003695488,-0.6));
#83335=CARTESIAN_POINT('',(7.78509570285678,-51.3000003695488,-0.6));
#83336=CARTESIAN_POINT('',(15.5701914057136,-51.3000003695488,-0.9));
#83337=CARTESIAN_POINT('',(15.5701914057136,-51.3000003695488,-0.6));
#83338=CARTESIAN_POINT('',(15.5701914057136,-51.3000003695488,-0.9));
#83339=CARTESIAN_POINT('Origin',(13.8817873224616,-52.9860846400261,-0.6));
#83340=CARTESIAN_POINT('',(13.8817873224616,-52.9860846400261,-0.6));
#83341=CARTESIAN_POINT('',(10.4030900973563,-56.4600022473006,-0.6));
#83342=CARTESIAN_POINT('',(13.8817873224616,-52.9860846400261,-0.9));
#83343=CARTESIAN_POINT('',(13.8817873224616,-52.9860846400261,-0.6));
#83344=CARTESIAN_POINT('',(13.8817873224616,-52.9860846400261,-0.9));
#83345=CARTESIAN_POINT('Origin',(13.8817873224616,-51.3000003695488,-0.6));
#83346=CARTESIAN_POINT('',(13.8817873224616,-51.3000003695488,-0.6));
#83347=CARTESIAN_POINT('',(13.8817873224616,-52.1500001847744,-0.6));
#83348=CARTESIAN_POINT('',(13.8817873224616,-51.3000003695488,-0.9));
#83349=CARTESIAN_POINT('',(13.8817873224616,-51.3000003695488,-0.6));
#83350=CARTESIAN_POINT('',(13.8817873224616,-51.3000003695488,-0.9));
#83351=CARTESIAN_POINT('Origin',(13.4318533167243,-51.3000003695488,-0.6));
#83352=CARTESIAN_POINT('',(13.4318533167243,-51.3000003695488,-0.6));
#83353=CARTESIAN_POINT('',(6.71592665836215,-51.3000003695488,-0.6));
#83354=CARTESIAN_POINT('',(13.4318533167243,-51.3000003695488,-0.9));
#83355=CARTESIAN_POINT('',(13.4318533167243,-51.3000003695488,-0.6));
#83356=CARTESIAN_POINT('',(13.4318533167243,-51.3000003695488,-0.9));
#83357=CARTESIAN_POINT('Origin',(13.4318533167243,-54.7000001072884,-0.6));
#83358=CARTESIAN_POINT('',(13.4318533167243,-54.7000001072884,-0.6));
#83359=CARTESIAN_POINT('',(13.4318533167243,-53.8500000536442,-0.6));
#83360=CARTESIAN_POINT('',(13.4318533167243,-54.7000001072884,-0.9));
#83361=CARTESIAN_POINT('',(13.4318533167243,-54.7000001072884,-0.6));
#83362=CARTESIAN_POINT('',(13.4318533167243,-54.7000001072884,-0.9));
#83363=CARTESIAN_POINT('Origin',(13.8817873224616,-54.7000001072884,-0.6));
#83364=CARTESIAN_POINT('',(13.8817873224616,-54.7000001072884,-0.6));
#83365=CARTESIAN_POINT('',(6.9408936612308,-54.7000001072884,-0.6));
#83366=CARTESIAN_POINT('',(13.8817873224616,-54.7000001072884,-0.9));
#83367=CARTESIAN_POINT('',(13.8817873224616,-54.7000001072884,-0.6));
#83368=CARTESIAN_POINT('',(13.8817873224616,-54.7000001072884,-0.9));
#83369=CARTESIAN_POINT('Origin',(13.8817873224616,-53.5218278765678,-0.6));
#83370=CARTESIAN_POINT('',(13.8817873224616,-53.2609139382839,-0.6));
#83371=CARTESIAN_POINT('',(13.8817873224616,-53.5218278765678,-0.9));
#83372=CARTESIAN_POINT('Origin',(14.8373117670417,-53.0000002384186,-0.9));
#83373=CARTESIAN_POINT('Origin',(21.5375890955329,-54.2987720370293,-0.6));
#83374=CARTESIAN_POINT('',(21.5375890955329,-54.2987720370293,-0.6));
#83375=CARTESIAN_POINT('',(23.2120695337653,-54.2987720370293,-0.6));
#83376=CARTESIAN_POINT('',(10.7687945477664,-54.2987720370293,-0.6));
#83377=CARTESIAN_POINT('',(21.5375890955329,-54.2987720370293,-0.9));
#83378=CARTESIAN_POINT('',(21.5375890955329,-54.2987720370293,-0.6));
#83379=CARTESIAN_POINT('',(23.2120695337653,-54.2987720370293,-0.9));
#83380=CARTESIAN_POINT('',(21.5375890955329,-54.2987720370293,-0.9));
#83381=CARTESIAN_POINT('',(23.2120695337653,-54.2987720370293,-0.6));
#83382=CARTESIAN_POINT('Origin',(21.5375890955329,-51.3000003695488,-0.6));
#83383=CARTESIAN_POINT('',(21.5375890955329,-51.3000003695488,-0.6));
#83384=CARTESIAN_POINT('',(21.5375890955329,-52.1500001847744,-0.6));
#83385=CARTESIAN_POINT('',(21.5375890955329,-51.3000003695488,-0.9));
#83386=CARTESIAN_POINT('',(21.5375890955329,-51.3000003695488,-0.6));
#83387=CARTESIAN_POINT('',(21.5375890955329,-51.3000003695488,-0.9));
#83388=CARTESIAN_POINT('Origin',(21.0876550897956,-51.3000003695488,-0.6));
#83389=CARTESIAN_POINT('',(21.0876550897956,-51.3000003695488,-0.6));
#83390=CARTESIAN_POINT('',(10.5438275448978,-51.3000003695488,-0.6));
#83391=CARTESIAN_POINT('',(21.0876550897956,-51.3000003695488,-0.9));
#83392=CARTESIAN_POINT('',(21.0876550897956,-51.3000003695488,-0.6));
#83393=CARTESIAN_POINT('',(21.0876550897956,-51.3000003695488,-0.9));
#83394=CARTESIAN_POINT('Origin',(21.0876550897956,-54.7000001072884,-0.6));
#83395=CARTESIAN_POINT('',(21.0876550897956,-54.7000001072884,-0.6));
#83396=CARTESIAN_POINT('',(21.0876550897956,-53.8500000536442,-0.6));
#83397=CARTESIAN_POINT('',(21.0876550897956,-54.7000001072884,-0.9));
#83398=CARTESIAN_POINT('',(21.0876550897956,-54.7000001072884,-0.6));
#83399=CARTESIAN_POINT('',(21.0876550897956,-54.7000001072884,-0.9));
#83400=CARTESIAN_POINT('Origin',(23.2120695337653,-54.7000001072884,-0.6));
#83401=CARTESIAN_POINT('',(23.2120695337653,-54.7000001072884,-0.6));
#83402=CARTESIAN_POINT('',(11.6060347668827,-54.7000001072884,-0.6));
#83403=CARTESIAN_POINT('',(23.2120695337653,-54.7000001072884,-0.9));
#83404=CARTESIAN_POINT('',(23.2120695337653,-54.7000001072884,-0.6));
#83405=CARTESIAN_POINT('',(23.2120695337653,-54.7000001072884,-0.9));
#83406=CARTESIAN_POINT('Origin',(23.2120695337653,-54.2987720370293,-0.6));
#83407=CARTESIAN_POINT('',(23.2120695337653,-53.6493860185146,-0.6));
#83408=CARTESIAN_POINT('',(23.2120695337653,-54.2987720370293,-0.9));
#83409=CARTESIAN_POINT('Origin',(22.1498623117805,-53.0000002384186,-0.9));
#83410=CARTESIAN_POINT('Ctrl Pts',(27.2463884577155,-54.4715551733971,-0.6));
#83411=CARTESIAN_POINT('Ctrl Pts',(27.2463884577155,-54.4715551733971,-0.9));
#83412=CARTESIAN_POINT('Ctrl Pts',(27.0782461389899,-54.5840380787849,-0.6));
#83413=CARTESIAN_POINT('Ctrl Pts',(27.0782461389899,-54.5840380787849,-0.9));
#83414=CARTESIAN_POINT('Ctrl Pts',(26.8405237421393,-54.6420190930367,-0.6));
#83415=CARTESIAN_POINT('Ctrl Pts',(26.8405237421393,-54.6420190930367,-0.9));
#83416=CARTESIAN_POINT('',(27.2463884577155,-54.4715551733971,-0.6));
#83417=CARTESIAN_POINT('',(26.8405237421393,-54.6420190930367,-0.6));
#83418=CARTESIAN_POINT('Ctrl Pts',(27.2463884577155,-54.4715551733971,-0.6));
#83419=CARTESIAN_POINT('Ctrl Pts',(27.0782461389899,-54.5840380787849,-0.6));
#83420=CARTESIAN_POINT('Ctrl Pts',(26.8405237421393,-54.6420190930367,-0.6));
#83421=CARTESIAN_POINT('',(27.2463884577155,-54.4715551733971,-0.9));
#83422=CARTESIAN_POINT('',(27.2463884577155,-54.4715551733971,-0.6));
#83423=CARTESIAN_POINT('',(26.8405237421393,-54.6420190930367,-0.9));
#83424=CARTESIAN_POINT('Ctrl Pts',(27.2463884577155,-54.4715551733971,-0.9));
#83425=CARTESIAN_POINT('Ctrl Pts',(27.0782461389899,-54.5840380787849,-0.9));
#83426=CARTESIAN_POINT('Ctrl Pts',(26.8405237421393,-54.6420190930367,-0.9));
#83427=CARTESIAN_POINT('',(26.8405237421393,-54.6420190930367,-0.6));
#83428=CARTESIAN_POINT('Ctrl Pts',(27.55600836128,-54.1630969643593,-0.6));
#83429=CARTESIAN_POINT('Ctrl Pts',(27.55600836128,-54.1630969643593,-0.9));
#83430=CARTESIAN_POINT('Ctrl Pts',(27.4145307764411,-54.3590722680092,-0.6));
#83431=CARTESIAN_POINT('Ctrl Pts',(27.4145307764411,-54.3590722680092,-0.9));
#83432=CARTESIAN_POINT('Ctrl Pts',(27.2463884577155,-54.4715551733971,-0.6));
#83433=CARTESIAN_POINT('Ctrl Pts',(27.2463884577155,-54.4715551733971,-0.9));
#83434=CARTESIAN_POINT('',(27.55600836128,-54.1630969643593,-0.6));
#83435=CARTESIAN_POINT('Ctrl Pts',(27.55600836128,-54.1630969643593,-0.6));
#83436=CARTESIAN_POINT('Ctrl Pts',(27.4145307764411,-54.3590722680092,-0.6));
#83437=CARTESIAN_POINT('Ctrl Pts',(27.2463884577155,-54.4715551733971,-0.6));
#83438=CARTESIAN_POINT('',(27.55600836128,-54.1630969643593,-0.9));
#83439=CARTESIAN_POINT('',(27.55600836128,-54.1630969643593,-0.6));
#83440=CARTESIAN_POINT('Ctrl Pts',(27.55600836128,-54.1630969643593,-0.9));
#83441=CARTESIAN_POINT('Ctrl Pts',(27.4145307764411,-54.3590722680092,-0.9));
#83442=CARTESIAN_POINT('Ctrl Pts',(27.2463884577155,-54.4715551733971,-0.9));
#83443=CARTESIAN_POINT('Ctrl Pts',(27.7879324182868,-53.6679403185844,-0.6));
#83444=CARTESIAN_POINT('Ctrl Pts',(27.7879324182868,-53.6679403185844,-0.9));
#83445=CARTESIAN_POINT('Ctrl Pts',(27.6974764093757,-53.9671216607094,-0.6));
#83446=CARTESIAN_POINT('Ctrl Pts',(27.6974764093757,-53.9671216607094,-0.9));
#83447=CARTESIAN_POINT('Ctrl Pts',(27.55600836128,-54.1630969643593,-0.6));
#83448=CARTESIAN_POINT('Ctrl Pts',(27.55600836128,-54.1630969643593,-0.9));
#83449=CARTESIAN_POINT('',(27.7879324182868,-53.6679403185844,-0.6));
#83450=CARTESIAN_POINT('Ctrl Pts',(27.7879324182868,-53.6679403185844,-0.6));
#83451=CARTESIAN_POINT('Ctrl Pts',(27.6974764093757,-53.9671216607094,-0.6));
#83452=CARTESIAN_POINT('Ctrl Pts',(27.55600836128,-54.1630969643593,-0.6));
#83453=CARTESIAN_POINT('',(27.7879324182868,-53.6679403185844,-0.9));
#83454=CARTESIAN_POINT('',(27.7879324182868,-53.6679403185844,-0.6));
#83455=CARTESIAN_POINT('Ctrl Pts',(27.7879324182868,-53.6679403185844,-0.9));
#83456=CARTESIAN_POINT('Ctrl Pts',(27.6974764093757,-53.9671216607094,-0.9));
#83457=CARTESIAN_POINT('Ctrl Pts',(27.55600836128,-54.1630969643593,-0.9));
#83458=CARTESIAN_POINT('Ctrl Pts',(27.8783788904548,-52.9814462065697,-0.6));
#83459=CARTESIAN_POINT('Ctrl Pts',(27.8783788904548,-52.9814462065697,-0.9));
#83460=CARTESIAN_POINT('Ctrl Pts',(27.8783788904548,-53.3687583804131,-0.6));
#83461=CARTESIAN_POINT('Ctrl Pts',(27.8783788904548,-53.3687583804131,-0.9));
#83462=CARTESIAN_POINT('Ctrl Pts',(27.7879324182868,-53.6679403185844,-0.6));
#83463=CARTESIAN_POINT('Ctrl Pts',(27.7879324182868,-53.6679403185844,-0.9));
#83464=CARTESIAN_POINT('',(27.8783788904548,-52.9814462065697,-0.6));
#83465=CARTESIAN_POINT('Ctrl Pts',(27.8783788904548,-52.9814462065697,-0.6));
#83466=CARTESIAN_POINT('Ctrl Pts',(27.8783788904548,-53.3687583804131,-0.6));
#83467=CARTESIAN_POINT('Ctrl Pts',(27.7879324182868,-53.6679403185844,-0.6));
#83468=CARTESIAN_POINT('',(27.8783788904548,-52.9814462065697,-0.9));
#83469=CARTESIAN_POINT('',(27.8783788904548,-52.9814462065697,-0.6));
#83470=CARTESIAN_POINT('Ctrl Pts',(27.8783788904548,-52.9814462065697,-0.9));
#83471=CARTESIAN_POINT('Ctrl Pts',(27.8783788904548,-53.3687583804131,-0.9));
#83472=CARTESIAN_POINT('Ctrl Pts',(27.7879324182868,-53.6679403185844,-0.9));
#83473=CARTESIAN_POINT('Ctrl Pts',(27.7450266107917,-52.1731923222542,-0.6));
#83474=CARTESIAN_POINT('Ctrl Pts',(27.7450266107917,-52.1731923222542,-0.9));
#83475=CARTESIAN_POINT('Ctrl Pts',(27.8783788904548,-52.5268761515617,-0.6));
#83476=CARTESIAN_POINT('Ctrl Pts',(27.8783788904548,-52.5268761515617,-0.9));
#83477=CARTESIAN_POINT('Ctrl Pts',(27.8783788904548,-52.9814462065697,-0.6));
#83478=CARTESIAN_POINT('Ctrl Pts',(27.8783788904548,-52.9814462065697,-0.9));
#83479=CARTESIAN_POINT('',(27.7450266107917,-52.1731923222542,-0.6));
#83480=CARTESIAN_POINT('Ctrl Pts',(27.7450266107917,-52.1731923222542,-0.6));
#83481=CARTESIAN_POINT('Ctrl Pts',(27.8783788904548,-52.5268761515617,-0.6));
#83482=CARTESIAN_POINT('Ctrl Pts',(27.8783788904548,-52.9814462065697,-0.6));
#83483=CARTESIAN_POINT('',(27.7450266107917,-52.1731923222542,-0.9));
#83484=CARTESIAN_POINT('',(27.7450266107917,-52.1731923222542,-0.6));
#83485=CARTESIAN_POINT('Ctrl Pts',(27.7450266107917,-52.1731923222542,-0.9));
#83486=CARTESIAN_POINT('Ctrl Pts',(27.8783788904548,-52.5268761515617,-0.9));
#83487=CARTESIAN_POINT('Ctrl Pts',(27.8783788904548,-52.9814462065697,-0.9));
#83488=CARTESIAN_POINT('Ctrl Pts',(27.3426332697272,-51.5922240614891,-0.6));
#83489=CARTESIAN_POINT('Ctrl Pts',(27.3426332697272,-51.5922240614891,-0.9));
#83490=CARTESIAN_POINT('Ctrl Pts',(27.6116647943854,-51.8195084929466,-0.6));
#83491=CARTESIAN_POINT('Ctrl Pts',(27.6116647943854,-51.8195084929466,-0.9));
#83492=CARTESIAN_POINT('Ctrl Pts',(27.7450266107917,-52.1731923222542,-0.6));
#83493=CARTESIAN_POINT('Ctrl Pts',(27.7450266107917,-52.1731923222542,-0.9));
#83494=CARTESIAN_POINT('',(27.3426332697272,-51.5922240614891,-0.6));
#83495=CARTESIAN_POINT('Ctrl Pts',(27.3426332697272,-51.5922240614891,-0.6));
#83496=CARTESIAN_POINT('Ctrl Pts',(27.6116647943854,-51.8195084929466,-0.6));
#83497=CARTESIAN_POINT('Ctrl Pts',(27.7450266107917,-52.1731923222542,-0.6));
#83498=CARTESIAN_POINT('',(27.3426332697272,-51.5922240614891,-0.9));
#83499=CARTESIAN_POINT('',(27.3426332697272,-51.5922240614891,-0.6));
#83500=CARTESIAN_POINT('Ctrl Pts',(27.3426332697272,-51.5922240614891,-0.9));
#83501=CARTESIAN_POINT('Ctrl Pts',(27.6116647943854,-51.8195084929466,-0.9));
#83502=CARTESIAN_POINT('Ctrl Pts',(27.7450266107917,-52.1731923222542,-0.9));
#83503=CARTESIAN_POINT('Ctrl Pts',(26.8439951166511,-51.3487039208412,-0.6));
#83504=CARTESIAN_POINT('Ctrl Pts',(26.8439951166511,-51.3487039208412,-0.9));
#83505=CARTESIAN_POINT('Ctrl Pts',(27.1362200006843,-51.4159618020058,-0.6));
#83506=CARTESIAN_POINT('Ctrl Pts',(27.1362200006843,-51.4159618020058,-0.9));
#83507=CARTESIAN_POINT('Ctrl Pts',(27.3426332697272,-51.5922240614891,-0.6));
#83508=CARTESIAN_POINT('Ctrl Pts',(27.3426332697272,-51.5922240614891,-0.9));
#83509=CARTESIAN_POINT('',(26.8439951166511,-51.3487039208412,-0.6));
#83510=CARTESIAN_POINT('Ctrl Pts',(26.8439951166511,-51.3487039208412,-0.6));
#83511=CARTESIAN_POINT('Ctrl Pts',(27.1362200006843,-51.4159618020058,-0.6));
#83512=CARTESIAN_POINT('Ctrl Pts',(27.3426332697272,-51.5922240614891,-0.6));
#83513=CARTESIAN_POINT('',(26.8439951166511,-51.3487039208412,-0.9));
#83514=CARTESIAN_POINT('',(26.8439951166511,-51.3487039208412,-0.6));
#83515=CARTESIAN_POINT('Ctrl Pts',(26.8439951166511,-51.3487039208412,-0.9));
#83516=CARTESIAN_POINT('Ctrl Pts',(27.1362200006843,-51.4159618020058,-0.9));
#83517=CARTESIAN_POINT('Ctrl Pts',(27.3426332697272,-51.5922240614891,-0.9));
#83518=CARTESIAN_POINT('Ctrl Pts',(26.2386789545417,-51.3000003695488,-0.6));
#83519=CARTESIAN_POINT('Ctrl Pts',(26.2386789545417,-51.3000003695488,-0.9));
#83520=CARTESIAN_POINT('Ctrl Pts',(26.6352644190192,-51.3000003695488,-0.6));
#83521=CARTESIAN_POINT('Ctrl Pts',(26.6352644190192,-51.3000003695488,-0.9));
#83522=CARTESIAN_POINT('Ctrl Pts',(26.8439951166511,-51.3487039208412,-0.6));
#83523=CARTESIAN_POINT('Ctrl Pts',(26.8439951166511,-51.3487039208412,-0.9));
#83524=CARTESIAN_POINT('',(26.2386789545417,-51.3000003695488,-0.6));
#83525=CARTESIAN_POINT('Ctrl Pts',(26.2386789545417,-51.3000003695488,-0.6));
#83526=CARTESIAN_POINT('Ctrl Pts',(26.6352644190192,-51.3000003695488,-0.6));
#83527=CARTESIAN_POINT('Ctrl Pts',(26.8439951166511,-51.3487039208412,-0.6));
#83528=CARTESIAN_POINT('',(26.2386789545417,-51.3000003695488,-0.9));
#83529=CARTESIAN_POINT('',(26.2386789545417,-51.3000003695488,-0.6));
#83530=CARTESIAN_POINT('Ctrl Pts',(26.2386789545417,-51.3000003695488,-0.9));
#83531=CARTESIAN_POINT('Ctrl Pts',(26.6352644190192,-51.3000003695488,-0.9));
#83532=CARTESIAN_POINT('Ctrl Pts',(26.8439951166511,-51.3487039208412,-0.9));
#83533=CARTESIAN_POINT('Origin',(25.06746198982,-51.3000003695488,-0.6));
#83534=CARTESIAN_POINT('',(25.06746198982,-51.3000003695488,-0.6));
#83535=CARTESIAN_POINT('',(12.53373099491,-51.3000003695488,-0.6));
#83536=CARTESIAN_POINT('',(25.06746198982,-51.3000003695488,-0.9));
#83537=CARTESIAN_POINT('',(25.06746198982,-51.3000003695488,-0.6));
#83538=CARTESIAN_POINT('',(25.06746198982,-51.3000003695488,-0.9));
#83539=CARTESIAN_POINT('Origin',(25.06746198982,-54.7000001072884,-0.6));
#83540=CARTESIAN_POINT('',(25.06746198982,-54.7000001072884,-0.6));
#83541=CARTESIAN_POINT('',(25.06746198982,-53.8500000536442,-0.6));
#83542=CARTESIAN_POINT('',(25.06746198982,-54.7000001072884,-0.9));
#83543=CARTESIAN_POINT('',(25.06746198982,-54.7000001072884,-0.6));
#83544=CARTESIAN_POINT('',(25.06746198982,-54.7000001072884,-0.9));
#83545=CARTESIAN_POINT('Origin',(26.2943449243903,-54.7000001072884,-0.6));
#83546=CARTESIAN_POINT('',(26.2943449243903,-54.7000001072884,-0.6));
#83547=CARTESIAN_POINT('',(13.1471724621952,-54.7000001072884,-0.6));
#83548=CARTESIAN_POINT('',(26.2943449243903,-54.7000001072884,-0.9));
#83549=CARTESIAN_POINT('',(26.2943449243903,-54.7000001072884,-0.6));
#83550=CARTESIAN_POINT('',(26.2943449243903,-54.7000001072884,-0.9));
#83551=CARTESIAN_POINT('Ctrl Pts',(26.8405237421393,-54.6420190930367,-0.6));
#83552=CARTESIAN_POINT('Ctrl Pts',(26.8405237421393,-54.6420190930367,-0.9));
#83553=CARTESIAN_POINT('Ctrl Pts',(26.6028013452888,-54.7000001072884,-0.6));
#83554=CARTESIAN_POINT('Ctrl Pts',(26.6028013452888,-54.7000001072884,-0.9));
#83555=CARTESIAN_POINT('Ctrl Pts',(26.2943449243903,-54.7000001072884,-0.6));
#83556=CARTESIAN_POINT('Ctrl Pts',(26.2943449243903,-54.7000001072884,-0.9));
#83557=CARTESIAN_POINT('Ctrl Pts',(26.8405237421393,-54.6420190930367,-0.6));
#83558=CARTESIAN_POINT('Ctrl Pts',(26.6028013452888,-54.7000001072884,-0.6));
#83559=CARTESIAN_POINT('Ctrl Pts',(26.2943449243903,-54.7000001072884,-0.6));
#83560=CARTESIAN_POINT('Ctrl Pts',(26.8405237421393,-54.6420190930367,-0.9));
#83561=CARTESIAN_POINT('Ctrl Pts',(26.6028013452888,-54.7000001072884,-0.9));
#83562=CARTESIAN_POINT('Ctrl Pts',(26.2943449243903,-54.7000001072884,-0.9));
#83563=CARTESIAN_POINT('Origin',(26.4729204401374,-53.0000002384186,-0.9));
#83564=CARTESIAN_POINT('Origin',(32.6444044336677,-53.190177500248,-0.6));
#83565=CARTESIAN_POINT('',(32.6444044336677,-53.190177500248,-0.6));
#83566=CARTESIAN_POINT('',(32.1225824579597,-53.190177500248,-0.6));
#83567=CARTESIAN_POINT('',(16.3222022168338,-53.190177500248,-0.6));
#83568=CARTESIAN_POINT('',(32.6444044336677,-53.190177500248,-0.9));
#83569=CARTESIAN_POINT('',(32.6444044336677,-53.190177500248,-0.6));
#83570=CARTESIAN_POINT('',(32.1225824579597,-53.190177500248,-0.9));
#83571=CARTESIAN_POINT('',(32.6444044336677,-53.190177500248,-0.9));
#83572=CARTESIAN_POINT('',(32.1225824579597,-53.190177500248,-0.6));
#83573=CARTESIAN_POINT('Ctrl Pts',(32.8948869928718,-53.2064120173454,-0.6));
#83574=CARTESIAN_POINT('Ctrl Pts',(32.8948869928718,-53.2064120173454,-0.9));
#83575=CARTESIAN_POINT('Ctrl Pts',(32.818345092237,-53.190177500248,-0.6));
#83576=CARTESIAN_POINT('Ctrl Pts',(32.818345092237,-53.190177500248,-0.9));
#83577=CARTESIAN_POINT('Ctrl Pts',(32.6444044336677,-53.190177500248,-0.6));
#83578=CARTESIAN_POINT('Ctrl Pts',(32.6444044336677,-53.190177500248,-0.9));
#83579=CARTESIAN_POINT('',(32.8948869928718,-53.2064120173454,-0.6));
#83580=CARTESIAN_POINT('Ctrl Pts',(32.8948869928718,-53.2064120173454,-0.6));
#83581=CARTESIAN_POINT('Ctrl Pts',(32.818345092237,-53.190177500248,-0.6));
#83582=CARTESIAN_POINT('Ctrl Pts',(32.6444044336677,-53.190177500248,-0.6));
#83583=CARTESIAN_POINT('',(32.8948869928718,-53.2064120173454,-0.9));
#83584=CARTESIAN_POINT('',(32.8948869928718,-53.2064120173454,-0.6));
#83585=CARTESIAN_POINT('Ctrl Pts',(32.8948869928718,-53.2064120173454,-0.9));
#83586=CARTESIAN_POINT('Ctrl Pts',(32.818345092237,-53.190177500248,-0.9));
#83587=CARTESIAN_POINT('Ctrl Pts',(32.6444044336677,-53.190177500248,-0.9));
#83588=CARTESIAN_POINT('Ctrl Pts',(33.1001367792487,-53.2968620657921,-0.6));
#83589=CARTESIAN_POINT('Ctrl Pts',(33.1001367792487,-53.2968620657921,-0.9));
#83590=CARTESIAN_POINT('Ctrl Pts',(32.9992475733161,-53.2319239974022,-0.6));
#83591=CARTESIAN_POINT('Ctrl Pts',(32.9992475733161,-53.2319239974022,-0.9));
#83592=CARTESIAN_POINT('Ctrl Pts',(32.8948869928718,-53.2064120173454,-0.6));
#83593=CARTESIAN_POINT('Ctrl Pts',(32.8948869928718,-53.2064120173454,-0.9));
#83594=CARTESIAN_POINT('',(33.1001367792487,-53.2968620657921,-0.6));
#83595=CARTESIAN_POINT('Ctrl Pts',(33.1001367792487,-53.2968620657921,-0.6));
#83596=CARTESIAN_POINT('Ctrl Pts',(32.9992475733161,-53.2319239974022,-0.6));
#83597=CARTESIAN_POINT('Ctrl Pts',(32.8948869928718,-53.2064120173454,-0.6));
#83598=CARTESIAN_POINT('',(33.1001367792487,-53.2968620657921,-0.9));
#83599=CARTESIAN_POINT('',(33.1001367792487,-53.2968620657921,-0.6));
#83600=CARTESIAN_POINT('Ctrl Pts',(33.1001367792487,-53.2968620657921,-0.9));
#83601=CARTESIAN_POINT('Ctrl Pts',(32.9992475733161,-53.2319239974022,-0.9));
#83602=CARTESIAN_POINT('Ctrl Pts',(32.8948869928718,-53.2064120173454,-0.9));
#83603=CARTESIAN_POINT('Ctrl Pts',(33.3285799250007,-53.5241476893425,-0.6));
#83604=CARTESIAN_POINT('Ctrl Pts',(33.3285799250007,-53.5241476893425,-0.9));
#83605=CARTESIAN_POINT('Ctrl Pts',(33.2010259851813,-53.3618007302284,-0.6));
#83606=CARTESIAN_POINT('Ctrl Pts',(33.2010259851813,-53.3618007302284,-0.9));
#83607=CARTESIAN_POINT('Ctrl Pts',(33.1001367792487,-53.2968620657921,-0.6));
#83608=CARTESIAN_POINT('Ctrl Pts',(33.1001367792487,-53.2968620657921,-0.9));
#83609=CARTESIAN_POINT('',(33.3285799250007,-53.5241476893425,-0.6));
#83610=CARTESIAN_POINT('Ctrl Pts',(33.3285799250007,-53.5241476893425,-0.6));
#83611=CARTESIAN_POINT('Ctrl Pts',(33.2010259851813,-53.3618007302284,-0.6));
#83612=CARTESIAN_POINT('Ctrl Pts',(33.1001367792487,-53.2968620657921,-0.6));
#83613=CARTESIAN_POINT('',(33.3285799250007,-53.5241476893425,-0.9));
#83614=CARTESIAN_POINT('',(33.3285799250007,-53.5241476893425,-0.6));
#83615=CARTESIAN_POINT('Ctrl Pts',(33.3285799250007,-53.5241476893425,-0.9));
#83616=CARTESIAN_POINT('Ctrl Pts',(33.2010259851813,-53.3618007302284,-0.9));
#83617=CARTESIAN_POINT('Ctrl Pts',(33.1001367792487,-53.2968620657921,-0.9));
#83618=CARTESIAN_POINT('Ctrl Pts',(33.6532774195075,-53.9926330447197,-0.6));
#83619=CARTESIAN_POINT('Ctrl Pts',(33.6532774195075,-53.9926330447197,-0.9));
#83620=CARTESIAN_POINT('Ctrl Pts',(33.45613386482,-53.6864940524101,-0.6));
#83621=CARTESIAN_POINT('Ctrl Pts',(33.45613386482,-53.6864940524101,-0.9));
#83622=CARTESIAN_POINT('Ctrl Pts',(33.3285799250007,-53.5241476893425,-0.6));
#83623=CARTESIAN_POINT('Ctrl Pts',(33.3285799250007,-53.5241476893425,-0.9));
#83624=CARTESIAN_POINT('',(33.6532774195075,-53.9926330447197,-0.6));
#83625=CARTESIAN_POINT('Ctrl Pts',(33.6532774195075,-53.9926330447197,-0.6));
#83626=CARTESIAN_POINT('Ctrl Pts',(33.45613386482,-53.6864940524101,-0.6));
#83627=CARTESIAN_POINT('Ctrl Pts',(33.3285799250007,-53.5241476893425,-0.6));
#83628=CARTESIAN_POINT('',(33.6532774195075,-53.9926330447197,-0.9));
#83629=CARTESIAN_POINT('',(33.6532774195075,-53.9926330447197,-0.6));
#83630=CARTESIAN_POINT('Ctrl Pts',(33.6532774195075,-53.9926330447197,-0.9));
#83631=CARTESIAN_POINT('Ctrl Pts',(33.45613386482,-53.6864940524101,-0.9));
#83632=CARTESIAN_POINT('Ctrl Pts',(33.3285799250007,-53.5241476893425,-0.9));
#83633=CARTESIAN_POINT('Origin',(34.1032018885016,-54.7000001072884,-0.6));
#83634=CARTESIAN_POINT('',(34.1032018885016,-54.7000001072884,-0.6));
#83635=CARTESIAN_POINT('',(28.806799412831,-46.3730454302682,-0.6));
#83636=CARTESIAN_POINT('',(34.1032018885016,-54.7000001072884,-0.9));
#83637=CARTESIAN_POINT('',(34.1032018885016,-54.7000001072884,-0.6));
#83638=CARTESIAN_POINT('',(34.1032018885016,-54.7000001072884,-0.9));
#83639=CARTESIAN_POINT('Origin',(34.6691026911139,-54.7000001072884,-0.6));
#83640=CARTESIAN_POINT('',(34.6691026911139,-54.7000001072884,-0.6));
#83641=CARTESIAN_POINT('',(17.334551345557,-54.7000001072884,-0.6));
#83642=CARTESIAN_POINT('',(34.6691026911139,-54.7000001072884,-0.9));
#83643=CARTESIAN_POINT('',(34.6691026911139,-54.7000001072884,-0.6));
#83644=CARTESIAN_POINT('',(34.6691026911139,-54.7000001072884,-0.9));
#83645=CARTESIAN_POINT('Origin',(34.0776911005378,-53.7746248841286,-0.6));
#83646=CARTESIAN_POINT('',(34.0776911005378,-53.7746248841286,-0.6));
#83647=CARTESIAN_POINT('',(28.9606432652394,-45.768036312039,-0.6));
#83648=CARTESIAN_POINT('',(34.0776911005378,-53.7746248841286,-0.9));
#83649=CARTESIAN_POINT('',(34.0776911005378,-53.7746248841286,-0.6));
#83650=CARTESIAN_POINT('',(34.0776911005378,-53.7746248841286,-0.9));
#83651=CARTESIAN_POINT('Ctrl Pts',(33.7042989954352,-53.3223740458488,-0.6));
#83652=CARTESIAN_POINT('Ctrl Pts',(33.7042989954352,-53.3223740458488,-0.9));
#83653=CARTESIAN_POINT('Ctrl Pts',(33.9014330133796,-53.5032741427422,-0.6));
#83654=CARTESIAN_POINT('Ctrl Pts',(33.9014330133796,-53.5032741427422,-0.9));
#83655=CARTESIAN_POINT('Ctrl Pts',(34.0776911005378,-53.7746248841286,-0.6));
#83656=CARTESIAN_POINT('Ctrl Pts',(34.0776911005378,-53.7746248841286,-0.9));
#83657=CARTESIAN_POINT('',(33.7042989954352,-53.3223740458488,-0.6));
#83658=CARTESIAN_POINT('Ctrl Pts',(33.7042989954352,-53.3223740458488,-0.6));
#83659=CARTESIAN_POINT('Ctrl Pts',(33.9014330133796,-53.5032741427422,-0.6));
#83660=CARTESIAN_POINT('Ctrl Pts',(34.0776911005378,-53.7746248841286,-0.6));
#83661=CARTESIAN_POINT('',(33.7042989954352,-53.3223740458488,-0.9));
#83662=CARTESIAN_POINT('',(33.7042989954352,-53.3223740458488,-0.6));
#83663=CARTESIAN_POINT('Ctrl Pts',(33.7042989954352,-53.3223740458488,-0.9));
#83664=CARTESIAN_POINT('Ctrl Pts',(33.9014330133796,-53.5032741427422,-0.9));
#83665=CARTESIAN_POINT('Ctrl Pts',(34.0776911005378,-53.7746248841286,-0.9));
#83666=CARTESIAN_POINT('Ctrl Pts',(33.4329500421882,-53.1530694365501,-0.6));
#83667=CARTESIAN_POINT('Ctrl Pts',(33.4329500421882,-53.1530694365501,-0.9));
#83668=CARTESIAN_POINT('Ctrl Pts',(33.6115255579352,-53.2388810515404,-0.6));
#83669=CARTESIAN_POINT('Ctrl Pts',(33.6115255579352,-53.2388810515404,-0.9));
#83670=CARTESIAN_POINT('Ctrl Pts',(33.7042989954352,-53.3223740458488,-0.6));
#83671=CARTESIAN_POINT('Ctrl Pts',(33.7042989954352,-53.3223740458488,-0.9));
#83672=CARTESIAN_POINT('',(33.4329500421882,-53.1530694365501,-0.6));
#83673=CARTESIAN_POINT('Ctrl Pts',(33.4329500421882,-53.1530694365501,-0.6));
#83674=CARTESIAN_POINT('Ctrl Pts',(33.6115255579352,-53.2388810515404,-0.6));
#83675=CARTESIAN_POINT('Ctrl Pts',(33.7042989954352,-53.3223740458488,-0.6));
#83676=CARTESIAN_POINT('',(33.4329500421882,-53.1530694365501,-0.9));
#83677=CARTESIAN_POINT('',(33.4329500421882,-53.1530694365501,-0.6));
#83678=CARTESIAN_POINT('Ctrl Pts',(33.4329500421882,-53.1530694365501,-0.9));
#83679=CARTESIAN_POINT('Ctrl Pts',(33.6115255579352,-53.2388810515404,-0.9));
#83680=CARTESIAN_POINT('Ctrl Pts',(33.7042989954352,-53.3223740458488,-0.9));
#83681=CARTESIAN_POINT('Ctrl Pts',(34.1565504297614,-52.8376535773277,-0.6));
#83682=CARTESIAN_POINT('Ctrl Pts',(34.1565504297614,-52.8376535773277,-0.9));
#83683=CARTESIAN_POINT('Ctrl Pts',(33.9223089441657,-53.0858115553856,-0.6));
#83684=CARTESIAN_POINT('Ctrl Pts',(33.9223089441657,-53.0858115553856,-0.9));
#83685=CARTESIAN_POINT('Ctrl Pts',(33.4329500421882,-53.1530694365501,-0.6));
#83686=CARTESIAN_POINT('Ctrl Pts',(33.4329500421882,-53.1530694365501,-0.9));
#83687=CARTESIAN_POINT('',(34.1565504297614,-52.8376535773277,-0.6));
#83688=CARTESIAN_POINT('Ctrl Pts',(34.1565504297614,-52.8376535773277,-0.6));
#83689=CARTESIAN_POINT('Ctrl Pts',(33.9223089441657,-53.0858115553856,-0.6));
#83690=CARTESIAN_POINT('Ctrl Pts',(33.4329500421882,-53.1530694365501,-0.6));
#83691=CARTESIAN_POINT('',(34.1565504297614,-52.8376535773277,-0.9));
#83692=CARTESIAN_POINT('',(34.1565504297614,-52.8376535773277,-0.6));
#83693=CARTESIAN_POINT('Ctrl Pts',(34.1565504297614,-52.8376535773277,-0.9));
#83694=CARTESIAN_POINT('Ctrl Pts',(33.9223089441657,-53.0858115553856,-0.9));
#83695=CARTESIAN_POINT('Ctrl Pts',(33.4329500421882,-53.1530694365501,-0.9));
#83696=CARTESIAN_POINT('Ctrl Pts',(34.3907919153571,-52.2276942133904,-0.6));
#83697=CARTESIAN_POINT('Ctrl Pts',(34.3907919153571,-52.2276942133904,-0.9));
#83698=CARTESIAN_POINT('Ctrl Pts',(34.3907919153571,-52.5894955992699,-0.6));
#83699=CARTESIAN_POINT('Ctrl Pts',(34.3907919153571,-52.5894955992699,-0.9));
#83700=CARTESIAN_POINT('Ctrl Pts',(34.1565504297614,-52.8376535773277,-0.6));
#83701=CARTESIAN_POINT('Ctrl Pts',(34.1565504297614,-52.8376535773277,-0.9));
#83702=CARTESIAN_POINT('',(34.3907919153571,-52.2276942133904,-0.6));
#83703=CARTESIAN_POINT('Ctrl Pts',(34.3907919153571,-52.2276942133904,-0.6));
#83704=CARTESIAN_POINT('Ctrl Pts',(34.3907919153571,-52.5894955992699,-0.6));
#83705=CARTESIAN_POINT('Ctrl Pts',(34.1565504297614,-52.8376535773277,-0.6));
#83706=CARTESIAN_POINT('',(34.3907919153571,-52.2276942133904,-0.9));
#83707=CARTESIAN_POINT('',(34.3907919153571,-52.2276942133904,-0.6));
#83708=CARTESIAN_POINT('Ctrl Pts',(34.3907919153571,-52.2276942133904,-0.9));
#83709=CARTESIAN_POINT('Ctrl Pts',(34.3907919153571,-52.5894955992699,-0.9));
#83710=CARTESIAN_POINT('Ctrl Pts',(34.1565504297614,-52.8376535773277,-0.9));
#83711=CARTESIAN_POINT('Ctrl Pts',(34.2493143305182,-51.7151431441307,-0.6));
#83712=CARTESIAN_POINT('Ctrl Pts',(34.2493143305182,-51.7151431441307,-0.9));
#83713=CARTESIAN_POINT('Ctrl Pts',(34.3907919153571,-51.9470672011375,-0.6));
#83714=CARTESIAN_POINT('Ctrl Pts',(34.3907919153571,-51.9470672011375,-0.9));
#83715=CARTESIAN_POINT('Ctrl Pts',(34.3907919153571,-52.2276942133904,-0.6));
#83716=CARTESIAN_POINT('Ctrl Pts',(34.3907919153571,-52.2276942133904,-0.9));
#83717=CARTESIAN_POINT('',(34.2493143305182,-51.7151431441307,-0.6));
#83718=CARTESIAN_POINT('Ctrl Pts',(34.2493143305182,-51.7151431441307,-0.6));
#83719=CARTESIAN_POINT('Ctrl Pts',(34.3907919153571,-51.9470672011375,-0.6));
#83720=CARTESIAN_POINT('Ctrl Pts',(34.3907919153571,-52.2276942133904,-0.6));
#83721=CARTESIAN_POINT('',(34.2493143305182,-51.7151431441307,-0.9));
#83722=CARTESIAN_POINT('',(34.2493143305182,-51.7151431441307,-0.6));
#83723=CARTESIAN_POINT('Ctrl Pts',(34.2493143305182,-51.7151431441307,-0.9));
#83724=CARTESIAN_POINT('Ctrl Pts',(34.3907919153571,-51.9470672011375,-0.9));
#83725=CARTESIAN_POINT('Ctrl Pts',(34.3907919153571,-52.2276942133904,-0.9));
#83726=CARTESIAN_POINT('Ctrl Pts',(33.8712778314948,-51.3916097283363,-0.6));
#83727=CARTESIAN_POINT('Ctrl Pts',(33.8712778314948,-51.3916097283363,-0.9));
#83728=CARTESIAN_POINT('Ctrl Pts',(34.1078462824225,-51.4832196831703,-0.6));
#83729=CARTESIAN_POINT('Ctrl Pts',(34.1078462824225,-51.4832196831703,-0.9));
#83730=CARTESIAN_POINT('Ctrl Pts',(34.2493143305182,-51.7151431441307,-0.6));
#83731=CARTESIAN_POINT('Ctrl Pts',(34.2493143305182,-51.7151431441307,-0.9));
#83732=CARTESIAN_POINT('',(33.8712778314948,-51.3916097283363,-0.6));
#83733=CARTESIAN_POINT('Ctrl Pts',(33.8712778314948,-51.3916097283363,-0.6));
#83734=CARTESIAN_POINT('Ctrl Pts',(34.1078462824225,-51.4832196831703,-0.6));
#83735=CARTESIAN_POINT('Ctrl Pts',(34.2493143305182,-51.7151431441307,-0.6));
#83736=CARTESIAN_POINT('',(33.8712778314948,-51.3916097283363,-0.9));
#83737=CARTESIAN_POINT('',(33.8712778314948,-51.3916097283363,-0.6));
#83738=CARTESIAN_POINT('Ctrl Pts',(33.8712778314948,-51.3916097283363,-0.9));
#83739=CARTESIAN_POINT('Ctrl Pts',(34.1078462824225,-51.4832196831703,-0.9));
#83740=CARTESIAN_POINT('Ctrl Pts',(34.2493143305182,-51.7151431441307,-0.9));
#83741=CARTESIAN_POINT('Ctrl Pts',(33.1801500543952,-51.3000003695488,-0.6));
#83742=CARTESIAN_POINT('Ctrl Pts',(33.1801500543952,-51.3000003695488,-0.9));
#83743=CARTESIAN_POINT('Ctrl Pts',(33.6347189173102,-51.3000003695488,-0.6));
#83744=CARTESIAN_POINT('Ctrl Pts',(33.6347189173102,-51.3000003695488,-0.9));
#83745=CARTESIAN_POINT('Ctrl Pts',(33.8712778314948,-51.3916097283363,-0.6));
#83746=CARTESIAN_POINT('Ctrl Pts',(33.8712778314948,-51.3916097283363,-0.9));
#83747=CARTESIAN_POINT('',(33.1801500543952,-51.3000003695488,-0.6));
#83748=CARTESIAN_POINT('Ctrl Pts',(33.1801500543952,-51.3000003695488,-0.6));
#83749=CARTESIAN_POINT('Ctrl Pts',(33.6347189173102,-51.3000003695488,-0.6));
#83750=CARTESIAN_POINT('Ctrl Pts',(33.8712778314948,-51.3916097283363,-0.6));
#83751=CARTESIAN_POINT('',(33.1801500543952,-51.3000003695488,-0.9));
#83752=CARTESIAN_POINT('',(33.1801500543952,-51.3000003695488,-0.6));
#83753=CARTESIAN_POINT('Ctrl Pts',(33.1801500543952,-51.3000003695488,-0.9));
#83754=CARTESIAN_POINT('Ctrl Pts',(33.6347189173102,-51.3000003695488,-0.9));
#83755=CARTESIAN_POINT('Ctrl Pts',(33.8712778314948,-51.3916097283363,-0.9));
#83756=CARTESIAN_POINT('Origin',(31.6726484522223,-51.3000003695488,-0.6));
#83757=CARTESIAN_POINT('',(31.6726484522223,-51.3000003695488,-0.6));
#83758=CARTESIAN_POINT('',(15.8363242261112,-51.3000003695488,-0.6));
#83759=CARTESIAN_POINT('',(31.6726484522223,-51.3000003695488,-0.9));
#83760=CARTESIAN_POINT('',(31.6726484522223,-51.3000003695488,-0.6));
#83761=CARTESIAN_POINT('',(31.6726484522223,-51.3000003695488,-0.9));
#83762=CARTESIAN_POINT('Origin',(31.6726484522223,-54.7000001072884,-0.6));
#83763=CARTESIAN_POINT('',(31.6726484522223,-54.7000001072884,-0.6));
#83764=CARTESIAN_POINT('',(31.6726484522223,-53.8500000536442,-0.6));
#83765=CARTESIAN_POINT('',(31.6726484522223,-54.7000001072884,-0.9));
#83766=CARTESIAN_POINT('',(31.6726484522223,-54.7000001072884,-0.6));
#83767=CARTESIAN_POINT('',(31.6726484522223,-54.7000001072884,-0.9));
#83768=CARTESIAN_POINT('Origin',(32.1225824579597,-54.7000001072884,-0.6));
#83769=CARTESIAN_POINT('',(32.1225824579597,-54.7000001072884,-0.6));
#83770=CARTESIAN_POINT('',(16.0612912289798,-54.7000001072884,-0.6));
#83771=CARTESIAN_POINT('',(32.1225824579597,-54.7000001072884,-0.9));
#83772=CARTESIAN_POINT('',(32.1225824579597,-54.7000001072884,-0.6));
#83773=CARTESIAN_POINT('',(32.1225824579597,-54.7000001072884,-0.9));
#83774=CARTESIAN_POINT('Origin',(32.1225824579597,-53.190177500248,-0.6));
#83775=CARTESIAN_POINT('',(32.1225824579597,-53.095088750124,-0.6));
#83776=CARTESIAN_POINT('',(32.1225824579597,-53.190177500248,-0.9));
#83777=CARTESIAN_POINT('Origin',(33.1708755716681,-53.0000002384186,-0.9));
#83778=CARTESIAN_POINT('Origin',(-36.,-60.,-0.6));
#83779=CARTESIAN_POINT('',(36.,-60.,0.));
#83780=CARTESIAN_POINT('',(-36.,-60.,0.));
#83781=CARTESIAN_POINT('',(-18.,-60.,0.));
#83782=CARTESIAN_POINT('',(36.,-60.,-0.6));
#83783=CARTESIAN_POINT('',(36.,-60.,-0.6));
#83784=CARTESIAN_POINT('',(-36.,-60.,-0.6));
#83785=CARTESIAN_POINT('',(-36.,-60.,-0.6));
#83786=CARTESIAN_POINT('',(-36.,-60.,-0.6));
#83787=CARTESIAN_POINT('Origin',(-36.,-46.,-0.6));
#83788=CARTESIAN_POINT('',(-36.,-46.,0.));
#83789=CARTESIAN_POINT('',(-36.,-23.,0.));
#83790=CARTESIAN_POINT('',(-36.,-46.,-0.6));
#83791=CARTESIAN_POINT('',(-36.,-46.,-0.6));
#83792=CARTESIAN_POINT('',(-36.,-46.,-0.6));
#83793=CARTESIAN_POINT('Origin',(36.,-46.,-0.6));
#83794=CARTESIAN_POINT('',(36.,-46.,0.));
#83795=CARTESIAN_POINT('',(18.,-46.,0.));
#83796=CARTESIAN_POINT('',(36.,-46.,-0.6));
#83797=CARTESIAN_POINT('',(36.,-46.,-0.6));
#83798=CARTESIAN_POINT('',(36.,-46.,-0.6));
#83799=CARTESIAN_POINT('Origin',(36.,-60.,-0.6));
#83800=CARTESIAN_POINT('',(36.,-30.,0.));
#83801=CARTESIAN_POINT('',(36.,-60.,-0.6));
#83802=CARTESIAN_POINT('Origin',(0.,-53.,-0.6));
#83803=CARTESIAN_POINT('Origin',(-75.,-50.,-0.25));
#83804=CARTESIAN_POINT('',(-80.,-50.,0.));
#83805=CARTESIAN_POINT('Origin',(-75.,-50.,0.));
#83806=CARTESIAN_POINT('',(-79.5,-50.,-0.5));
#83807=CARTESIAN_POINT('',(-79.75,-50.,-0.25));
#83808=CARTESIAN_POINT('Origin',(-75.,-50.,-0.5));
#83809=CARTESIAN_POINT('Origin',(-75.,-50.,-16.5));
#83810=CARTESIAN_POINT('',(-79.5,-50.,-15.5));
#83811=CARTESIAN_POINT('Origin',(-75.,-50.,-15.5));
#83812=CARTESIAN_POINT('',(-79.5,-50.,-16.5));
#83813=CARTESIAN_POINT('Origin',(0.,0.,0.));
#83814=CARTESIAN_POINT('',(-89.,-55.,0.));
#83815=CARTESIAN_POINT('',(-89.,55.,0.));
#83816=CARTESIAN_POINT('',(-89.,27.5,0.));
#83817=CARTESIAN_POINT('',(-80.,-64.,0.));
#83818=CARTESIAN_POINT('Origin',(-80.,-55.,0.));
#83819=CARTESIAN_POINT('',(80.,-64.,0.));
#83820=CARTESIAN_POINT('',(-40.,-64.,0.));
#83821=CARTESIAN_POINT('',(89.,-55.,0.));
#83822=CARTESIAN_POINT('Origin',(80.,-55.,0.));
#83823=CARTESIAN_POINT('',(89.,55.,0.));
#83824=CARTESIAN_POINT('',(89.,-27.5,0.));
#83825=CARTESIAN_POINT('',(80.,64.,0.));
#83826=CARTESIAN_POINT('Origin',(80.,55.,0.));
#83827=CARTESIAN_POINT('',(-80.,64.,0.));
#83828=CARTESIAN_POINT('',(40.,64.,0.));
#83829=CARTESIAN_POINT('Origin',(-80.,55.,0.));
#83830=CARTESIAN_POINT('',(70.,-50.,0.));
#83831=CARTESIAN_POINT('Origin',(75.,-50.,0.));
#83832=CARTESIAN_POINT('',(-38.3,4.69039724073436E-15,8.15320033709099E-16));
#83833=CARTESIAN_POINT('Origin',(-35.,4.28626379701574E-15,0.));
#83834=CARTESIAN_POINT('',(31.7,4.04133443718627E-16,8.15320033709099E-16));
#83835=CARTESIAN_POINT('Origin',(35.,0.,0.));
#83836=CARTESIAN_POINT('',(-3.3,35.,8.15320033709099E-16));
#83837=CARTESIAN_POINT('Origin',(2.14313189850787E-15,35.,0.));
#83838=CARTESIAN_POINT('',(-3.30000000000001,-35.,8.15320033709099E-16));
#83839=CARTESIAN_POINT('Origin',(-6.4293956955236E-15,-35.,0.));
#83840=CARTESIAN_POINT('',(-20.025,2.45235521529257E-15,0.));
#83841=CARTESIAN_POINT('Origin',(0.,0.,0.));
#83842=CARTESIAN_POINT('',(-27.7487373415292,-24.7487373415292,0.));
#83843=CARTESIAN_POINT('Origin',(-24.7487373415292,-24.7487373415292,0.));
#83844=CARTESIAN_POINT('',(21.7487373415292,24.7487373415292,0.));
#83845=CARTESIAN_POINT('Origin',(24.7487373415292,24.7487373415292,0.));
#83846=CARTESIAN_POINT('',(-80.,50.,0.));
#83847=CARTESIAN_POINT('Origin',(-75.,50.,0.));
#83848=CARTESIAN_POINT('',(70.,50.,0.));
#83849=CARTESIAN_POINT('Origin',(75.,50.,0.));
#83850=CARTESIAN_POINT('Origin',(-75.,-50.,-15.75));
#83851=CARTESIAN_POINT('',(-80.,-50.,-16.));
#83852=CARTESIAN_POINT('Origin',(-75.,-50.,-16.));
#83853=CARTESIAN_POINT('',(-79.75,-50.,-15.75));
#83854=CARTESIAN_POINT('Origin',(0.,0.,-16.));
#83855=CARTESIAN_POINT('',(80.,-64.5,-16.));
#83856=CARTESIAN_POINT('',(89.5,-55.,-16.));
#83857=CARTESIAN_POINT('Origin',(80.,-55.,-16.));
#83858=CARTESIAN_POINT('',(-80.,-64.5,-16.));
#83859=CARTESIAN_POINT('',(-40.,-64.5,-16.));
#83860=CARTESIAN_POINT('',(-89.5,-55.,-16.));
#83861=CARTESIAN_POINT('Origin',(-80.,-55.,-16.));
#83862=CARTESIAN_POINT('',(-89.5,55.,-16.));
#83863=CARTESIAN_POINT('',(-89.5,27.5,-16.));
#83864=CARTESIAN_POINT('',(-80.,64.5,-16.));
#83865=CARTESIAN_POINT('Origin',(-80.,55.,-16.));
#83866=CARTESIAN_POINT('',(80.,64.5,-16.));
#83867=CARTESIAN_POINT('',(40.,64.5,-16.));
#83868=CARTESIAN_POINT('',(89.5,55.,-16.));
#83869=CARTESIAN_POINT('Origin',(80.,55.,-16.));
#83870=CARTESIAN_POINT('',(89.5,-27.5,-16.));
#83871=CARTESIAN_POINT('',(70.,50.,-16.));
#83872=CARTESIAN_POINT('Origin',(75.,50.,-16.));
#83873=CARTESIAN_POINT('',(-80.,50.,-16.));
#83874=CARTESIAN_POINT('Origin',(-75.,50.,-16.));
#83875=CARTESIAN_POINT('',(70.,-50.,-16.));
#83876=CARTESIAN_POINT('Origin',(75.,-50.,-16.));
#83877=CARTESIAN_POINT('Origin',(75.,50.,-0.25));
#83878=CARTESIAN_POINT('',(70.5,50.,-0.5));
#83879=CARTESIAN_POINT('',(70.25,50.,-0.25));
#83880=CARTESIAN_POINT('Origin',(75.,50.,-0.5));
#83881=CARTESIAN_POINT('Origin',(75.,50.,-16.5));
#83882=CARTESIAN_POINT('',(70.5,50.,-15.5));
#83883=CARTESIAN_POINT('Origin',(75.,50.,-15.5));
#83884=CARTESIAN_POINT('',(70.5,50.,-16.5));
#83885=CARTESIAN_POINT('Origin',(75.,50.,-15.75));
#83886=CARTESIAN_POINT('',(70.25,50.,-15.75));
#83887=CARTESIAN_POINT('Origin',(75.,-50.,-0.25));
#83888=CARTESIAN_POINT('',(70.5,-50.,-0.5));
#83889=CARTESIAN_POINT('',(70.25,-50.,-0.25));
#83890=CARTESIAN_POINT('Origin',(75.,-50.,-0.5));
#83891=CARTESIAN_POINT('Origin',(75.,-50.,-16.5));
#83892=CARTESIAN_POINT('',(70.5,-50.,-15.5));
#83893=CARTESIAN_POINT('Origin',(75.,-50.,-15.5));
#83894=CARTESIAN_POINT('',(70.5,-50.,-16.5));
#83895=CARTESIAN_POINT('Origin',(75.,-50.,-15.75));
#83896=CARTESIAN_POINT('',(70.25,-50.,-15.75));
#83897=CARTESIAN_POINT('Origin',(-75.,50.,-0.25));
#83898=CARTESIAN_POINT('',(-79.5,50.,-0.5));
#83899=CARTESIAN_POINT('',(-79.75,50.,-0.25));
#83900=CARTESIAN_POINT('Origin',(-75.,50.,-0.5));
#83901=CARTESIAN_POINT('Origin',(-75.,50.,-16.5));
#83902=CARTESIAN_POINT('',(-79.5,50.,-15.5));
#83903=CARTESIAN_POINT('Origin',(-75.,50.,-15.5));
#83904=CARTESIAN_POINT('',(-79.5,50.,-16.5));
#83905=CARTESIAN_POINT('Origin',(-75.,50.,-15.75));
#83906=CARTESIAN_POINT('',(-79.75,50.,-15.75));
#83907=CARTESIAN_POINT('Origin',(24.7487373415292,24.7487373415292,-10.9012909285413));
#83908=CARTESIAN_POINT('',(21.7487373415292,24.7487373415292,-10.));
#83909=CARTESIAN_POINT('Origin',(24.7487373415292,24.7487373415292,-10.));
#83910=CARTESIAN_POINT('',(24.7487373415292,24.7487373415292,-11.8025818570827));
#83911=CARTESIAN_POINT('',(23.2487373415292,24.7487373415292,-10.9012909285413));
#83912=CARTESIAN_POINT('Origin',(24.7487373415292,24.7487373415292,-5.));
#83913=CARTESIAN_POINT('',(21.7487373415292,24.7487373415292,-5.));
#83914=CARTESIAN_POINT('Origin',(-24.7487373415292,-24.7487373415292,-10.9012909285413));
#83915=CARTESIAN_POINT('',(-27.7487373415292,-24.7487373415292,-10.));
#83916=CARTESIAN_POINT('Origin',(-24.7487373415292,-24.7487373415292,-10.));
#83917=CARTESIAN_POINT('',(-24.7487373415292,-24.7487373415292,-11.8025818570827));
#83918=CARTESIAN_POINT('',(-26.2487373415292,-24.7487373415292,-10.9012909285413));
#83919=CARTESIAN_POINT('Origin',(-24.7487373415292,-24.7487373415292,-5.));
#83920=CARTESIAN_POINT('',(-27.7487373415292,-24.7487373415292,-5.));
#83921=CARTESIAN_POINT('Origin',(-35.,4.28626379701574E-15,-14.916312444017));
#83922=CARTESIAN_POINT('',(-38.05,4.65978107075568E-15,-14.));
#83923=CARTESIAN_POINT('Origin',(-35.,4.28626379701574E-15,-14.));
#83924=CARTESIAN_POINT('',(-35.,4.28626379701574E-15,-15.8326248880341));
#83925=CARTESIAN_POINT('',(-36.525,4.47302243388571E-15,-14.916312444017));
#83926=CARTESIAN_POINT('Origin',(-35.,4.28626379701574E-15,-0.125));
#83927=CARTESIAN_POINT('',(-38.05,4.65978107075568E-15,-0.250000000000001));
#83928=CARTESIAN_POINT('',(-38.175,4.67508915574502E-15,-0.125));
#83929=CARTESIAN_POINT('Origin',(-35.,4.28626379701574E-15,-0.250000000000001));
#83930=CARTESIAN_POINT('Origin',(-35.,4.28626379701574E-15,-7.));
#83931=CARTESIAN_POINT('',(-38.05,4.65978107075568E-15,-7.));
#83932=CARTESIAN_POINT('Origin',(35.,0.,-14.916312444017));
#83933=CARTESIAN_POINT('',(31.95,3.73517273739943E-16,-14.));
#83934=CARTESIAN_POINT('Origin',(35.,0.,-14.));
#83935=CARTESIAN_POINT('',(35.,0.,-15.8326248880341));
#83936=CARTESIAN_POINT('',(33.475,1.86758636869971E-16,-14.916312444017));
#83937=CARTESIAN_POINT('Origin',(35.,0.,-0.125));
#83938=CARTESIAN_POINT('',(31.95,3.73517273739943E-16,-0.250000000000001));
#83939=CARTESIAN_POINT('',(31.825,3.88825358729285E-16,-0.125));
#83940=CARTESIAN_POINT('Origin',(35.,0.,-0.250000000000001));
#83941=CARTESIAN_POINT('Origin',(35.,0.,-7.));
#83942=CARTESIAN_POINT('',(31.95,3.73517273739943E-16,-7.));
#83943=CARTESIAN_POINT('Origin',(2.14313189850787E-15,35.,-14.916312444017));
#83944=CARTESIAN_POINT('',(-3.05,35.,-14.));
#83945=CARTESIAN_POINT('Origin',(2.14313189850787E-15,35.,-14.));
#83946=CARTESIAN_POINT('',(2.14313189850787E-15,35.,-15.8326248880341));
#83947=CARTESIAN_POINT('',(-1.525,35.,-14.916312444017));
#83948=CARTESIAN_POINT('Origin',(2.14313189850787E-15,35.,-0.125));
#83949=CARTESIAN_POINT('',(-3.05,35.,-0.250000000000001));
#83950=CARTESIAN_POINT('',(-3.175,35.,-0.125));
#83951=CARTESIAN_POINT('Origin',(2.14313189850787E-15,35.,-0.250000000000001));
#83952=CARTESIAN_POINT('Origin',(2.14313189850787E-15,35.,-7.));
#83953=CARTESIAN_POINT('',(-3.05,35.,-7.));
#83954=CARTESIAN_POINT('Origin',(-6.4293956955236E-15,-35.,-14.916312444017));
#83955=CARTESIAN_POINT('',(-3.05000000000001,-35.,-14.));
#83956=CARTESIAN_POINT('Origin',(-6.4293956955236E-15,-35.,-14.));
#83957=CARTESIAN_POINT('',(-6.4293956955236E-15,-35.,-15.8326248880341));
#83958=CARTESIAN_POINT('',(-1.52500000000001,-35.,-14.916312444017));
#83959=CARTESIAN_POINT('Origin',(-6.4293956955236E-15,-35.,-0.125));
#83960=CARTESIAN_POINT('',(-3.05000000000001,-35.,-0.250000000000001));
#83961=CARTESIAN_POINT('',(-3.17500000000001,-35.,-0.125));
#83962=CARTESIAN_POINT('Origin',(-6.4293956955236E-15,-35.,-0.250000000000001));
#83963=CARTESIAN_POINT('Origin',(-6.4293956955236E-15,-35.,-7.));
#83964=CARTESIAN_POINT('',(-3.05000000000001,-35.,-7.));
#83965=CARTESIAN_POINT('Origin',(0.,0.,-4.2));
#83966=CARTESIAN_POINT('',(-20.025,-2.45235521529257E-15,-4.2));
#83967=CARTESIAN_POINT('Origin',(0.,0.,-4.2));
#83968=CARTESIAN_POINT('',(-20.025,-2.45235521529257E-15,-4.2));
#83969=CARTESIAN_POINT('Origin',(0.,0.,-4.2));
#83970=CARTESIAN_POINT('Origin',(80.,-55.,-15.75));
#83971=CARTESIAN_POINT('',(90.,-55.,-15.5));
#83972=CARTESIAN_POINT('',(89.5,-55.,-16.));
#83973=CARTESIAN_POINT('',(80.,-65.,-15.5));
#83974=CARTESIAN_POINT('Origin',(80.,-55.,-15.5));
#83975=CARTESIAN_POINT('',(80.,-65.,-15.5));
#83976=CARTESIAN_POINT('Origin',(89.75,-27.5,-15.75));
#83977=CARTESIAN_POINT('',(90.,55.,-15.5));
#83978=CARTESIAN_POINT('',(89.5,55.,-16.));
#83979=CARTESIAN_POINT('',(90.,-27.5,-15.5));
#83980=CARTESIAN_POINT('Origin',(80.,55.,-15.75));
#83981=CARTESIAN_POINT('',(80.,65.,-15.5));
#83982=CARTESIAN_POINT('',(80.,64.5,-16.));
#83983=CARTESIAN_POINT('Origin',(80.,55.,-15.5));
#83984=CARTESIAN_POINT('Origin',(40.,64.75,-15.75));
#83985=CARTESIAN_POINT('',(-80.,65.,-15.5));
#83986=CARTESIAN_POINT('',(-80.,64.5,-16.));
#83987=CARTESIAN_POINT('',(40.,65.,-15.5));
#83988=CARTESIAN_POINT('Origin',(-80.,55.,-15.75));
#83989=CARTESIAN_POINT('',(-90.,55.,-15.5));
#83990=CARTESIAN_POINT('',(-89.5,55.,-16.));
#83991=CARTESIAN_POINT('Origin',(-80.,55.,-15.5));
#83992=CARTESIAN_POINT('Origin',(-89.75,27.5,-15.75));
#83993=CARTESIAN_POINT('',(-90.,-55.,-15.5));
#83994=CARTESIAN_POINT('',(-89.5,-55.,-16.));
#83995=CARTESIAN_POINT('',(-90.,27.5,-15.5));
#83996=CARTESIAN_POINT('Origin',(-80.,-55.,-15.75));
#83997=CARTESIAN_POINT('',(-80.,-65.,-15.5));
#83998=CARTESIAN_POINT('',(-80.,-64.5,-16.));
#83999=CARTESIAN_POINT('Origin',(-80.,-55.,-15.5));
#84000=CARTESIAN_POINT('Origin',(-40.,-64.75,-15.75));
#84001=CARTESIAN_POINT('',(-40.,-65.,-15.5));
#84002=CARTESIAN_POINT('Origin',(-90.,55.,-16.));
#84003=CARTESIAN_POINT('',(-90.,-55.,-1.));
#84004=CARTESIAN_POINT('',(-90.,-55.,-16.));
#84005=CARTESIAN_POINT('',(-90.,55.,-1.));
#84006=CARTESIAN_POINT('',(-90.,27.5,-1.));
#84007=CARTESIAN_POINT('',(-90.,55.,-16.));
#84008=CARTESIAN_POINT('Origin',(-80.,-55.,-16.));
#84009=CARTESIAN_POINT('',(-80.,-65.,-1.));
#84010=CARTESIAN_POINT('',(-80.,-65.,-16.));
#84011=CARTESIAN_POINT('Origin',(-80.,-55.,-1.));
#84012=CARTESIAN_POINT('Origin',(-80.,-65.,-16.));
#84013=CARTESIAN_POINT('',(80.,-65.,-1.));
#84014=CARTESIAN_POINT('',(80.,-65.,-16.));
#84015=CARTESIAN_POINT('',(-40.,-65.,-1.));
#84016=CARTESIAN_POINT('Origin',(80.,-55.,-16.));
#84017=CARTESIAN_POINT('',(90.,-55.,-1.));
#84018=CARTESIAN_POINT('',(90.,-55.,-16.));
#84019=CARTESIAN_POINT('Origin',(80.,-55.,-1.));
#84020=CARTESIAN_POINT('Origin',(-89.5,27.5,-0.5));
#84021=CARTESIAN_POINT('',(-90.,-55.,-1.));
#84022=CARTESIAN_POINT('',(-89.,55.,0.));
#84023=CARTESIAN_POINT('Origin',(-80.,-55.,-0.5));
#84024=CARTESIAN_POINT('',(-80.,-65.,-1.));
#84025=CARTESIAN_POINT('Origin',(-40.,-64.5,-0.5));
#84026=CARTESIAN_POINT('',(80.,-65.,-1.));
#84027=CARTESIAN_POINT('Origin',(80.,-55.,-0.5));
#84028=CARTESIAN_POINT('',(90.,-55.,-1.));
#84029=CARTESIAN_POINT('Origin',(89.5,-27.5,-0.5));
#84030=CARTESIAN_POINT('',(90.,55.,-1.));
#84031=CARTESIAN_POINT('',(90.,55.,-1.));
#84032=CARTESIAN_POINT('',(90.,-27.5,-1.));
#84033=CARTESIAN_POINT('Origin',(80.,55.,-0.5));
#84034=CARTESIAN_POINT('',(80.,65.,-1.));
#84035=CARTESIAN_POINT('',(80.,65.,-1.));
#84036=CARTESIAN_POINT('Origin',(80.,55.,-1.));
#84037=CARTESIAN_POINT('Origin',(40.,64.5,-0.5));
#84038=CARTESIAN_POINT('',(-80.,65.,-1.));
#84039=CARTESIAN_POINT('',(-80.,65.,-1.));
#84040=CARTESIAN_POINT('',(40.,65.,-1.));
#84041=CARTESIAN_POINT('Origin',(-80.,55.,-0.5));
#84042=CARTESIAN_POINT('Origin',(-80.,55.,-1.));
#84043=CARTESIAN_POINT('Origin',(-80.,55.,-16.));
#84044=CARTESIAN_POINT('',(-80.,65.,-16.));
#84045=CARTESIAN_POINT('Origin',(80.,65.,-16.));
#84046=CARTESIAN_POINT('',(80.,65.,-16.));
#84047=CARTESIAN_POINT('Origin',(80.,55.,-16.));
#84048=CARTESIAN_POINT('',(90.,55.,-16.));
#84049=CARTESIAN_POINT('Origin',(90.,-55.,-16.));
#94274=UNCERTAINTY_MEASURE_WITH_UNIT(LENGTH_MEASURE(0.01),#94302,
'DISTANCE_ACCURACY_VALUE',
'Maximum model space distance between geometric entities at asserted c
onnectivities');
#94285=UNCERTAINTY_MEASURE_WITH_UNIT(LENGTH_MEASURE(0.01),#94302,
'DISTANCE_ACCURACY_VALUE',
'Maximum model space distance between geometric entities at asserted c
onnectivities');
#94290=(
GEOMETRIC_REPRESENTATION_CONTEXT(3)
GLOBAL_UNCERTAINTY_ASSIGNED_CONTEXT((#94274))
GLOBAL_UNIT_ASSIGNED_CONTEXT((#94302,#94304,#94305))
REPRESENTATION_CONTEXT('','3D')
);
#94301=(
GEOMETRIC_REPRESENTATION_CONTEXT(3)
GLOBAL_UNCERTAINTY_ASSIGNED_CONTEXT((#94285))
GLOBAL_UNIT_ASSIGNED_CONTEXT((#94302,#94304,#94305))
REPRESENTATION_CONTEXT('','3D')
);
#94302=(
LENGTH_UNIT()
NAMED_UNIT(*)
SI_UNIT(.MILLI.,.METRE.)
);
#94304=(
NAMED_UNIT(*)
PLANE_ANGLE_UNIT()
SI_UNIT($,.RADIAN.)
);
#94305=(
NAMED_UNIT(*)
SI_UNIT($,.STERADIAN.)
SOLID_ANGLE_UNIT()
);
#94310=SHAPE_DEFINITION_REPRESENTATION(#94325,#94374);
#94325=PRODUCT_DEFINITION_SHAPE('',$,#94390);
#94374=SHAPE_REPRESENTATION('',(#54216),#94290);
#94385=PRODUCT_DEFINITION_CONTEXT('part definition',#94432,'design');
#94390=PRODUCT_DEFINITION('2026-10-11-08-26-34-988',
'04_Base_Plate_180x130x16',#94405,#94385);
#94405=PRODUCT_DEFINITION_FORMATION('',$,#94438);
#94432=APPLICATION_CONTEXT(
'Core Data for Automotive Mechanical Design Process');
#94433=PRODUCT_CONTEXT('part definition',#94432,'mechanical');
#94438=PRODUCT('2026-10-11-08-26-34-988','04_Base_Plate_180x130x16',$,(#94433));
#94554=COLOUR_RGB('Dark Blue',0.08,0.2,0.34);
#94555=FILL_AREA_STYLE_COLOUR('',#94554);
#94556=FILL_AREA_STYLE('',(#94555));
#94557=SURFACE_STYLE_FILL_AREA(#94556);
#94558=SURFACE_SIDE_STYLE('',(#94557));
#94559=SURFACE_STYLE_USAGE(.BOTH.,#94558);
#94560=PRESENTATION_STYLE_ASSIGNMENT((#94559));
ENDSEC;
END-ISO-10303-21;
